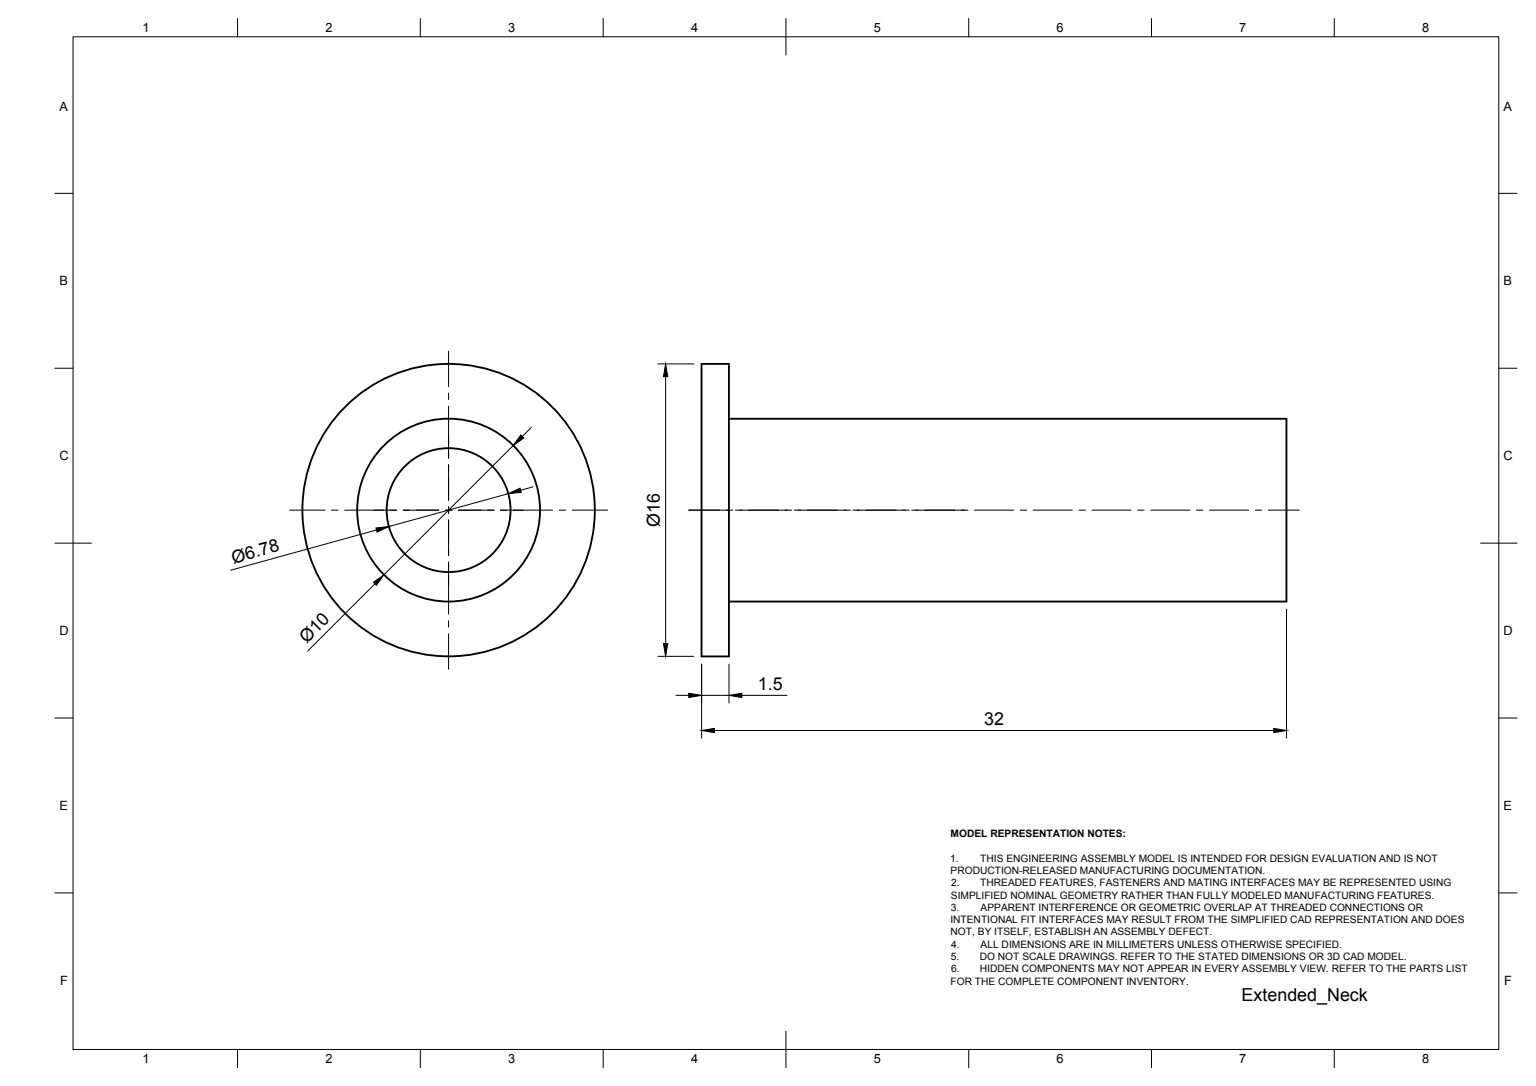
ISO-10303-21;
HEADER;
/* Generated by software containing ST-Developer
 * from STEP Tools, Inc. (www.steptools.com) 
 */

FILE_DESCRIPTION(
/* description */ (''),
/* implementation_level */ '2;1');

FILE_NAME(
/* name */ 'Extended_Neck.step',
/* time_stamp */ '2026-10-06T12:52:28-07:00',
/* author */ (''),
/* organization */ (''),
/* preprocessor_version */ 'ST-DEVELOPER v20.2',
/* originating_system */ 'Autodesk Translation Framework v15.15.0.0',
/* authorisation */ '');

FILE_SCHEMA (('AUTOMOTIVE_DESIGN { 1 0 10303 214 3 1 1 }'));
ENDSEC;

DATA;
#10=MECHANICAL_DESIGN_GEOMETRIC_PRESENTATION_REPRESENTATION('',(#76),#34403);
#45=B_SPLINE_SURFACE_WITH_KNOTS('',3,3,((#12810,#12811,#12812,#12813,#12814,
#12815,#12816,#12817,#12818,#12819,#12820,#12821,#12822,#12823,#12824,#12825,
#12826,#12827,#12828,#12829,#12830,#12831,#12832,#12833,#12834,#12835,#12836,
#12837,#12838,#12839,#12840,#12841,#12842,#12843,#12844,#12845,#12846,#12847,
#12848,#12849,#12850,#12851,#12852,#12853,#12854,#12855,#12856,#12857,#12858,
#12859,#12860,#12861,#12862,#12863,#12864,#12865),(#12866,#12867,#12868,
#12869,#12870,#12871,#12872,#12873,#12874,#12875,#12876,#12877,#12878,#12879,
#12880,#12881,#12882,#12883,#12884,#12885,#12886,#12887,#12888,#12889,#12890,
#12891,#12892,#12893,#12894,#12895,#12896,#12897,#12898,#12899,#12900,#12901,
#12902,#12903,#12904,#12905,#12906,#12907,#12908,#12909,#12910,#12911,#12912,
#12913,#12914,#12915,#12916,#12917,#12918,#12919,#12920,#12921),(#12922,
#12923,#12924,#12925,#12926,#12927,#12928,#12929,#12930,#12931,#12932,#12933,
#12934,#12935,#12936,#12937,#12938,#12939,#12940,#12941,#12942,#12943,#12944,
#12945,#12946,#12947,#12948,#12949,#12950,#12951,#12952,#12953,#12954,#12955,
#12956,#12957,#12958,#12959,#12960,#12961,#12962,#12963,#12964,#12965,#12966,
#12967,#12968,#12969,#12970,#12971,#12972,#12973,#12974,#12975,#12976,#12977),
(#12978,#12979,#12980,#12981,#12982,#12983,#12984,#12985,#12986,#12987,
#12988,#12989,#12990,#12991,#12992,#12993,#12994,#12995,#12996,#12997,#12998,
#12999,#13000,#13001,#13002,#13003,#13004,#13005,#13006,#13007,#13008,#13009,
#13010,#13011,#13012,#13013,#13014,#13015,#13016,#13017,#13018,#13019,#13020,
#13021,#13022,#13023,#13024,#13025,#13026,#13027,#13028,#13029,#13030,#13031,
#13032,#13033)),.UNSPECIFIED.,.F.,.F.,.F.,(4,4),(4,1,1,1,1,1,1,1,1,1,1,
1,1,1,1,1,1,1,1,1,1,1,1,1,1,1,1,1,1,1,1,1,1,1,1,1,1,1,1,1,1,1,1,1,1,1,1,
1,1,1,1,1,1,4),(-0.00052867975577478,0.0806738746488675),(15.627449007124,
16.6139235895809,17.6003981720377,18.5868727544945,19.5733473369513,20.5598219194081,
21.5462965018649,22.5327710843217,23.5192456667785,24.5057202492353,25.4921948316921,
26.4786694141489,27.4651439966058,28.4516185790626,29.4380931615194,30.4245677439762,
31.411042326433,32.3975169088898,33.3839914913466,34.3704660738034,35.3569406562602,
36.343415238717,37.3298898211739,38.3163644036307,39.3028389860875,40.2893135685443,
41.2757881510011,42.2622627334579,43.2487373159147,44.2352118983715,45.2216864808283,
46.2081610632851,47.1946356457419,48.1811102281988,49.1675848106556,50.1540593931124,
51.1405339755692,52.127008558026,53.1134831404828,54.0999577229396,55.0864323053964,
56.0729068878532,57.05938147031,58.0458560527669,59.0323306352237,60.0188052176805,
61.0052798001373,61.9917543825941,62.9782289650509,63.9647035475077,64.9511781299645,
65.9376527124213,66.9241272948781,67.9106018773349),.UNSPECIFIED.);
#46=B_SPLINE_SURFACE_WITH_KNOTS('',3,3,((#13314,#13315,#13316,#13317,#13318,
#13319,#13320,#13321,#13322,#13323,#13324,#13325,#13326,#13327,#13328,#13329,
#13330,#13331,#13332,#13333,#13334,#13335,#13336,#13337,#13338,#13339,#13340,
#13341,#13342,#13343,#13344,#13345,#13346,#13347,#13348,#13349,#13350,#13351,
#13352,#13353,#13354,#13355,#13356,#13357,#13358,#13359,#13360,#13361,#13362,
#13363,#13364,#13365,#13366,#13367,#13368,#13369),(#13370,#13371,#13372,
#13373,#13374,#13375,#13376,#13377,#13378,#13379,#13380,#13381,#13382,#13383,
#13384,#13385,#13386,#13387,#13388,#13389,#13390,#13391,#13392,#13393,#13394,
#13395,#13396,#13397,#13398,#13399,#13400,#13401,#13402,#13403,#13404,#13405,
#13406,#13407,#13408,#13409,#13410,#13411,#13412,#13413,#13414,#13415,#13416,
#13417,#13418,#13419,#13420,#13421,#13422,#13423,#13424,#13425),(#13426,
#13427,#13428,#13429,#13430,#13431,#13432,#13433,#13434,#13435,#13436,#13437,
#13438,#13439,#13440,#13441,#13442,#13443,#13444,#13445,#13446,#13447,#13448,
#13449,#13450,#13451,#13452,#13453,#13454,#13455,#13456,#13457,#13458,#13459,
#13460,#13461,#13462,#13463,#13464,#13465,#13466,#13467,#13468,#13469,#13470,
#13471,#13472,#13473,#13474,#13475,#13476,#13477,#13478,#13479,#13480,#13481),
(#13482,#13483,#13484,#13485,#13486,#13487,#13488,#13489,#13490,#13491,
#13492,#13493,#13494,#13495,#13496,#13497,#13498,#13499,#13500,#13501,#13502,
#13503,#13504,#13505,#13506,#13507,#13508,#13509,#13510,#13511,#13512,#13513,
#13514,#13515,#13516,#13517,#13518,#13519,#13520,#13521,#13522,#13523,#13524,
#13525,#13526,#13527,#13528,#13529,#13530,#13531,#13532,#13533,#13534,#13535,
#13536,#13537)),.UNSPECIFIED.,.F.,.F.,.F.,(4,4),(4,1,1,1,1,1,1,1,1,1,1,
1,1,1,1,1,1,1,1,1,1,1,1,1,1,1,1,1,1,1,1,1,1,1,1,1,1,1,1,1,1,1,1,1,1,1,1,
1,1,1,1,1,1,4),(-0.000393360025247636,0.0809589398657946),(18.1690368310252,
19.155511413482,20.1419859959388,21.1284605783956,22.1149351608524,23.1014097433092,
24.087884325766,25.0743589082228,26.0608334906796,27.0473080731364,28.0337826555933,
29.0202572380501,30.0067318205069,30.9932064029637,31.9796809854205,32.9661555678773,
33.9526301503341,34.9391047327909,35.9255793152477,36.9120538977045,37.8985284801614,
38.8850030626182,39.871477645075,40.8579522275318,41.8444268099886,42.8309013924454,
43.8173759749022,44.803850557359,45.7903251398158,46.7767997222726,47.7632743047295,
48.7497488871863,49.7362234696431,50.7226980520999,51.7091726345567,52.6956472170135,
53.6821217994703,54.6685963819271,55.6550709643839,56.6415455468407,57.6280201292976,
58.6144947117544,59.6009692942112,60.587443876668,61.5739184591248,62.5603930415816,
63.5468676240384,64.5333422064952,65.519816788952,66.5062913714088,67.4927659538656,
68.4792405363225,69.4657151187793,70.452868086171),.UNSPECIFIED.);
#60=SHAPE_REPRESENTATION_RELATIONSHIP('SRR','None',#34438,#68);
#68=ADVANCED_BREP_SHAPE_REPRESENTATION('',(#84),#34398);
#76=STYLED_ITEM('',(#34484),#84);
#84=MANIFOLD_SOLID_BREP('Body1',#4385);
#97=FACE_BOUND('',#795,.T.);
#98=FACE_BOUND('',#797,.T.);
#99=FACE_BOUND('',#800,.T.);
#131=PLANE('',#4547);
#132=PLANE('',#4551);
#133=PLANE('',#4553);
#134=PLANE('',#4556);
#182=CIRCLE('',#4524,4.085);
#183=CIRCLE('',#4532,4.085);
#184=CIRCLE('',#4534,3.38975);
#185=CIRCLE('',#4542,3.38975);
#186=CIRCLE('',#4543,3.38975);
#187=CIRCLE('',#4544,3.38975);
#188=CIRCLE('',#4549,8.);
#189=CIRCLE('',#4550,8.);
#190=CIRCLE('',#4552,5.);
#191=CIRCLE('',#4554,5.);
#533=FACE_OUTER_BOUND('',#772,.T.);
#534=FACE_OUTER_BOUND('',#773,.T.);
#535=FACE_OUTER_BOUND('',#774,.T.);
#536=FACE_OUTER_BOUND('',#775,.T.);
#537=FACE_OUTER_BOUND('',#776,.T.);
#538=FACE_OUTER_BOUND('',#777,.T.);
#539=FACE_OUTER_BOUND('',#778,.T.);
#540=FACE_OUTER_BOUND('',#779,.T.);
#541=FACE_OUTER_BOUND('',#780,.T.);
#542=FACE_OUTER_BOUND('',#781,.T.);
#543=FACE_OUTER_BOUND('',#782,.T.);
#544=FACE_OUTER_BOUND('',#783,.T.);
#545=FACE_OUTER_BOUND('',#784,.T.);
#546=FACE_OUTER_BOUND('',#785,.T.);
#547=FACE_OUTER_BOUND('',#786,.T.);
#548=FACE_OUTER_BOUND('',#787,.T.);
#549=FACE_OUTER_BOUND('',#788,.T.);
#550=FACE_OUTER_BOUND('',#789,.T.);
#551=FACE_OUTER_BOUND('',#790,.T.);
#552=FACE_OUTER_BOUND('',#791,.T.);
#553=FACE_OUTER_BOUND('',#792,.T.);
#554=FACE_OUTER_BOUND('',#793,.T.);
#555=FACE_OUTER_BOUND('',#794,.T.);
#556=FACE_OUTER_BOUND('',#796,.T.);
#557=FACE_OUTER_BOUND('',#798,.T.);
#558=FACE_OUTER_BOUND('',#799,.T.);
#772=EDGE_LOOP('',(#2757,#2758,#2759,#2760));
#773=EDGE_LOOP('',(#2761,#2762,#2763,#2764,#2765,#2766));
#774=EDGE_LOOP('',(#2767,#2768,#2769,#2770,#2771,#2772));
#775=EDGE_LOOP('',(#2773,#2774,#2775,#2776,#2777,#2778));
#776=EDGE_LOOP('',(#2779,#2780,#2781,#2782,#2783,#2784));
#777=EDGE_LOOP('',(#2785,#2786,#2787,#2788,#2789,#2790));
#778=EDGE_LOOP('',(#2791,#2792,#2793,#2794,#2795,#2796));
#779=EDGE_LOOP('',(#2797,#2798,#2799,#2800,#2801,#2802));
#780=EDGE_LOOP('',(#2803,#2804,#2805,#2806,#2807,#2808));
#781=EDGE_LOOP('',(#2809,#2810,#2811,#2812,#2813,#2814));
#782=EDGE_LOOP('',(#2815,#2816,#2817,#2818,#2819,#2820));
#783=EDGE_LOOP('',(#2821,#2822,#2823,#2824,#2825));
#784=EDGE_LOOP('',(#2826,#2827,#2828,#2829,#2830,#2831));
#785=EDGE_LOOP('',(#2832,#2833,#2834,#2835,#2836));
#786=EDGE_LOOP('',(#2837,#2838,#2839,#2840,#2841,#2842));
#787=EDGE_LOOP('',(#2843,#2844,#2845,#2846,#2847,#2848,#2849,#2850));
#788=EDGE_LOOP('',(#2851,#2852,#2853,#2854,#2855));
#789=EDGE_LOOP('',(#2856,#2857,#2858,#2859,#2860,#2861));
#790=EDGE_LOOP('',(#2862,#2863,#2864,#2865,#2866,#2867,#2868,#2869,#2870,
#2871,#2872,#2873,#2874,#2875,#2876,#2877,#2878,#2879,#2880,#2881,#2882,
#2883,#2884,#2885,#2886,#2887,#2888,#2889,#2890,#2891,#2892,#2893,#2894,
#2895,#2896,#2897));
#791=EDGE_LOOP('',(#2898,#2899,#2900,#2901,#2902));
#792=EDGE_LOOP('',(#2903,#2904,#2905,#2906,#2907,#2908,#2909,#2910,#2911,
#2912,#2913,#2914,#2915,#2916,#2917,#2918,#2919,#2920,#2921,#2922,#2923,
#2924,#2925,#2926,#2927,#2928,#2929,#2930,#2931,#2932,#2933,#2934,#2935));
#793=EDGE_LOOP('',(#2936,#2937,#2938,#2939));
#794=EDGE_LOOP('',(#2940));
#795=EDGE_LOOP('',(#2941));
#796=EDGE_LOOP('',(#2942));
#797=EDGE_LOOP('',(#2943));
#798=EDGE_LOOP('',(#2944,#2945,#2946,#2947));
#799=EDGE_LOOP('',(#2948));
#800=EDGE_LOOP('',(#2949,#2950,#2951,#2952));
#1021=LINE('',#6412,#1158);
#1022=LINE('',#6478,#1159);
#1023=LINE('',#6912,#1160);
#1024=LINE('',#7381,#1161);
#1025=LINE('',#7847,#1162);
#1026=LINE('',#8319,#1163);
#1027=LINE('',#8782,#1164);
#1028=LINE('',#9248,#1165);
#1029=LINE('',#9489,#1166);
#1030=LINE('',#9865,#1167);
#1031=LINE('',#10100,#1168);
#1032=LINE('',#10536,#1169);
#1033=LINE('',#10928,#1170);
#1034=LINE('',#11325,#1171);
#1035=LINE('',#11705,#1172);
#1036=LINE('',#11896,#1173);
#1037=LINE('',#11943,#1174);
#1038=LINE('',#13633,#1175);
#1039=LINE('',#13642,#1176);
#1158=VECTOR('',#5100,4.085);
#1159=VECTOR('',#5105,4.085);
#1160=VECTOR('',#5108,4.085);
#1161=VECTOR('',#5111,4.085);
#1162=VECTOR('',#5114,4.085);
#1163=VECTOR('',#5117,4.085);
#1164=VECTOR('',#5120,4.085);
#1165=VECTOR('',#5123,4.085);
#1166=VECTOR('',#5128,3.38975);
#1167=VECTOR('',#5133,3.38975);
#1168=VECTOR('',#5136,3.38975);
#1169=VECTOR('',#5139,3.38975);
#1170=VECTOR('',#5142,3.38975);
#1171=VECTOR('',#5145,3.38975);
#1172=VECTOR('',#5148,3.38975);
#1173=VECTOR('',#5153,3.38975);
#1174=VECTOR('',#5156,3.38975);
#1175=VECTOR('',#5169,8.);
#1176=VECTOR('',#5182,5.);
#1296=B_SPLINE_CURVE_WITH_KNOTS('',3,(#6414,#6415,#6416,#6417),
 .UNSPECIFIED.,.F.,.F.,(4,4),(66.9422038205255,67.9106018773349),
 .UNSPECIFIED.);
#1297=B_SPLINE_CURVE_WITH_KNOTS('',3,(#6420,#6421,#6422,#6423,#6424,#6425,
#6426,#6427,#6428,#6429,#6430,#6431,#6432,#6433,#6434,#6435,#6436,#6437,
#6438,#6439,#6440,#6441,#6442,#6443,#6444,#6445,#6446,#6447,#6448,#6449,
#6450,#6451,#6452,#6453,#6454,#6455,#6456,#6457,#6458,#6459,#6460,#6461,
#6462,#6463,#6464,#6465,#6466,#6467,#6468,#6469,#6470,#6471,#6472,#6473,
#6474),.UNSPECIFIED.,.F.,.F.,(4,3,3,3,3,3,3,3,3,3,3,3,3,3,3,3,3,3,4),(66.9424261296312,
67.0301287110664,67.11783680989,67.2055708646774,67.2933977991414,67.3812798406369,
67.4692836569234,67.4927659538656,67.5800588691701,67.6672436830704,67.7543439714456,
67.8413856927823,67.9283969745756,68.0153990026826,68.1024129513622,68.1895118069197,
68.276654508908,68.3639316760445,68.4345182397239),.UNSPECIFIED.);
#1298=B_SPLINE_CURVE_WITH_KNOTS('',3,(#6480,#6481,#6482,#6483,#6484,#6485,
#6486,#6487,#6488,#6489,#6490,#6491,#6492,#6493,#6494,#6495,#6496,#6497,
#6498,#6499,#6500,#6501,#6502,#6503,#6504,#6505,#6506,#6507,#6508,#6509,
#6510,#6511,#6512,#6513,#6514,#6515,#6516,#6517,#6518,#6519,#6520,#6521,
#6522,#6523,#6524,#6525,#6526,#6527,#6528,#6529,#6530,#6531,#6532,#6533,
#6534,#6535,#6536,#6537,#6538,#6539,#6540,#6541,#6542,#6543,#6544,#6545,
#6546,#6547,#6548,#6549,#6550,#6551,#6552,#6553,#6554,#6555,#6556,#6557,
#6558,#6559,#6560,#6561,#6562,#6563,#6564,#6565,#6566,#6567,#6568,#6569,
#6570,#6571,#6572,#6573,#6574,#6575,#6576,#6577,#6578,#6579,#6580,#6581,
#6582,#6583,#6584,#6585,#6586,#6587,#6588,#6589,#6590,#6591,#6592,#6593,
#6594,#6595,#6596,#6597,#6598,#6599,#6600,#6601,#6602,#6603,#6604,#6605,
#6606,#6607,#6608,#6609,#6610,#6611,#6612,#6613,#6614,#6615,#6616,#6617,
#6618,#6619,#6620,#6621,#6622,#6623,#6624,#6625,#6626,#6627,#6628,#6629,
#6630,#6631,#6632,#6633,#6634,#6635,#6636,#6637,#6638,#6639,#6640,#6641,
#6642,#6643,#6644,#6645,#6646,#6647,#6648,#6649,#6650,#6651,#6652,#6653,
#6654,#6655,#6656,#6657,#6658,#6659,#6660,#6661,#6662,#6663,#6664,#6665,
#6666,#6667,#6668,#6669,#6670,#6671,#6672,#6673,#6674,#6675),
 .UNSPECIFIED.,.F.,.F.,(4,3,3,3,3,3,3,3,3,3,3,3,3,3,3,3,3,3,3,3,3,3,3,3,
3,3,3,3,3,3,3,3,3,3,3,3,3,3,3,3,3,3,3,3,3,3,3,3,3,3,3,3,3,3,3,3,3,3,3,3,
3,3,3,3,3,4),(60.65863305798,60.7462805898925,60.8339724069765,60.9218056826776,
61.0052798001373,61.0931588658759,61.1809279562765,61.268609989713,61.3590030388232,
61.4465878063973,61.5341599134385,61.6217399433751,61.7093484801914,61.7970529682031,
61.8848150467633,61.9727002613834,61.9917543825941,62.0796342468088,62.1674043958499,
62.2550877431606,62.3454803958969,62.4330670954196,62.5206413585054,62.6082237650501,
62.6958348956645,62.783542281868,62.8713074397826,62.9591959709118,62.9782289650509,
63.0659959514938,63.1536528050209,63.2412225781541,63.3316576993233,63.4191308553117,
63.5065917826189,63.5940611841444,63.6815597638258,63.7691558290588,63.8568102574783,
63.944589744661,63.9647035475077,64.052716452029,64.1406191116994,64.2284342850664,
64.3187772656787,64.406493254731,64.4941956385468,64.581904856344,64.6742231747492,
64.7620556467768,64.8499453709517,64.9379542944654,64.9511781299645,65.039109056126,
65.1269316198708,65.2146686503736,65.3050416581296,65.3926847974272,65.4803164125707,
65.5679570124934,65.6556271074234,65.743394281365,65.8312197741986,65.9191689688196,
65.9376527124213,65.9734457253856),.UNSPECIFIED.);
#1299=B_SPLINE_CURVE_WITH_KNOTS('',3,(#6676,#6677,#6678,#6679,#6680),
 .UNSPECIFIED.,.F.,.F.,(4,1,4),(65.9734517999329,66.9241272948781,66.9422038205255),
 .UNSPECIFIED.);
#1300=B_SPLINE_CURVE_WITH_KNOTS('',3,(#6682,#6683,#6684,#6685,#6686,#6687,
#6688,#6689,#6690,#6691,#6692,#6693,#6694,#6695,#6696,#6697,#6698,#6699,
#6700,#6701,#6702,#6703,#6704,#6705,#6706,#6707,#6708,#6709,#6710,#6711,
#6712,#6713,#6714,#6715),.UNSPECIFIED.,.F.,.F.,(4,3,3,3,3,3,3,3,3,3,3,4),
(65.9734457253856,66.0635791722207,66.1537859784836,66.2441584095279,66.3346160682269,
66.4252650574005,66.5062913714088,66.5943110699188,66.6821978307666,66.7700074190229,
66.8577576382145,66.9424261296312),.UNSPECIFIED.);
#1301=B_SPLINE_CURVE_WITH_KNOTS('',3,(#6716,#6717,#6718,#6719,#6720,#6721,
#6722,#6723,#6724,#6725,#6726,#6727,#6728,#6729,#6730,#6731,#6732,#6733,
#6734,#6735,#6736,#6737,#6738,#6739,#6740,#6741,#6742,#6743,#6744,#6745,
#6746,#6747,#6748,#6749,#6750,#6751,#6752,#6753,#6754,#6755,#6756,#6757,
#6758,#6759,#6760,#6761,#6762,#6763,#6764,#6765,#6766,#6767,#6768,#6769,
#6770,#6771,#6772,#6773,#6774,#6775,#6776,#6777,#6778,#6779,#6780,#6781,
#6782,#6783,#6784,#6785,#6786,#6787,#6788,#6789,#6790,#6791,#6792,#6793,
#6794,#6795,#6796,#6797,#6798,#6799,#6800,#6801,#6802,#6803,#6804,#6805,
#6806,#6807,#6808,#6809,#6810,#6811,#6812,#6813,#6814,#6815,#6816,#6817,
#6818,#6819,#6820,#6821,#6822,#6823,#6824,#6825,#6826,#6827,#6828,#6829,
#6830,#6831,#6832,#6833,#6834,#6835,#6836,#6837,#6838,#6839,#6840,#6841,
#6842,#6843,#6844,#6845,#6846,#6847,#6848,#6849,#6850,#6851,#6852,#6853,
#6854,#6855,#6856,#6857,#6858,#6859,#6860,#6861,#6862,#6863,#6864,#6865,
#6866,#6867,#6868,#6869,#6870,#6871,#6872,#6873,#6874,#6875,#6876,#6877,
#6878,#6879,#6880,#6881,#6882,#6883,#6884,#6885,#6886,#6887,#6888,#6889,
#6890,#6891,#6892,#6893,#6894,#6895,#6896,#6897,#6898,#6899,#6900,#6901,
#6902,#6903,#6904,#6905,#6906,#6907,#6908),.UNSPECIFIED.,.F.,.F.,(4,3,3,
3,3,3,3,3,3,3,3,3,3,3,3,3,3,3,3,3,3,3,3,3,3,3,3,3,3,3,3,3,3,3,3,3,3,3,3,
3,3,3,3,3,3,3,3,3,3,3,3,3,3,3,3,3,3,3,3,3,3,3,3,3,4),(60.6593693718721,
60.7471428095145,60.8348250979655,60.922439102879,61.0100156253259,61.0975752044484,
61.1851384398607,61.2727259287143,61.3604075726339,61.4481429995207,61.5360068051033,
61.5739184591248,61.6617852019871,61.7495420513973,61.8372119392129,61.927609577009,
62.015182510545,62.1027429191062,62.1903113984739,62.2779085450996,62.3656019348734,
62.4533530734372,62.541227657696,62.5603930415816,62.6482441716657,62.7359853638815,
62.8236395693427,62.9140430761797,63.001600365264,63.0891451707661,63.1766981055555,
63.2642797832255,63.3519578926021,63.439693843782,63.5275534886173,63.5468676240384,
63.634746673192,63.722515747168,63.810197764357,63.9005908196243,63.9881755714853,
64.0757476630367,64.1633276777229,64.2509361995434,64.3386406730057,64.4264027372613,
64.5142879380342,64.5333422064952,64.621221995123,64.7089920681593,64.7966753391438,
64.8870680203698,64.9746546432615,65.0622288297388,65.1498111597819,65.2374222140876,
65.3251295246472,65.4128946072222,65.5007830640145,65.519816788952,65.6138059465638,
65.707511444738,65.8010451097038,65.8943210633096,65.9734457251906),
 .UNSPECIFIED.);
#1302=B_SPLINE_CURVE_WITH_KNOTS('',3,(#6914,#6915,#6916,#6917,#6918,#6919,
#6920,#6921,#6922,#6923,#6924,#6925,#6926,#6927,#6928,#6929,#6930,#6931,
#6932,#6933,#6934,#6935,#6936,#6937,#6938,#6939,#6940,#6941,#6942,#6943,
#6944,#6945,#6946,#6947,#6948,#6949,#6950,#6951,#6952,#6953,#6954,#6955,
#6956,#6957,#6958,#6959,#6960,#6961,#6962,#6963,#6964,#6965,#6966,#6967,
#6968,#6969,#6970,#6971,#6972,#6973,#6974,#6975,#6976,#6977,#6978,#6979,
#6980,#6981,#6982,#6983,#6984,#6985,#6986,#6987,#6988,#6989,#6990,#6991,
#6992,#6993,#6994,#6995,#6996,#6997,#6998,#6999,#7000,#7001,#7002,#7003,
#7004,#7005,#7006,#7007,#7008,#7009,#7010,#7011,#7012,#7013,#7014,#7015,
#7016,#7017,#7018,#7019,#7020,#7021,#7022,#7023,#7024,#7025,#7026,#7027,
#7028,#7029,#7030,#7031,#7032,#7033,#7034,#7035,#7036,#7037,#7038,#7039,
#7040,#7041,#7042,#7043,#7044,#7045,#7046,#7047,#7048,#7049,#7050,#7051,
#7052,#7053,#7054,#7055,#7056,#7057,#7058,#7059,#7060,#7061,#7062,#7063,
#7064,#7065,#7066,#7067,#7068,#7069,#7070,#7071,#7072,#7073,#7074,#7075,
#7076,#7077,#7078,#7079,#7080,#7081,#7082,#7083,#7084,#7085,#7086,#7087,
#7088,#7089,#7090,#7091,#7092,#7093,#7094,#7095,#7096,#7097,#7098,#7099,
#7100,#7101,#7102,#7103,#7104,#7105,#7106),.UNSPECIFIED.,.F.,.F.,(4,3,3,
3,3,3,3,3,3,3,3,3,3,3,3,3,3,3,3,3,3,3,3,3,3,3,3,3,3,3,3,3,3,3,3,3,3,3,3,
3,3,3,3,3,3,3,3,3,3,3,3,3,3,3,3,3,3,3,3,3,3,3,3,3,4),(54.3763646710769,
54.4651231253668,54.5526899009801,54.6402468478357,54.7278145647135,54.8174689998842,
54.9051667757655,54.9957995405809,55.0864323053964,55.1742960896468,55.2620499541187,
55.3497168345997,55.4401155912564,55.5276854816214,55.615242839173,55.7028082631215,
55.7904023533463,55.8780927007007,55.9658408016046,56.0537123778884,56.0729068878532,
56.1607710647536,56.2485253261876,56.3361926074087,56.4265912152714,56.5141615131015,
56.6017192798774,56.689285114346,56.7768796159245,56.864570373776,56.952318885137,
57.0401908687341,57.05938147031,57.1472435605767,57.2349957310401,57.3226609195071,
57.4130603111646,57.5006285251765,57.5881842150842,57.6757479819056,57.7633404273363,
57.851029156223,57.9387756522291,58.02664565519,58.0458560527669,58.1337211732737,
58.2214763663591,58.3091445663341,58.3995428249453,58.4871140040178,58.5746726366804,
58.6622393207953,58.7498346548823,58.8375262159865,58.9252755144032,59.0131482558552,
59.0323306352237,59.1201349616358,59.2078320873874,59.2954427965408,59.3829878029622,
59.4704935028068,59.5579758209044,59.6454743488502,59.6902604182061),
 .UNSPECIFIED.);
#1303=B_SPLINE_CURVE_WITH_KNOTS('',3,(#7107,#7108,#7109,#7110,#7111,#7112,
#7113,#7114,#7115,#7116,#7117,#7118,#7119,#7120,#7121,#7122,#7123,#7124,
#7125,#7126,#7127,#7128,#7129,#7130,#7131,#7132,#7133,#7134,#7135,#7136,
#7137,#7138,#7139,#7140,#7141,#7142,#7143),.UNSPECIFIED.,.F.,.F.,(4,3,3,
3,3,3,3,3,3,3,3,3,4),(59.6902604184005,59.7919143931213,59.8941560797584,
59.9970488126565,60.0188052176805,60.1066415554168,60.194374903753,60.2820260480705,
60.3696157068656,60.4571706432182,60.544705998586,60.632257830546,60.65863305798),
 .UNSPECIFIED.);
#1304=B_SPLINE_CURVE_WITH_KNOTS('',3,(#7145,#7146,#7147,#7148,#7149,#7150,
#7151,#7152,#7153,#7154,#7155,#7156,#7157,#7158,#7159,#7160,#7161,#7162,
#7163,#7164,#7165,#7166,#7167,#7168,#7169,#7170,#7171,#7172,#7173,#7174,
#7175,#7176,#7177,#7178,#7179,#7180,#7181),.UNSPECIFIED.,.F.,.F.,(4,3,3,
3,3,3,3,3,3,3,3,3,4),(59.69026041841,59.7770684744581,59.8637759910736,
59.9542344767729,60.0408167469363,60.1273775252551,60.2139383758267,60.3005208587838,
60.3871935732878,60.4739195335137,60.5607688817594,60.587443876668,60.6593693718721),
 .UNSPECIFIED.);
#1305=B_SPLINE_CURVE_WITH_KNOTS('',3,(#7182,#7183,#7184,#7185,#7186,#7187,
#7188,#7189,#7190,#7191,#7192,#7193,#7194,#7195,#7196,#7197,#7198,#7199,
#7200,#7201,#7202,#7203,#7204,#7205,#7206,#7207,#7208,#7209,#7210,#7211,
#7212,#7213,#7214,#7215,#7216,#7217,#7218,#7219,#7220,#7221,#7222,#7223,
#7224,#7225,#7226,#7227,#7228,#7229,#7230,#7231,#7232,#7233,#7234,#7235,
#7236,#7237,#7238,#7239,#7240,#7241,#7242,#7243,#7244,#7245,#7246,#7247,
#7248,#7249,#7250,#7251,#7252,#7253,#7254,#7255,#7256,#7257,#7258,#7259,
#7260,#7261,#7262,#7263,#7264,#7265,#7266,#7267,#7268,#7269,#7270,#7271,
#7272,#7273,#7274,#7275,#7276,#7277,#7278,#7279,#7280,#7281,#7282,#7283,
#7284,#7285,#7286,#7287,#7288,#7289,#7290,#7291,#7292,#7293,#7294,#7295,
#7296,#7297,#7298,#7299,#7300,#7301,#7302,#7303,#7304,#7305,#7306,#7307,
#7308,#7309,#7310,#7311,#7312,#7313,#7314,#7315,#7316,#7317,#7318,#7319,
#7320,#7321,#7322,#7323,#7324,#7325,#7326,#7327,#7328,#7329,#7330,#7331,
#7332,#7333,#7334,#7335,#7336,#7337,#7338,#7339,#7340,#7341,#7342,#7343,
#7344,#7345,#7346,#7347,#7348,#7349,#7350,#7351,#7352,#7353,#7354,#7355,
#7356,#7357,#7358,#7359,#7360,#7361,#7362,#7363,#7364,#7365,#7366,#7367,
#7368,#7369,#7370,#7371,#7372,#7373,#7374,#7375,#7376,#7377),
 .UNSPECIFIED.,.F.,.F.,(4,3,3,3,3,3,3,3,3,3,3,3,3,3,3,3,3,3,3,3,3,3,3,3,
3,3,3,3,3,3,3,3,3,3,3,3,3,3,3,3,3,3,3,3,3,3,3,3,3,3,3,3,3,3,3,3,3,3,3,3,
3,3,3,3,3,4),(54.3753548645582,54.4630392923091,54.5507792046392,54.6386454074467,
54.6685963819271,54.7564600562574,54.8442138119439,54.9318805848875,55.0222793823246,
55.1098491689013,55.1974064242269,55.2849717476172,55.3725657390588,55.4602559907231,
55.5480039976374,55.6358754830825,55.6550709643839,55.7429347095602,55.8306885366184,
55.9183553813669,56.0087541520512,56.0963240110393,56.1838813388722,56.2714467347849,
56.3590407986829,56.4467311223415,56.5344792010609,56.6223507574992,56.6415455468407,
56.7294090248321,56.8171625843396,56.9048291614957,56.995228032471,57.0827976254673,
57.170354688365,57.257919820688,57.3455136226315,57.433203688048,57.5209515104051,
57.6088228151113,57.6280201292976,57.7158839134109,57.8036377777518,57.8913046581076,
57.9817034148135,58.069273305069,58.1568306625171,58.2443960863681,58.3319901765016,
58.4196805237739,58.5074286246011,58.5953002008165,58.6144947117544,58.7023588861019,
58.7901131449712,58.8777804236191,58.9681790324431,59.0557493276956,59.1433070918966,
59.2308729237961,59.3184674228137,59.4061581781297,59.4939066869673,59.5817786680768,
59.6009692942112,59.6902604182061),.UNSPECIFIED.);
#1306=B_SPLINE_CURVE_WITH_KNOTS('',3,(#7383,#7384,#7385,#7386,#7387,#7388,
#7389,#7390,#7391,#7392,#7393,#7394,#7395,#7396,#7397,#7398,#7399,#7400,
#7401,#7402,#7403,#7404,#7405,#7406,#7407,#7408,#7409,#7410,#7411,#7412,
#7413,#7414,#7415,#7416,#7417,#7418,#7419,#7420,#7421,#7422,#7423,#7424,
#7425,#7426,#7427,#7428,#7429,#7430,#7431,#7432,#7433,#7434,#7435,#7436,
#7437,#7438,#7439,#7440,#7441,#7442,#7443,#7444,#7445,#7446,#7447,#7448,
#7449,#7450,#7451,#7452,#7453,#7454,#7455,#7456,#7457,#7458,#7459,#7460,
#7461,#7462,#7463,#7464,#7465,#7466,#7467,#7468,#7469,#7470,#7471,#7472,
#7473,#7474,#7475,#7476,#7477,#7478,#7479,#7480,#7481,#7482,#7483,#7484,
#7485,#7486,#7487,#7488,#7489,#7490,#7491,#7492,#7493,#7494,#7495,#7496,
#7497,#7498,#7499,#7500,#7501,#7502,#7503,#7504,#7505,#7506,#7507,#7508,
#7509,#7510,#7511,#7512,#7513,#7514,#7515,#7516,#7517,#7518,#7519,#7520,
#7521,#7522,#7523,#7524,#7525,#7526,#7527,#7528,#7529,#7530,#7531,#7532,
#7533,#7534,#7535,#7536,#7537,#7538,#7539,#7540,#7541,#7542,#7543,#7544,
#7545,#7546,#7547,#7548,#7549,#7550,#7551,#7552,#7553,#7554,#7555,#7556,
#7557,#7558,#7559,#7560,#7561,#7562,#7563,#7564,#7565,#7566,#7567,#7568,
#7569,#7570,#7571,#7572,#7573,#7574,#7575),.UNSPECIFIED.,.F.,.F.,(4,3,3,
3,3,3,3,3,3,3,3,3,3,3,3,3,3,3,3,3,3,3,3,3,3,3,3,3,3,3,3,3,3,3,3,3,3,3,3,
3,3,3,3,3,3,3,3,3,3,3,3,3,3,3,3,3,3,3,3,3,3,3,3,3,4),(48.0922715957158,
48.1811102281988,48.2689738944005,48.356727642146,48.4443944073429,48.534793207757,
48.6223629871136,48.7099202354255,48.7974855520155,48.8850795368768,48.9727697823158,
49.0605177832053,49.1483892629593,49.1675848106556,49.255448478926,49.3432022287112,
49.430868995917,49.5212677955664,49.6088375768429,49.6963948270385,49.7839601454743,
49.8715541321415,49.9592443793189,50.0469923819093,50.1348638632974,50.1540593931124,
50.2419230728153,50.3296768340956,50.4173436128442,50.5077424081848,50.5953122010484,
50.682869462827,50.7704347928287,50.8580287910321,50.9457190496439,51.0334670636219,
51.1213385562451,51.1405339755692,51.2283976218724,51.3161513497307,51.4038180950754,
51.4942169029442,51.5817866626605,51.6693438914446,51.7569091886402,51.8445031542623,
51.9321933807854,52.0199413629268,52.1078128243148,52.127008558026,52.2148722323394,
52.3026259880082,52.3902927609331,52.4806915583768,52.5682613449324,52.6558186002362,
52.743383923604,52.8309779150221,52.9186681666621,53.0064161735513,53.0942876589708,
53.1134831404828,53.2201894401228,53.325638450398,53.4070751108784),
 .UNSPECIFIED.);
#1307=B_SPLINE_CURVE_WITH_KNOTS('',3,(#7576,#7577,#7578,#7579,#7580,#7581,
#7582,#7583,#7584,#7585,#7586,#7587,#7588,#7589,#7590,#7591,#7592,#7593,
#7594,#7595,#7596,#7597,#7598,#7599,#7600,#7601,#7602,#7603,#7604,#7605,
#7606,#7607,#7608,#7609,#7610,#7611,#7612),.UNSPECIFIED.,.F.,.F.,(4,3,3,
3,3,3,3,3,3,3,3,3,4),(53.4070751110265,53.4941360616469,53.5811674224662,
53.668190330731,53.7552259127633,53.8423504842459,53.9295193536601,54.0168313543366,
54.0999577229396,54.18781472203,54.2755749632124,54.3632416699008,54.3763646710769),
 .UNSPECIFIED.);
#1308=B_SPLINE_CURVE_WITH_KNOTS('',3,(#7614,#7615,#7616,#7617,#7618,#7619,
#7620,#7621,#7622,#7623,#7624,#7625,#7626,#7627,#7628,#7629,#7630,#7631,
#7632,#7633,#7634,#7635,#7636,#7637,#7638,#7639,#7640,#7641,#7642,#7643,
#7644,#7645,#7646,#7647),.UNSPECIFIED.,.F.,.F.,(4,3,3,3,3,3,3,3,3,3,3,4),
(53.4070751112481,53.514566858387,53.6236544087936,53.6821217994703,53.7699662995981,
53.8577089201619,53.9453704283004,54.0329715255116,54.1205451319431,54.2080995546255,
54.2956889402079,54.3753548645582),.UNSPECIFIED.);
#1309=B_SPLINE_CURVE_WITH_KNOTS('',3,(#7648,#7649,#7650,#7651,#7652,#7653,
#7654,#7655,#7656,#7657,#7658,#7659,#7660,#7661,#7662,#7663,#7664,#7665,
#7666,#7667,#7668,#7669,#7670,#7671,#7672,#7673,#7674,#7675,#7676,#7677,
#7678,#7679,#7680,#7681,#7682,#7683,#7684,#7685,#7686,#7687,#7688,#7689,
#7690,#7691,#7692,#7693,#7694,#7695,#7696,#7697,#7698,#7699,#7700,#7701,
#7702,#7703,#7704,#7705,#7706,#7707,#7708,#7709,#7710,#7711,#7712,#7713,
#7714,#7715,#7716,#7717,#7718,#7719,#7720,#7721,#7722,#7723,#7724,#7725,
#7726,#7727,#7728,#7729,#7730,#7731,#7732,#7733,#7734,#7735,#7736,#7737,
#7738,#7739,#7740,#7741,#7742,#7743,#7744,#7745,#7746,#7747,#7748,#7749,
#7750,#7751,#7752,#7753,#7754,#7755,#7756,#7757,#7758,#7759,#7760,#7761,
#7762,#7763,#7764,#7765,#7766,#7767,#7768,#7769,#7770,#7771,#7772,#7773,
#7774,#7775,#7776,#7777,#7778,#7779,#7780,#7781,#7782,#7783,#7784,#7785,
#7786,#7787,#7788,#7789,#7790,#7791,#7792,#7793,#7794,#7795,#7796,#7797,
#7798,#7799,#7800,#7801,#7802,#7803,#7804,#7805,#7806,#7807,#7808,#7809,
#7810,#7811,#7812,#7813,#7814,#7815,#7816,#7817,#7818,#7819,#7820,#7821,
#7822,#7823,#7824,#7825,#7826,#7827,#7828,#7829,#7830,#7831,#7832,#7833,
#7834,#7835,#7836,#7837,#7838,#7839,#7840,#7841,#7842,#7843),
 .UNSPECIFIED.,.F.,.F.,(4,3,3,3,3,3,3,3,3,3,3,3,3,3,3,3,3,3,3,3,3,3,3,3,
3,3,3,3,3,3,3,3,3,3,3,3,3,3,3,3,3,3,3,3,3,3,3,3,3,3,3,3,3,3,3,3,3,3,3,3,
3,3,3,3,3,4),(48.0930924415186,48.1806692098407,48.2682278326461,48.3557889116037,
48.4433730450696,48.5310507770843,48.6187812155429,48.7066414710093,48.7497488871863,
48.8376125557049,48.92536630576,49.0130330732565,49.1034318728048,49.1910016544217,
49.2785589049755,49.3661242237864,49.4537182108454,49.5414084584371,49.6291564614553,
49.7170279432874,49.7362234696431,49.8240871398504,49.9118408916014,49.9995076607984,
50.0899064597111,50.1774762430298,50.2650334952829,50.3525988157889,50.4401928045367,
50.5278830537994,50.6156310584803,50.7035025419507,50.7226980520999,50.8105617183162,
50.8983154660761,50.9859822312877,51.0763810316963,51.1639508110672,51.2515080593933,
51.3390733759977,51.4266673608728,51.5143576063255,51.6021056072286,51.6899770869957,
51.7091726345567,51.7970363028357,51.88479005263,51.9724568198442,52.0628556194904,
52.1504254007761,52.2379826509813,52.3255479694264,52.4131419561032,52.5008322032902,
52.5885802058899,52.6764516872875,52.6956472170135,52.7845757037651,52.8715739991427,
52.9584927489579,53.0453533763273,53.1357838100021,53.222609258072,53.3094383650151,
53.3963131402274,53.4070751110265),.UNSPECIFIED.);
#1310=B_SPLINE_CURVE_WITH_KNOTS('',3,(#7849,#7850,#7851,#7852,#7853,#7854,
#7855,#7856,#7857,#7858,#7859,#7860,#7861,#7862,#7863,#7864,#7865,#7866,
#7867,#7868,#7869,#7870,#7871,#7872,#7873,#7874,#7875,#7876,#7877,#7878,
#7879,#7880,#7881,#7882,#7883,#7884,#7885,#7886,#7887,#7888,#7889,#7890,
#7891,#7892,#7893,#7894,#7895,#7896,#7897,#7898,#7899,#7900,#7901,#7902,
#7903,#7904,#7905,#7906,#7907,#7908,#7909,#7910,#7911,#7912,#7913,#7914,
#7915,#7916,#7917,#7918,#7919,#7920,#7921,#7922,#7923,#7924,#7925,#7926,
#7927,#7928,#7929,#7930,#7931,#7932,#7933,#7934,#7935,#7936,#7937,#7938,
#7939,#7940,#7941,#7942,#7943,#7944,#7945,#7946,#7947,#7948,#7949,#7950,
#7951,#7952,#7953,#7954,#7955,#7956,#7957,#7958,#7959,#7960,#7961,#7962,
#7963,#7964,#7965,#7966,#7967,#7968,#7969,#7970,#7971,#7972,#7973,#7974,
#7975,#7976,#7977,#7978,#7979,#7980,#7981,#7982,#7983,#7984,#7985,#7986,
#7987,#7988,#7989,#7990,#7991,#7992,#7993,#7994,#7995,#7996,#7997,#7998,
#7999,#8000,#8001,#8002,#8003,#8004,#8005,#8006,#8007,#8008,#8009,#8010,
#8011,#8012,#8013,#8014,#8015,#8016,#8017,#8018,#8019,#8020,#8021,#8022,
#8023,#8024,#8025,#8026,#8027,#8028,#8029,#8030,#8031,#8032,#8033,#8034,
#8035,#8036,#8037,#8038,#8039,#8040,#8041,#8042,#8043,#8044),
 .UNSPECIFIED.,.F.,.F.,(4,3,3,3,3,3,3,3,3,3,3,3,3,3,3,3,3,3,3,3,3,3,3,3,
3,3,3,3,3,3,3,3,3,3,3,3,3,3,3,3,3,3,3,3,3,3,3,3,3,3,3,3,3,3,3,3,3,3,3,3,
3,3,3,3,3,4),(41.8093593517908,41.896925700064,41.9882599584125,42.0759549956636,
42.1637095871173,42.2515854767932,42.2622627334579,42.35012640214,42.4378801523619,
42.5255469200282,42.615945719514,42.7035155013069,42.7910727520387,42.8786380710294,
42.96623205827,43.0539223060446,43.1416703092467,43.229541791263,43.2487373159147,
43.3366009845863,43.4243547347969,43.5120215024516,43.6024203019415,43.6899900837217,
43.7775473344403,43.8651126534175,43.9527066406441,44.0403968884042,44.1281448915917,
44.216016373593,44.2352118983715,44.3230755672879,44.4108293177442,44.4984960856451,
44.588894885043,44.6764646670691,44.7640219180332,44.8515872372552,44.9391812247254,
45.0268714727266,45.1146194761536,45.2024909583908,45.2216864808283,45.3095501492757,
45.3973038992634,45.4849706666966,45.5753694662701,45.6629392478338,45.7504964983383,
45.8380618171039,45.9256558041216,46.0133460516777,46.1010940546639,46.1889655364693,
46.2081610632851,46.2951590562398,46.3820476809983,46.4688508233759,46.5555938060835,
46.6423059132212,46.7290085973227,46.8157232991051,46.9025184488413,46.9893581812461,
47.076320341889,47.1238898036606),.UNSPECIFIED.);
#1311=B_SPLINE_CURVE_WITH_KNOTS('',3,(#8045,#8046,#8047,#8048,#8049,#8050,
#8051,#8052,#8053,#8054,#8055,#8056,#8057,#8058,#8059,#8060,#8061,#8062,
#8063,#8064,#8065,#8066,#8067,#8068,#8069,#8070,#8071,#8072,#8073,#8074,
#8075,#8076,#8077,#8078,#8079,#8080,#8081),.UNSPECIFIED.,.F.,.F.,(4,3,3,
3,3,3,3,3,3,3,3,3,4),(47.1238898038469,47.1946356457419,47.2825045734518,
47.3702623111564,47.4605134717263,47.5481137855468,47.6356791061043,47.7232300467962,
47.8107872053906,47.8984076190842,47.9860664921885,48.0738212559678,48.0922715957158),
 .UNSPECIFIED.);
#1312=B_SPLINE_CURVE_WITH_KNOTS('',3,(#8083,#8084,#8085,#8086,#8087,#8088,
#8089,#8090,#8091,#8092,#8093,#8094,#8095,#8096,#8097,#8098,#8099,#8100,
#8101,#8102,#8103,#8104,#8105,#8106,#8107,#8108,#8109,#8110,#8111,#8112,
#8113,#8114,#8115,#8116,#8117,#8118,#8119),.UNSPECIFIED.,.F.,.F.,(4,3,3,
3,3,3,3,3,3,3,3,3,4),(47.1238898038469,47.2116835861261,47.2994728509267,
47.3872777931941,47.4751186140045,47.5630664520304,47.6510775151526,47.7392218004681,
47.7632743047295,47.8511215254599,47.9388724351879,48.026531246103,48.0930924415186),
 .UNSPECIFIED.);
#1313=B_SPLINE_CURVE_WITH_KNOTS('',3,(#8120,#8121,#8122,#8123,#8124,#8125,
#8126,#8127,#8128,#8129,#8130,#8131,#8132,#8133,#8134,#8135,#8136,#8137,
#8138,#8139,#8140,#8141,#8142,#8143,#8144,#8145,#8146,#8147,#8148,#8149,
#8150,#8151,#8152,#8153,#8154,#8155,#8156,#8157,#8158,#8159,#8160,#8161,
#8162,#8163,#8164,#8165,#8166,#8167,#8168,#8169,#8170,#8171,#8172,#8173,
#8174,#8175,#8176,#8177,#8178,#8179,#8180,#8181,#8182,#8183,#8184,#8185,
#8186,#8187,#8188,#8189,#8190,#8191,#8192,#8193,#8194,#8195,#8196,#8197,
#8198,#8199,#8200,#8201,#8202,#8203,#8204,#8205,#8206,#8207,#8208,#8209,
#8210,#8211,#8212,#8213,#8214,#8215,#8216,#8217,#8218,#8219,#8220,#8221,
#8222,#8223,#8224,#8225,#8226,#8227,#8228,#8229,#8230,#8231,#8232,#8233,
#8234,#8235,#8236,#8237,#8238,#8239,#8240,#8241,#8242,#8243,#8244,#8245,
#8246,#8247,#8248,#8249,#8250,#8251,#8252,#8253,#8254,#8255,#8256,#8257,
#8258,#8259,#8260,#8261,#8262,#8263,#8264,#8265,#8266,#8267,#8268,#8269,
#8270,#8271,#8272,#8273,#8274,#8275,#8276,#8277,#8278,#8279,#8280,#8281,
#8282,#8283,#8284,#8285,#8286,#8287,#8288,#8289,#8290,#8291,#8292,#8293,
#8294,#8295,#8296,#8297,#8298,#8299,#8300,#8301,#8302,#8303,#8304,#8305,
#8306,#8307,#8308,#8309,#8310,#8311,#8312,#8313,#8314,#8315),
 .UNSPECIFIED.,.F.,.F.,(4,3,3,3,3,3,3,3,3,3,3,3,3,3,3,3,3,3,3,3,3,3,3,3,
3,3,3,3,3,3,3,3,3,3,3,3,3,3,3,3,3,3,3,3,3,3,3,3,3,3,3,3,3,3,3,3,3,3,3,3,
3,3,3,3,3,4),(41.8092918158648,41.8444268099886,41.9322904786594,42.0200442288696,
42.107710996524,42.1981097960142,42.2856795777946,42.3732368285137,42.4608021474917,
42.5483961347192,42.6360863824806,42.7238343856694,42.8117058676723,42.8309013924454,
42.918765061131,43.0065188113555,43.094185579024,43.1845843785088,43.2721541603024,
43.3597114110342,43.4472767300246,43.5348707172641,43.6225609650369,43.7103089682367,
43.7981804502501,43.8173759749022,43.9052396436662,43.9929933939702,44.0806601617188,
44.1710589611738,44.258628743049,44.3461859938629,44.4337513129356,44.5213453002577,
44.6090355481129,44.6967835513953,44.7846550334906,44.803850557359,44.8917142260414,
44.9794679762634,45.0671347439299,45.1575335434156,45.2451033252088,45.3326605759407,
45.4202258949318,45.5078198821724,45.5955101299472,45.6832581331496,45.7711296151661,
45.7903251398158,45.8781888084878,45.9659425586989,46.0536093263539,46.1440081258437,
46.2315779076243,46.3191351583433,46.406700477321,46.494294464548,46.5819847123087,
46.6697327154966,46.7576041974983,46.7767997222726,46.8778180388024,46.9784525393735,
47.0783877221767,47.1238898036409),.UNSPECIFIED.);
#1314=B_SPLINE_CURVE_WITH_KNOTS('',3,(#8321,#8322,#8323,#8324,#8325,#8326,
#8327,#8328,#8329,#8330,#8331,#8332,#8333,#8334,#8335,#8336,#8337,#8338,
#8339,#8340,#8341,#8342,#8343,#8344,#8345,#8346,#8347,#8348,#8349,#8350,
#8351,#8352,#8353,#8354,#8355,#8356,#8357,#8358,#8359,#8360,#8361,#8362,
#8363,#8364,#8365,#8366,#8367,#8368,#8369,#8370,#8371,#8372,#8373,#8374,
#8375,#8376,#8377,#8378,#8379,#8380,#8381,#8382,#8383,#8384,#8385,#8386,
#8387,#8388,#8389,#8390,#8391,#8392,#8393,#8394,#8395,#8396,#8397,#8398,
#8399,#8400,#8401,#8402,#8403,#8404,#8405,#8406,#8407,#8408,#8409,#8410,
#8411,#8412,#8413,#8414,#8415,#8416,#8417,#8418,#8419,#8420,#8421,#8422,
#8423,#8424,#8425,#8426,#8427,#8428,#8429,#8430,#8431,#8432,#8433,#8434,
#8435,#8436,#8437,#8438,#8439,#8440,#8441,#8442,#8443,#8444,#8445,#8446,
#8447,#8448,#8449,#8450,#8451,#8452,#8453,#8454,#8455,#8456,#8457,#8458,
#8459,#8460,#8461,#8462,#8463,#8464,#8465,#8466,#8467,#8468,#8469,#8470,
#8471,#8472,#8473,#8474,#8475,#8476,#8477,#8478,#8479,#8480,#8481,#8482,
#8483,#8484,#8485,#8486,#8487,#8488,#8489,#8490,#8491,#8492,#8493,#8494,
#8495,#8496,#8497,#8498,#8499,#8500,#8501,#8502,#8503,#8504,#8505,#8506,
#8507,#8508,#8509,#8510,#8511,#8512,#8513),.UNSPECIFIED.,.F.,.F.,(4,3,3,
3,3,3,3,3,3,3,3,3,3,3,3,3,3,3,3,3,3,3,3,3,3,3,3,3,3,3,3,3,3,3,3,3,3,3,3,
3,3,3,3,3,3,3,3,3,3,3,3,3,3,3,3,3,3,3,3,3,3,3,3,3,4),(35.5268366911762,
35.6145084367687,35.7056217870122,35.7931929079879,35.8807503212151,35.9683146264148,
36.0559064231432,36.1435939353638,36.2313381445587,36.3192071347035,36.343415238717,
36.431278907217,36.5190326572565,36.6066994247405,36.6970982242947,36.784668005907,
36.872225256459,36.9597905752715,37.0473845623344,37.1350748099347,37.2228228129641,
37.3106942948111,37.3298898211739,37.4177534896489,37.505507239659,37.5931740071094,
37.6835728066745,37.7711425882421,37.8586998387456,37.946265157505,38.0338591445114,
38.1215493920497,38.2092973950135,38.2971688767908,38.3163644036307,38.4042280725361,
38.4919818229839,38.5796485908782,38.6700473902794,38.7576171723039,38.8451744232686,
38.9327397424928,39.0203337299674,39.1080239779757,39.1957719814113,39.2836434636597,
39.3028389860875,39.3907026547579,39.4784564049676,39.5661231726209,39.6565219721114,
39.7440917538913,39.8316490046101,39.9192143235875,40.0068083108156,40.0944985585765,
40.1822465617651,40.2701180437678,40.2893135685443,40.3795378388649,40.4696301596092,
40.5623987438737,40.6522493144927,40.74647690558,40.8407044966673),
 .UNSPECIFIED.);
#1315=B_SPLINE_CURVE_WITH_KNOTS('',3,(#8514,#8515,#8516,#8517,#8518,#8519,
#8520,#8521,#8522,#8523,#8524,#8525,#8526,#8527,#8528,#8529,#8530,#8531,
#8532,#8533,#8534,#8535,#8536,#8537,#8538,#8539,#8540,#8541,#8542,#8543,
#8544,#8545,#8546,#8547),.UNSPECIFIED.,.F.,.F.,(4,3,3,3,3,3,3,3,3,3,3,4),
(40.840704496799,40.9348549665562,41.0293618567931,41.1240517300647,41.2190251707754,
41.2757881510011,41.3636473621912,41.451401427047,41.540890908233,41.6284903539905,
41.7189248528907,41.8093593517908),.UNSPECIFIED.);
#1316=B_SPLINE_CURVE_WITH_KNOTS('',3,(#8549,#8550,#8551,#8552,#8553,#8554,
#8555,#8556,#8557,#8558,#8559,#8560,#8561,#8562,#8563,#8564,#8565,#8566,
#8567,#8568,#8569,#8570,#8571,#8572,#8573,#8574,#8575,#8576,#8577,#8578,
#8579,#8580,#8581,#8582,#8583,#8584,#8585),.UNSPECIFIED.,.F.,.F.,(4,3,3,
3,3,3,3,3,3,3,3,3,4),(40.8407044966673,40.8579522275318,40.9458179320816,
41.0335732153263,41.121241015274,41.2088441090132,41.2964126890953,41.3839673694283,
41.4715287488756,41.5591660707284,41.6468417480247,41.7346436206963,41.8092918158648),
 .UNSPECIFIED.);
#1317=B_SPLINE_CURVE_WITH_KNOTS('',3,(#8586,#8587,#8588,#8589,#8590,#8591,
#8592,#8593,#8594,#8595,#8596,#8597,#8598,#8599,#8600,#8601,#8602,#8603,
#8604,#8605,#8606,#8607,#8608,#8609,#8610,#8611,#8612,#8613,#8614,#8615,
#8616,#8617,#8618,#8619,#8620,#8621,#8622,#8623,#8624,#8625,#8626,#8627,
#8628,#8629,#8630,#8631,#8632,#8633,#8634,#8635,#8636,#8637,#8638,#8639,
#8640,#8641,#8642,#8643,#8644,#8645,#8646,#8647,#8648,#8649,#8650,#8651,
#8652,#8653,#8654,#8655,#8656,#8657,#8658,#8659,#8660,#8661,#8662,#8663,
#8664,#8665,#8666,#8667,#8668,#8669,#8670,#8671,#8672,#8673,#8674,#8675,
#8676,#8677,#8678,#8679,#8680,#8681,#8682,#8683,#8684,#8685,#8686,#8687,
#8688,#8689,#8690,#8691,#8692,#8693,#8694,#8695,#8696,#8697,#8698,#8699,
#8700,#8701,#8702,#8703,#8704,#8705,#8706,#8707,#8708,#8709,#8710,#8711,
#8712,#8713,#8714,#8715,#8716,#8717,#8718,#8719,#8720,#8721,#8722,#8723,
#8724,#8725,#8726,#8727,#8728,#8729,#8730,#8731,#8732,#8733,#8734,#8735,
#8736,#8737,#8738,#8739,#8740,#8741,#8742,#8743,#8744,#8745,#8746,#8747,
#8748,#8749,#8750,#8751,#8752,#8753,#8754,#8755,#8756,#8757,#8758,#8759,
#8760,#8761,#8762,#8763,#8764,#8765,#8766,#8767,#8768,#8769,#8770,#8771,
#8772,#8773,#8774,#8775,#8776,#8777,#8778),.UNSPECIFIED.,.F.,.F.,(4,3,3,
3,3,3,3,3,3,3,3,3,3,3,3,3,3,3,3,3,3,3,3,3,3,3,3,3,3,3,3,3,3,3,3,3,3,3,3,
3,3,3,3,3,3,3,3,3,3,3,3,3,3,3,3,3,3,3,3,3,3,3,3,3,4),(35.5260257192705,
35.6136077753379,35.7012827832995,35.7890093143363,35.8768671942592,35.9255793152477,
36.0134429833182,36.1011967329437,36.1888635000296,36.279262299739,36.3668320809955,
36.4543893312083,36.5419546496982,36.6295486364565,36.7172388837792,36.8049868865467,
36.8928583681567,36.9120538977045,36.9999175641475,37.0876713120909,37.1753380774423,
37.2657368777822,37.3533066571848,37.4408639055025,37.5284292220579,37.6160232068443,
37.7037134521494,37.7914614528703,37.8793329324066,37.8985284801614,37.9863921502957,
38.0741459019874,38.1618126711394,38.2522114700742,38.3397812533827,38.4273385056385,
38.51490382616,38.6024978149364,38.6901880642466,38.777936068986,38.8658075525305,
38.8850030626182,38.9728667311203,39.060620481162,39.1482872486483,39.2386860482016,
39.3262558298162,39.4138130803705,39.5013783991851,39.5889723862506,39.6766626338531,
39.7644106368846,39.8522821187338,39.871477645075,39.9590839627409,40.046580472658,
40.1339904231532,40.2223296823268,40.3096449944239,40.3969485865632,40.4842613371711,
40.5733721270138,40.6608118986615,40.7507581976017,40.8407044965419),
 .UNSPECIFIED.);
#1318=B_SPLINE_CURVE_WITH_KNOTS('',3,(#8784,#8785,#8786,#8787,#8788,#8789,
#8790,#8791,#8792,#8793,#8794,#8795,#8796,#8797,#8798,#8799,#8800,#8801,
#8802,#8803,#8804,#8805,#8806,#8807,#8808,#8809,#8810,#8811,#8812,#8813,
#8814,#8815,#8816,#8817,#8818,#8819,#8820,#8821,#8822,#8823,#8824,#8825,
#8826,#8827,#8828,#8829,#8830,#8831,#8832,#8833,#8834,#8835,#8836,#8837,
#8838,#8839,#8840,#8841,#8842,#8843,#8844,#8845,#8846,#8847,#8848,#8849,
#8850,#8851,#8852,#8853,#8854,#8855,#8856,#8857,#8858,#8859,#8860,#8861,
#8862,#8863,#8864,#8865,#8866,#8867,#8868,#8869,#8870,#8871,#8872,#8873,
#8874,#8875,#8876,#8877,#8878,#8879,#8880,#8881,#8882,#8883,#8884,#8885,
#8886,#8887,#8888,#8889,#8890,#8891,#8892,#8893,#8894,#8895,#8896,#8897,
#8898,#8899,#8900,#8901,#8902,#8903,#8904,#8905,#8906,#8907,#8908,#8909,
#8910,#8911,#8912,#8913,#8914,#8915,#8916,#8917,#8918,#8919,#8920,#8921,
#8922,#8923,#8924,#8925,#8926,#8927,#8928,#8929,#8930,#8931,#8932,#8933,
#8934,#8935,#8936,#8937,#8938,#8939,#8940,#8941,#8942,#8943,#8944,#8945,
#8946,#8947,#8948,#8949,#8950,#8951,#8952,#8953,#8954,#8955,#8956,#8957,
#8958,#8959,#8960,#8961,#8962,#8963,#8964,#8965,#8966,#8967,#8968,#8969,
#8970,#8971,#8972,#8973,#8974,#8975,#8976,#8977,#8978,#8979),
 .UNSPECIFIED.,.F.,.F.,(4,3,3,3,3,3,3,3,3,3,3,3,3,3,3,3,3,3,3,3,3,3,3,3,
3,3,3,3,3,3,3,3,3,3,3,3,3,3,3,3,3,3,3,3,3,3,3,3,3,3,3,3,3,3,3,3,3,3,3,3,
3,3,3,3,3,4),(29.2425482859762,29.3302955402787,29.4181664625321,29.4380931615194,
29.525956904785,29.613710730384,29.7013775741223,29.791776345354,29.8793462044527,
29.9669035328111,30.0544689296637,30.1420629949156,30.2297533205319,30.3175014015646,
30.4053729608139,30.4245677439762,30.5124314160683,30.6001851699415,30.687851941495,
30.7782507396122,30.8658205258578,30.9533777812449,31.0409431050895,31.1285370973784,
31.2162273504652,31.3039753591402,31.3918468468228,31.411042326433,31.4989059745539,
31.5866597038815,31.6743264503483,31.764725257666,31.8522950176361,31.9398522463518,
32.0274175431573,32.1150115080668,32.202701733406,32.2904497140863,32.3783211736226,
32.3975169088898,32.4853805881456,32.5731343490644,32.660801127537,32.7511999230132,
32.8387697158143,32.9263269776097,33.0138923077074,33.101486306086,33.1891765649889,
33.2769245793264,33.3647960724051,33.3839914913466,33.4718551594076,33.5596089090236,
33.6472756761,33.737674475813,33.8252442570602,33.9128015072637,34.0003668257444,
34.0879608124935,34.1756510598073,34.2633990625659,34.3512705441674,34.3704660738034,
34.4979605070231,34.5575191894877),.UNSPECIFIED.);
#1319=B_SPLINE_CURVE_WITH_KNOTS('',3,(#8980,#8981,#8982,#8983,#8984,#8985,
#8986,#8987,#8988,#8989,#8990,#8991,#8992,#8993,#8994,#8995,#8996,#8997,
#8998,#8999,#9000,#9001,#9002,#9003,#9004,#9005,#9006,#9007,#9008,#9009,
#9010,#9011,#9012,#9013,#9014,#9015,#9016),.UNSPECIFIED.,.F.,.F.,(4,3,3,
3,3,3,3,3,3,3,3,3,4),(34.5575191896929,34.6439788935642,34.7330991139012,
34.8194341984083,34.9057479013124,34.9920619722673,35.0783981577317,35.1648239857159,
35.2513038501986,35.3379043039037,35.3569406562602,35.4447862511981,35.5268366911762),
 .UNSPECIFIED.);
#1320=B_SPLINE_CURVE_WITH_KNOTS('',3,(#9018,#9019,#9020,#9021,#9022,#9023,
#9024,#9025,#9026,#9027,#9028,#9029,#9030,#9031,#9032,#9033,#9034,#9035,
#9036,#9037,#9038,#9039,#9040,#9041,#9042,#9043,#9044,#9045,#9046,#9047,
#9048,#9049,#9050,#9051),.UNSPECIFIED.,.F.,.F.,(4,3,3,3,3,3,3,3,3,3,3,4),
(34.5575191896899,34.6549831946974,34.7527736528568,34.8510352792918,34.9391047327909,
35.0269585210482,35.1147082551822,35.2023747117386,35.289976688806,35.3775401437585,
35.465101297594,35.5260257192705),.UNSPECIFIED.);
#1321=B_SPLINE_CURVE_WITH_KNOTS('',3,(#9052,#9053,#9054,#9055,#9056,#9057,
#9058,#9059,#9060,#9061,#9062,#9063,#9064,#9065,#9066,#9067,#9068,#9069,
#9070,#9071,#9072,#9073,#9074,#9075,#9076,#9077,#9078,#9079,#9080,#9081,
#9082,#9083,#9084,#9085,#9086,#9087,#9088,#9089,#9090,#9091,#9092,#9093,
#9094,#9095,#9096,#9097,#9098,#9099,#9100,#9101,#9102,#9103,#9104,#9105,
#9106,#9107,#9108,#9109,#9110,#9111,#9112,#9113,#9114,#9115,#9116,#9117,
#9118,#9119,#9120,#9121,#9122,#9123,#9124,#9125,#9126,#9127,#9128,#9129,
#9130,#9131,#9132,#9133,#9134,#9135,#9136,#9137,#9138,#9139,#9140,#9141,
#9142,#9143,#9144,#9145,#9146,#9147,#9148,#9149,#9150,#9151,#9152,#9153,
#9154,#9155,#9156,#9157,#9158,#9159,#9160,#9161,#9162,#9163,#9164,#9165,
#9166,#9167,#9168,#9169,#9170,#9171,#9172,#9173,#9174,#9175,#9176,#9177,
#9178,#9179,#9180,#9181,#9182,#9183,#9184,#9185,#9186,#9187,#9188,#9189,
#9190,#9191,#9192,#9193,#9194,#9195,#9196,#9197,#9198,#9199,#9200,#9201,
#9202,#9203,#9204,#9205,#9206,#9207,#9208,#9209,#9210,#9211,#9212,#9213,
#9214,#9215,#9216,#9217,#9218,#9219,#9220,#9221,#9222,#9223,#9224,#9225,
#9226,#9227,#9228,#9229,#9230,#9231,#9232,#9233,#9234,#9235,#9236,#9237,
#9238,#9239,#9240,#9241,#9242,#9243,#9244),.UNSPECIFIED.,.F.,.F.,(4,3,3,
3,3,3,3,3,3,3,3,3,3,3,3,3,3,3,3,3,3,3,3,3,3,3,3,3,3,3,3,3,3,3,3,3,3,3,3,
3,3,3,3,3,3,3,3,3,3,3,3,3,3,3,3,3,3,3,3,3,3,3,3,3,4),(29.243664967692,29.3312944627721,
29.4188783169648,29.5064396083037,29.5939989404945,29.6815769108029,29.7692462733555,
29.8569643702558,29.9448174904114,30.0067318205069,30.0945955831954,30.1823494302193,
30.2700162973492,30.360415060551,30.447984947815,30.5355423060676,30.6231077345184,
30.7107018330489,30.7983921942754,30.8861403123251,30.9740119103669,30.9932064029637,
31.0810698948999,31.1688234656784,31.2564900514433,31.3468889181904,31.4344585131339,
31.522015575508,31.6095807048371,31.697174501315,31.7848645576492,31.872612368797,
31.9604836592968,31.9796809854205,32.0675447282664,32.1552985534412,32.2429653967515,
32.3333641681422,32.420934026805,32.5084913547255,32.5960567511386,32.6836508159498,
32.771341141126,32.8590892217185,32.9469607805306,32.9661555678773,33.0540192399948,
33.1417729938924,33.2294397654696,33.3198385635777,33.4074083498455,33.4949656052541,
33.5825309291192,33.6701249214278,33.7578151745333,33.8455631832266,33.9334346709259,
33.9526301503341,34.0414524496082,34.1301581696792,34.2187666849647,34.3072860964107,
34.395752460746,34.484192796774,34.5575191894877),.UNSPECIFIED.);
#1322=B_SPLINE_CURVE_WITH_KNOTS('',3,(#9250,#9251,#9252,#9253,#9254,#9255,
#9256,#9257,#9258,#9259,#9260,#9261,#9262,#9263,#9264,#9265,#9266,#9267,
#9268,#9269,#9270,#9271,#9272,#9273,#9274,#9275,#9276,#9277,#9278,#9279,
#9280,#9281,#9282,#9283),.UNSPECIFIED.,.F.,.F.,(4,3,3,3,3,3,3,3,3,3,3,4),
(21.9911485751285,22.1149351608524,22.2027160146711,22.2903837338802,22.3779478024412,
22.4654536992169,22.5529221753128,22.6403739494206,22.7278622838359,22.8153692328211,
22.9029614226615,22.959407626261),.UNSPECIFIED.);
#1323=B_SPLINE_CURVE_WITH_KNOTS('',3,(#9285,#9286,#9287,#9288,#9289,#9290,
#9291),.UNSPECIFIED.,.F.,.F.,(4,1,1,1,4),(18.1690368310252,19.155511413482,
20.1419859959388,21.1284605783956,21.9911407069303),.UNSPECIFIED.);
#1324=B_SPLINE_CURVE_WITH_KNOTS('',3,(#9295,#9296,#9297,#9298,#9299,#9300,
#9301,#9302,#9303,#9304,#9305,#9306,#9307,#9308,#9309,#9310,#9311,#9312,
#9313,#9314,#9315,#9316,#9317,#9318,#9319,#9320,#9321,#9322,#9323,#9324,
#9325,#9326,#9327,#9328,#9329,#9330,#9331,#9332,#9333,#9334,#9335,#9336,
#9337,#9338,#9339,#9340,#9341,#9342,#9343,#9344,#9345,#9346,#9347,#9348,
#9349,#9350,#9351,#9352,#9353,#9354,#9355,#9356,#9357,#9358,#9359,#9360,
#9361,#9362,#9363,#9364,#9365,#9366,#9367,#9368,#9369,#9370,#9371,#9372,
#9373,#9374,#9375,#9376,#9377,#9378,#9379,#9380,#9381,#9382,#9383,#9384,
#9385,#9386,#9387,#9388,#9389,#9390,#9391,#9392,#9393,#9394,#9395,#9396,
#9397,#9398,#9399,#9400,#9401,#9402,#9403,#9404,#9405,#9406,#9407,#9408,
#9409,#9410,#9411,#9412,#9413,#9414,#9415,#9416,#9417,#9418,#9419,#9420,
#9421,#9422,#9423,#9424,#9425,#9426,#9427,#9428,#9429,#9430,#9431,#9432,
#9433,#9434,#9435,#9436,#9437,#9438,#9439,#9440,#9441,#9442,#9443,#9444,
#9445,#9446,#9447,#9448,#9449,#9450,#9451),.UNSPECIFIED.,.F.,.F.,(4,3,3,
3,3,3,3,3,3,3,3,3,3,3,3,3,3,3,3,3,3,3,3,3,3,3,3,3,3,3,3,3,3,3,3,3,3,3,3,
3,3,3,3,3,3,3,3,3,3,3,3,3,4),(17.6451204658269,17.7324138960806,17.8195992142952,
17.9066999959299,17.9937421922357,18.080753937747,18.167756417921,18.2547708066079,
18.3418700810798,18.4290131909813,18.5162907440526,18.5868727544945,18.6748711844211,
18.7627621489718,18.8505683956313,18.9409157632963,19.0286297421553,19.1163326847563,
19.2040450297739,19.2963706065682,19.3842126461842,19.4721141501259,19.5601379184068,
19.5733473369513,19.661119323604,19.7487802196365,19.8363530814819,19.9267866862227,
20.0142605428918,20.1017212859224,20.1891896184029,20.2766862438119,20.3642790579177,
20.4519294732645,20.5397038712882,20.5598219194081,20.6477025677944,20.7354733506331,
20.8231571819731,20.9135495969596,21.0011364059084,21.0887106394504,21.1762928775113,
21.2639037006302,21.3516105759406,21.4393751033165,21.5272628354399,21.5462965018649,
21.6407892334465,21.7349872067073,21.8290035864883,21.9227454576979,21.9911485749053),
 .UNSPECIFIED.);
#1325=B_SPLINE_CURVE_WITH_KNOTS('',3,(#9452,#9453,#9454,#9455,#9456,#9457,
#9458,#9459,#9460,#9461,#9462,#9463,#9464,#9465,#9466,#9467,#9468,#9469,
#9470,#9471,#9472,#9473,#9474,#9475,#9476,#9477,#9478,#9479,#9480,#9481,
#9482,#9483,#9484,#9485),.UNSPECIFIED.,.F.,.F.,(4,3,3,3,3,3,3,3,3,3,3,4),
(21.9911485751285,22.081189059175,22.1712954056986,22.2616643253544,22.3520075127491,
22.442539438158,22.5327710843217,22.6206308683745,22.7083577673478,22.7960076583844,
22.8835975443804,22.9601178369312),.UNSPECIFIED.);
#1326=B_SPLINE_CURVE_WITH_KNOTS('',3,(#9491,#9492,#9493,#9494),
 .UNSPECIFIED.,.F.,.F.,(4,4),(47.7645509873098,47.8044058628387),
 .UNSPECIFIED.);
#1327=B_SPLINE_CURVE_WITH_KNOTS('',3,(#9496,#9497,#9498,#9499,#9500,#9501,
#9502,#9503,#9504,#9505,#9506,#9507,#9508,#9509,#9510,#9511,#9512,#9513,
#9514,#9515,#9516,#9517,#9518,#9519,#9520,#9521,#9522,#9523,#9524,#9525,
#9526,#9527,#9528,#9529,#9530,#9531,#9532,#9533,#9534,#9535,#9536,#9537,
#9538,#9539,#9540,#9541,#9542,#9543,#9544,#9545,#9546,#9547,#9548,#9549,
#9550,#9551,#9552,#9553,#9554,#9555,#9556,#9557,#9558,#9559,#9560,#9561,
#9562,#9563,#9564,#9565,#9566,#9567,#9568,#9569,#9570,#9571,#9572,#9573,
#9574,#9575,#9576,#9577,#9578,#9579,#9580,#9581,#9582,#9583,#9584,#9585,
#9586,#9587,#9588,#9589,#9590,#9591,#9592,#9593,#9594,#9595,#9596,#9597,
#9598,#9599,#9600,#9601,#9602,#9603,#9604,#9605,#9606,#9607,#9608,#9609,
#9610,#9611,#9612,#9613,#9614,#9615,#9616,#9617,#9618,#9619,#9620,#9621,
#9622,#9623,#9624,#9625,#9626,#9627,#9628,#9629,#9630,#9631,#9632,#9633,
#9634,#9635,#9636,#9637,#9638,#9639,#9640,#9641,#9642,#9643,#9644,#9645,
#9646),.UNSPECIFIED.,.F.,.F.,(4,3,3,3,3,3,3,3,3,3,3,3,3,3,3,3,3,3,3,3,3,
3,3,3,3,3,3,3,3,3,3,3,3,3,3,3,3,3,3,3,3,3,3,3,3,3,3,3,3,3,4),(47.8044088943605,
47.8988458715296,47.9933637699636,48.0880590284704,48.1828496682947,48.2778377921346,
48.3372545403837,48.4294696563408,48.5215643431454,48.6135647748162,48.7054993456098,
48.7973996202586,48.889289121424,48.9811913568557,49.0731852010223,49.1652272928627,
49.257412825594,49.3237291228405,49.41585789497,49.5078683040179,49.5997866059479,
49.6916425715041,49.7834664330782,49.8752817926359,49.9671122390392,50.0590383362072,
50.1510148357375,50.243138907479,50.3102037052973,50.4014179770184,50.4925118584179,
50.5835127350798,50.6744535421951,50.7653638250799,50.8562681794588,50.9471911906559,
51.0382208929196,51.1293056432464,51.2205548827498,51.2966782877541,51.3911470133568,
51.4854792917811,51.5796967693301,51.6738054165067,51.7678505381326,51.8618515310768,
51.9558277481792,52.0498237215135,52.1438284502303,52.2378954387847,52.2831528702109),
 .UNSPECIFIED.);
#1328=B_SPLINE_CURVE_WITH_KNOTS('',3,(#9650,#9651,#9652,#9653,#9654,#9655,
#9656,#9657,#9658,#9659,#9660,#9661,#9662,#9663,#9664,#9665,#9666,#9667,
#9668,#9669,#9670,#9671,#9672,#9673,#9674,#9675,#9676,#9677,#9678,#9679,
#9680,#9681,#9682,#9683,#9684,#9685,#9686,#9687,#9688,#9689,#9690,#9691,
#9692,#9693,#9694,#9695,#9696,#9697,#9698,#9699,#9700,#9701,#9702,#9703,
#9704,#9705,#9706,#9707,#9708,#9709,#9710,#9711,#9712,#9713,#9714,#9715,
#9716,#9717,#9718,#9719,#9720,#9721,#9722,#9723,#9724,#9725,#9726,#9727,
#9728,#9729,#9730,#9731,#9732,#9733,#9734,#9735,#9736,#9737,#9738,#9739,
#9740,#9741,#9742,#9743,#9744,#9745,#9746,#9747,#9748,#9749,#9750,#9751,
#9752,#9753,#9754,#9755,#9756,#9757,#9758,#9759,#9760,#9761,#9762,#9763,
#9764,#9765,#9766,#9767,#9768,#9769,#9770,#9771,#9772,#9773,#9774,#9775,
#9776,#9777,#9778,#9779,#9780,#9781,#9782,#9783,#9784,#9785,#9786,#9787,
#9788,#9789,#9790,#9791,#9792,#9793,#9794,#9795,#9796,#9797,#9798,#9799,
#9800,#9801,#9802,#9803,#9804,#9805,#9806,#9807,#9808,#9809,#9810,#9811,
#9812,#9813,#9814,#9815,#9816,#9817,#9818,#9819,#9820,#9821,#9822,#9823,
#9824,#9825,#9826,#9827,#9828,#9829,#9830,#9831,#9832,#9833,#9834,#9835,
#9836,#9837,#9838,#9839,#9840,#9841,#9842,#9843,#9844,#9845,#9846,#9847,
#9848,#9849,#9850,#9851,#9852,#9853,#9854,#9855,#9856,#9857),
 .UNSPECIFIED.,.F.,.F.,(4,3,3,3,3,3,3,3,3,3,3,3,3,3,3,3,3,3,3,3,3,3,3,3,
3,3,3,3,3,3,3,3,3,3,3,3,3,3,3,3,3,3,3,3,3,3,3,3,3,3,3,3,3,3,3,3,3,3,3,3,
3,3,3,3,3,3,3,3,3,4),(-50.2654642069239,-50.174002871108,-50.0826595972117,
-49.9877932879153,-49.8966027347253,-49.8054407495249,-49.7142829692658,
-49.6231050404631,-49.5318321853382,-49.440502858591,-49.3490411078306,
-49.3237291228405,-49.2315291015422,-49.1394464590948,-49.0474550341997,
-48.9555248846661,-48.8636262123592,-48.7717354971473,-48.6798292315804,
-48.5878270327216,-48.4957741651475,-48.4035740334089,-48.3372545403837,
-48.245291774167,-48.1534503585896,-48.0617037771693,-47.9700228870573,
-47.8783760922691,-47.7867395670033,-47.6950894999377,-47.6033450470191,
-47.5115511593569,-47.4196094077833,-47.3507799579269,-47.2587033417908,
-47.1667467351112,-47.0748837851034,-46.9830852378435,-46.8913200370523,
-46.7995644990034,-46.7077949539867,-46.6159310309032,-46.5240175020027,
-46.4319570406068,-46.36430537547,-46.2722322020199,-46.1802787999358,-46.088418812967,
-45.9966228505351,-45.9048600007786,-45.8131065761715,-45.7213389030145,
-45.6294764629031,-45.5375642026684,-45.4455046445268,-45.3778307930132,
-45.285784361828,-45.1938581747992,-45.1020258358177,-45.0102580580154,
-44.9185237121079,-44.8267990763685,-44.7350604431189,-44.6432272555675,
-44.5513444087202,-44.4593142303005,-44.3913562105564,-44.2836645683137,
-44.1732379897799,-44.0628114112462),.UNSPECIFIED.);
#1329=B_SPLINE_CURVE_WITH_KNOTS('',3,(#9858,#9859,#9860,#9861),
 .UNSPECIFIED.,.F.,.F.,(4,4),(-44.062811411082,-44.0219726945388),
 .UNSPECIFIED.);
#1330=B_SPLINE_CURVE_WITH_KNOTS('',3,(#9867,#9868,#9869,#9870),
 .UNSPECIFIED.,.F.,.F.,(4,4),(41.481273340989,41.5212235871809),
 .UNSPECIFIED.);
#1331=B_SPLINE_CURVE_WITH_KNOTS('',3,(#9871,#9872,#9873,#9874,#9875,#9876,
#9877,#9878,#9879,#9880),.UNSPECIFIED.,.F.,.F.,(4,1,1,1,1,1,1,4),(41.5212316192577,
42.4184070456428,43.4048816280996,44.3913562105564,45.3778307930133,46.3643053754701,
47.3507799579269,47.7645509873098),.UNSPECIFIED.);
#1332=B_SPLINE_CURVE_WITH_KNOTS('',3,(#9882,#9883,#9884,#9885,#9886,#9887,
#9888,#9889,#9890,#9891,#9892,#9893,#9894,#9895,#9896,#9897,#9898,#9899,
#9900,#9901,#9902,#9903,#9904,#9905,#9906,#9907,#9908,#9909,#9910,#9911,
#9912,#9913,#9914,#9915,#9916,#9917,#9918,#9919,#9920,#9921,#9922,#9923,
#9924,#9925,#9926,#9927,#9928,#9929,#9930,#9931,#9932,#9933,#9934,#9935,
#9936,#9937,#9938,#9939,#9940,#9941,#9942,#9943,#9944,#9945,#9946,#9947,
#9948,#9949,#9950,#9951,#9952,#9953,#9954,#9955,#9956,#9957,#9958,#9959,
#9960,#9961,#9962,#9963,#9964,#9965,#9966,#9967,#9968,#9969,#9970,#9971,
#9972,#9973,#9974,#9975,#9976,#9977,#9978,#9979,#9980,#9981,#9982,#9983,
#9984,#9985,#9986,#9987,#9988,#9989,#9990,#9991,#9992,#9993,#9994,#9995,
#9996,#9997,#9998,#9999,#10000,#10001,#10002,#10003,#10004,#10005,#10006,
#10007,#10008,#10009,#10010,#10011,#10012,#10013,#10014,#10015,#10016,#10017,
#10018,#10019,#10020,#10021,#10022,#10023,#10024,#10025,#10026,#10027,#10028,
#10029,#10030,#10031,#10032,#10033,#10034,#10035,#10036,#10037,#10038,#10039,
#10040,#10041,#10042,#10043,#10044,#10045,#10046,#10047,#10048,#10049,#10050,
#10051,#10052,#10053,#10054,#10055,#10056,#10057,#10058,#10059,#10060,#10061,
#10062,#10063,#10064,#10065,#10066,#10067,#10068,#10069,#10070,#10071,#10072,
#10073,#10074,#10075,#10076,#10077,#10078,#10079,#10080,#10081,#10082,#10083,
#10084,#10085,#10086,#10087,#10088,#10089,#10090,#10091,#10092),
 .UNSPECIFIED.,.F.,.F.,(4,3,3,3,3,3,3,3,3,3,3,3,3,3,3,3,3,3,3,3,3,3,3,3,
3,3,3,3,3,3,3,3,3,3,3,3,3,3,3,3,3,3,3,3,3,3,3,3,3,3,3,3,3,3,3,3,3,3,3,3,
3,3,3,3,3,3,3,3,3,3,4),(-44.0219726945388,-43.9302993798164,-43.8386303041183,
-43.746941779298,-43.6551507631959,-43.5633054158736,-43.4713063922967,
-43.4048816280996,-43.3128214862464,-43.2208813800638,-43.1290349336417,
-43.0372528238165,-42.9455040132506,-42.8537647976379,-42.7620114866317,
-42.6701635590492,-42.5782659160732,-42.4862209992494,-42.4184070456428,
-42.3263497646008,-42.234412573871,-42.1425690932578,-42.0507900127371,
-41.9590442693662,-41.8673081551732,-41.7755579761731,-41.6837132090212,
-41.5918187468843,-41.4997770122276,-41.431932463186,-41.3398731138376,
-41.2479338264137,-41.1560882237537,-41.0643069919101,-40.9725590800402,
-40.880820782799,-40.7890684088164,-40.6972214416019,-40.6053247733791,
-40.5132808450966,-40.4454578807292,-40.3533989564471,-40.2614600960634,
-40.1696149218158,-40.0778341186257,-39.9860866353904,-39.8943487662328,
-39.8025968192505,-39.7107502747056,-39.6188540273564,-39.5268105127238,
-39.4589832982724,-39.3669246585381,-39.2749860887432,-39.183141210696,
-39.0913607109285,-38.9996135354415,-38.9078759779926,-38.816124346316,
-38.724278120748,-38.6323821948822,-38.5403390025968,-38.4725087158156,
-38.3810288132208,-38.2896616015582,-38.1983825809915,-38.1071673347784,
-38.0159770156749,-37.9248025582061,-37.8335885854587,-37.7796261039024),
 .UNSPECIFIED.);
#1333=B_SPLINE_CURVE_WITH_KNOTS('',3,(#10093,#10094,#10095,#10096),
 .UNSPECIFIED.,.F.,.F.,(4,4),(-37.7796261036537,-37.7402431363199),
 .UNSPECIFIED.);
#1334=B_SPLINE_CURVE_WITH_KNOTS('',3,(#10102,#10103,#10104,#10105),
 .UNSPECIFIED.,.F.,.F.,(4,4),(-0.01489375026152,-0.000951714991103148),
 .UNSPECIFIED.);
#1335=B_SPLINE_CURVE_WITH_KNOTS('',3,(#10106,#10107,#10108,#10109,#10110,
#10111,#10112,#10113,#10114,#10115,#10116,#10117,#10118,#10119,#10120,#10121,
#10122,#10123,#10124,#10125,#10126,#10127,#10128,#10129,#10130,#10131,#10132,
#10133,#10134,#10135,#10136,#10137,#10138,#10139,#10140,#10141,#10142,#10143,
#10144,#10145,#10146,#10147,#10148,#10149,#10150,#10151,#10152,#10153,#10154,
#10155,#10156,#10157,#10158,#10159,#10160,#10161,#10162,#10163,#10164,#10165,
#10166,#10167,#10168,#10169,#10170,#10171,#10172,#10173,#10174,#10175,#10176,
#10177,#10178,#10179,#10180,#10181,#10182,#10183,#10184,#10185,#10186,#10187,
#10188,#10189,#10190,#10191,#10192,#10193,#10194,#10195,#10196,#10197,#10198,
#10199,#10200,#10201,#10202,#10203,#10204,#10205,#10206,#10207,#10208,#10209,
#10210,#10211,#10212,#10213,#10214,#10215,#10216,#10217,#10218,#10219,#10220,
#10221,#10222,#10223,#10224,#10225,#10226,#10227,#10228,#10229,#10230,#10231,
#10232,#10233,#10234,#10235,#10236,#10237,#10238,#10239,#10240,#10241,#10242,
#10243,#10244,#10245,#10246,#10247,#10248,#10249,#10250,#10251,#10252,#10253,
#10254,#10255,#10256,#10257,#10258,#10259,#10260,#10261,#10262,#10263,#10264,
#10265,#10266,#10267,#10268,#10269,#10270,#10271,#10272,#10273,#10274,#10275,
#10276,#10277,#10278,#10279,#10280,#10281,#10282,#10283,#10284,#10285,#10286,
#10287,#10288,#10289,#10290,#10291,#10292,#10293,#10294,#10295,#10296,#10297,
#10298,#10299,#10300,#10301,#10302,#10303,#10304,#10305,#10306,#10307,#10308,
#10309,#10310,#10311,#10312,#10313,#10314,#10315,#10316),.UNSPECIFIED.,
 .F.,.F.,(4,3,3,3,3,3,3,3,3,3,3,3,3,3,3,3,3,3,3,3,3,3,3,3,3,3,3,3,3,3,3,
3,3,3,3,3,3,3,3,3,3,3,3,3,3,3,3,3,3,3,3,3,3,3,3,3,3,3,3,3,3,3,3,3,3,3,3,
3,3,3,4),(35.2380382801875,35.3506623506834,35.4649882294613,35.5130849684452,
35.6051437708323,35.6970825062651,35.7889275526903,35.8807082242548,35.9724555735748,
36.0641933066831,36.1559451156365,36.2477915199073,36.3396876255291,36.4317309974756,
36.499559550902,36.5916183825352,36.683557146995,36.7754022221935,36.8671829220369,
36.9589302993224,37.0506680600512,37.1424198962478,37.2342663270164,37.32616245876,
37.4182058559552,37.4860341333588,37.5780930392207,37.6700318784838,37.7618770289539,
37.8536578044556,37.9454052576079,38.0371430943186,38.1288950065193,38.2207415128571,
38.3126377200377,38.4046811916876,38.4725087158156,38.5645673417354,38.6565059006634,
38.7483507707782,38.8401312670426,38.9318784417468,39.0236160011304,39.1153676374572,
39.2072138718485,39.2991098088712,39.3911530160044,39.4589832982724,39.5510422449303,
39.6429811231728,39.7348263107813,39.8266071205372,39.9183546061647,40.0100924735443,
40.1018444145791,40.1936909467628,40.2855871781657,40.37763067117,40.4454578807292,
40.5375172362535,40.6294565280628,40.7213021333286,40.8130833651009,40.9048312752559,
40.9965695691435,41.0883219381371,41.1801688978633,41.2720655571968,41.3641094743968,
41.431932463186,41.481273340989),.UNSPECIFIED.);
#1336=B_SPLINE_CURVE_WITH_KNOTS('',3,(#10318,#10319,#10320,#10321,#10322,
#10323,#10324,#10325,#10326,#10327,#10328,#10329,#10330,#10331,#10332,#10333,
#10334,#10335,#10336,#10337,#10338,#10339,#10340,#10341,#10342,#10343,#10344,
#10345,#10346,#10347,#10348,#10349,#10350,#10351,#10352,#10353,#10354,#10355,
#10356,#10357,#10358,#10359,#10360,#10361,#10362,#10363,#10364,#10365,#10366,
#10367,#10368,#10369,#10370,#10371,#10372,#10373,#10374,#10375,#10376,#10377,
#10378,#10379,#10380,#10381,#10382,#10383,#10384,#10385,#10386,#10387,#10388,
#10389,#10390,#10391,#10392,#10393,#10394,#10395,#10396,#10397,#10398,#10399,
#10400,#10401,#10402,#10403,#10404,#10405,#10406,#10407,#10408,#10409,#10410,
#10411,#10412,#10413,#10414,#10415,#10416,#10417,#10418,#10419,#10420,#10421,
#10422,#10423,#10424,#10425,#10426,#10427,#10428,#10429,#10430,#10431,#10432,
#10433,#10434,#10435,#10436,#10437,#10438,#10439,#10440,#10441,#10442,#10443,
#10444,#10445,#10446,#10447,#10448,#10449,#10450,#10451,#10452,#10453,#10454,
#10455,#10456,#10457,#10458,#10459,#10460,#10461,#10462,#10463,#10464,#10465,
#10466,#10467,#10468,#10469,#10470,#10471,#10472,#10473,#10474,#10475,#10476,
#10477,#10478,#10479,#10480,#10481,#10482,#10483,#10484,#10485,#10486,#10487,
#10488,#10489,#10490,#10491,#10492,#10493,#10494,#10495,#10496,#10497,#10498,
#10499,#10500,#10501,#10502,#10503,#10504,#10505,#10506,#10507,#10508,#10509,
#10510,#10511,#10512,#10513,#10514,#10515,#10516,#10517,#10518,#10519,#10520,
#10521,#10522,#10523,#10524,#10525,#10526,#10527,#10528),.UNSPECIFIED.,
 .F.,.F.,(4,3,3,3,3,3,3,3,3,3,3,3,3,3,3,3,3,3,3,3,3,3,3,3,3,3,3,3,3,3,3,
3,3,3,3,3,3,3,3,3,3,3,3,3,3,3,3,3,3,3,3,3,3,3,3,3,3,3,3,3,3,3,3,3,3,3,3,
3,3,3,4),(-37.7402431363199,-37.6296257451957,-37.5178108639187,-37.4860341333588,
-37.3939753040707,-37.3020365414895,-37.210191467705,-37.1184107685739,
-37.0266633915695,-36.9349256306911,-36.8431737939141,-36.7513273619022,
-36.6594312285449,-36.5673878291486,-36.4995595509019,-36.4075007467294,
-36.3155620098938,-36.2237169624464,-36.1319362904343,-36.0401889410196,
-35.9484512081691,-35.8566993998259,-35.7648529967065,-35.6729568925387,
-35.580913522525,-35.5130849684451,-35.4210261316512,-35.3290873616942,
-35.2372422806735,-35.1454615745483,-35.0537141907017,-34.9619764231418,
-34.8702245798533,-34.7783781416357,-34.6864820022339,-34.5944385971196,
-34.5266103859883,-34.4345515609237,-34.3426128028142,-34.2507677337424,
-34.1589870396681,-34.0672396679303,-33.9755019125228,-33.883750081415,
-33.7919036553475,-33.7000075280963,-33.6079641350102,-33.5401358035315,
-33.448076980176,-33.3561382238359,-33.2642931565909,-33.1725124644226,
-33.0807650946389,-32.989027341231,-32.8972755121666,-32.8054290881977,
-32.7135329630789,-32.6214895721594,-32.5536612210747,-32.4616023938271,
-32.369663633532,-32.2778185622746,-32.1860378660245,-32.0942904921179,
-32.0025527345512,-31.9108009012964,-31.8189544731144,-31.7270583437636,
-31.635014948624,-31.5671866386179,-31.4964407967228),.UNSPECIFIED.);
#1337=B_SPLINE_CURVE_WITH_KNOTS('',3,(#10529,#10530,#10531,#10532),
 .UNSPECIFIED.,.F.,.F.,(4,4),(-31.4964407964964,-31.4556278135382),
 .UNSPECIFIED.);
#1338=B_SPLINE_CURVE_WITH_KNOTS('',3,(#10537,#10538,#10539,#10540,#10541,
#10542,#10543,#10544,#10545,#10546,#10547,#10548,#10549,#10550,#10551,#10552,
#10553,#10554,#10555,#10556,#10557,#10558,#10559,#10560,#10561,#10562,#10563,
#10564,#10565,#10566,#10567,#10568,#10569,#10570,#10571,#10572,#10573,#10574,
#10575,#10576,#10577,#10578,#10579,#10580,#10581,#10582,#10583,#10584,#10585,
#10586,#10587,#10588,#10589,#10590,#10591,#10592,#10593,#10594,#10595,#10596,
#10597,#10598,#10599,#10600,#10601,#10602,#10603,#10604,#10605,#10606,#10607,
#10608,#10609,#10610,#10611,#10612,#10613,#10614,#10615,#10616,#10617,#10618,
#10619,#10620,#10621,#10622,#10623,#10624,#10625,#10626,#10627,#10628,#10629,
#10630,#10631,#10632,#10633,#10634,#10635,#10636,#10637,#10638,#10639,#10640,
#10641,#10642,#10643,#10644,#10645,#10646,#10647,#10648,#10649,#10650,#10651,
#10652,#10653,#10654,#10655,#10656,#10657,#10658,#10659,#10660,#10661,#10662,
#10663,#10664,#10665,#10666,#10667,#10668,#10669,#10670,#10671,#10672,#10673,
#10674,#10675,#10676,#10677,#10678,#10679,#10680,#10681,#10682,#10683,#10684,
#10685,#10686,#10687,#10688,#10689,#10690,#10691,#10692,#10693,#10694,#10695,
#10696,#10697,#10698,#10699,#10700,#10701,#10702,#10703,#10704,#10705,#10706,
#10707,#10708),.UNSPECIFIED.,.F.,.F.,(4,2,2,2,2,2,2,2,2,2,2,2,2,2,2,2,2,
2,2,2,2,2,2,2,2,2,2,2,2,2,2,2,2,2,2,2,2,2,2,2,2,2,2,2,2,2,2,2,2,2,2,2,2,
2,2,2,2,2,2,2,2,2,2,2,2,2,2,2,2,2,2,2,2,2,2,2,2,2,2,2,2,2,2,2,2,4),(-2.14953858586417,
-2.13610813898098,-2.10687093381457,-2.0935221044845,-2.0831254479754,-2.07149231131417,
-2.05102003132299,-2.00904126853951,-1.93718251534886,-1.92579729579304,
-1.91931651355889,-1.91321297044488,-1.90366780511875,-1.86670492808403,
-1.78240676041869,-1.76404857092553,-1.75282287879321,-1.74230005870951,
-1.72778442760372,-1.68692585622836,-1.64388492520681,-1.60272463552078,
-1.59094892501349,-1.58438844302371,-1.57833165355395,-1.56903538001366,
-1.53604613636689,-1.48940831177372,-1.44101759357861,-1.4257294457842,
-1.4151857264115,-1.40421607879289,-1.38718524602246,-1.33908552311463,
-1.26676466619605,-1.25545930392889,-1.24899494598056,-1.24288080222962,
-1.23328057998228,-1.19528505603487,-1.10808253925909,-1.09174994054149,
-1.08091235409407,-1.07013932885364,-1.05415624803017,-1.03536586910847,
-0.995752605398778,-0.930612136396024,-0.919842288811208,-0.913489215146185,
-0.907293604969757,-0.897281569532202,-0.846083643004777,-0.774843892541429,
-0.757586723106827,-0.746574089308113,-0.735937662077742,-0.720723346769414,
-0.67056321977808,-0.599313589175422,-0.586315801481275,-0.579511648957109,
-0.573555967702531,-0.564864394134943,-0.538903563574624,-0.484576057882175,
-0.435577041749676,-0.420270860093574,-0.409724031026593,-0.398758819190083,
-0.381751445361605,-0.361316527916232,-0.314989293643927,-0.261991215016622,
-0.25031083845285,-0.243769640704525,-0.237702029212099,-0.228347600828176,
-0.194514321580064,-0.106632668467665,-0.0883038156412996,-0.0770840502604572,
-0.0665590960501105,-0.0561515529498116,-0.0359226655579419,-0.01489375026152),
 .UNSPECIFIED.);
#1339=B_SPLINE_CURVE_WITH_KNOTS('',3,(#10710,#10711,#10712,#10713,#10714,
#10715,#10716,#10717,#10718,#10719,#10720,#10721,#10722,#10723,#10724,#10725,
#10726,#10727,#10728,#10729,#10730,#10731,#10732,#10733,#10734,#10735,#10736,
#10737,#10738,#10739,#10740,#10741,#10742,#10743,#10744,#10745,#10746,#10747,
#10748,#10749,#10750,#10751,#10752,#10753,#10754,#10755,#10756,#10757,#10758,
#10759,#10760,#10761,#10762,#10763,#10764,#10765,#10766,#10767,#10768,#10769,
#10770,#10771,#10772,#10773,#10774,#10775,#10776,#10777,#10778,#10779,#10780,
#10781,#10782,#10783,#10784,#10785,#10786,#10787,#10788,#10789,#10790,#10791,
#10792,#10793,#10794,#10795,#10796,#10797,#10798,#10799,#10800,#10801,#10802,
#10803,#10804,#10805,#10806,#10807,#10808,#10809,#10810,#10811,#10812,#10813,
#10814,#10815,#10816,#10817,#10818,#10819,#10820,#10821,#10822,#10823,#10824,
#10825,#10826,#10827,#10828,#10829,#10830,#10831,#10832,#10833,#10834,#10835,
#10836,#10837,#10838,#10839,#10840,#10841,#10842,#10843,#10844,#10845,#10846,
#10847,#10848,#10849,#10850,#10851,#10852,#10853,#10854,#10855,#10856,#10857,
#10858,#10859,#10860,#10861,#10862,#10863,#10864,#10865,#10866,#10867,#10868,
#10869,#10870,#10871,#10872,#10873,#10874,#10875,#10876,#10877,#10878,#10879,
#10880,#10881,#10882,#10883,#10884,#10885,#10886,#10887,#10888,#10889,#10890,
#10891,#10892,#10893,#10894,#10895,#10896,#10897,#10898,#10899,#10900,#10901,
#10902,#10903,#10904,#10905,#10906,#10907,#10908,#10909,#10910,#10911,#10912,
#10913,#10914,#10915,#10916,#10917,#10918,#10919,#10920),.UNSPECIFIED.,
 .F.,.F.,(4,3,3,3,3,3,3,3,3,3,3,3,3,3,3,3,3,3,3,3,3,3,3,3,3,3,3,3,3,3,3,
3,3,3,3,3,3,3,3,3,3,3,3,3,3,3,3,3,3,3,3,3,3,3,3,3,3,3,3,3,3,3,3,3,3,3,3,
3,3,3,4),(-31.4556278135382,-31.3645591435807,-31.2735913846309,-31.1826963684724,
-31.0918391897302,-31.000995169334,-30.9101396451473,-30.8191934310805,
-30.7281979935595,-30.6370606348414,-30.5807120561611,-30.4886532306627,
-30.3967144721414,-30.3048694026802,-30.2130887082518,-30.121341336182,
-30.0296035804647,-29.9378517490699,-29.8460053227535,-29.7541091952737,
-29.6620658019955,-29.5942374737043,-29.5021786477549,-29.410239888775,
-29.3183948188481,-29.2266141239454,-29.134866751396,-29.0431289951948,
-28.9513771633125,-28.8595307365047,-28.7676346085315,-28.6755912147604,
-28.6077628912475,-28.5157040655444,-28.4237653068137,-28.3319202371385,
-28.2401395424906,-28.1483921701978,-28.0566544142547,-27.9649025826313,
-27.8730561560826,-27.7811600283684,-27.6891166348549,-27.6212883087907,
-27.529229483072,-27.4372907243261,-27.3454456546361,-27.2536649599738,
-27.1619175876671,-27.0701798317099,-26.9784280000733,-26.8865815735122,
-26.7946854457863,-26.7026420522615,-26.6348137263339,-26.5427549005322,
-26.4508161417019,-26.3589710719269,-26.2671903771789,-26.1754430047856,
-26.0837052487418,-25.9919534170181,-25.9001069903698,-25.8082108625567,
-25.7161674689453,-25.6483391438771,-25.5487804941692,-25.4495593335883,
-25.3505537169068,-25.2518618478458,-25.2132554897648),.UNSPECIFIED.);
#1340=B_SPLINE_CURVE_WITH_KNOTS('',3,(#10921,#10922,#10923,#10924),
 .UNSPECIFIED.,.F.,.F.,(4,4),(-25.2132554895433,-25.1729131975202),
 .UNSPECIFIED.);
#1341=B_SPLINE_CURVE_WITH_KNOTS('',3,(#10930,#10931,#10932,#10933,#10934,
#10935,#10936,#10937),.UNSPECIFIED.,.F.,.F.,(4,2,2,4),(-0.0146656910965199,
-0.0136853303791787,-0.00578768816179248,-0.000952400549440762),
 .UNSPECIFIED.);
#1342=B_SPLINE_CURVE_WITH_KNOTS('',3,(#10938,#10939,#10940,#10941,#10942,
#10943,#10944,#10945,#10946,#10947,#10948,#10949,#10950,#10951,#10952,#10953,
#10954,#10955,#10956,#10957,#10958,#10959,#10960,#10961,#10962,#10963,#10964,
#10965,#10966,#10967,#10968,#10969,#10970,#10971,#10972,#10973,#10974,#10975,
#10976,#10977,#10978,#10979,#10980,#10981,#10982,#10983,#10984,#10985,#10986,
#10987,#10988,#10989,#10990,#10991,#10992,#10993,#10994,#10995,#10996,#10997,
#10998,#10999,#11000,#11001,#11002,#11003,#11004,#11005,#11006,#11007,#11008,
#11009,#11010,#11011,#11012,#11013,#11014,#11015,#11016,#11017,#11018,#11019,
#11020,#11021,#11022,#11023,#11024,#11025,#11026,#11027,#11028,#11029,#11030,
#11031,#11032,#11033,#11034,#11035,#11036,#11037,#11038,#11039,#11040,#11041,
#11042,#11043,#11044,#11045,#11046,#11047,#11048,#11049,#11050,#11051,#11052,
#11053,#11054,#11055,#11056,#11057,#11058,#11059,#11060,#11061,#11062,#11063,
#11064,#11065,#11066,#11067,#11068,#11069,#11070,#11071,#11072,#11073,#11074,
#11075,#11076,#11077,#11078,#11079,#11080,#11081,#11082,#11083,#11084,#11085,
#11086,#11087,#11088,#11089,#11090,#11091,#11092,#11093,#11094,#11095,#11096,
#11097,#11098,#11099,#11100,#11101,#11102,#11103,#11104,#11105),
 .UNSPECIFIED.,.F.,.F.,(4,2,2,2,2,2,2,2,2,2,2,2,2,2,2,2,2,2,2,2,2,2,2,2,
2,2,2,2,2,2,2,2,2,2,2,2,2,2,2,2,2,2,2,2,2,2,2,2,2,2,2,2,2,2,2,2,2,2,2,2,
2,2,2,2,2,2,2,2,2,2,2,2,2,2,2,2,2,2,2,2,2,2,2,4),(-4.27070740756644,-4.26845734415281,
-4.26513559133958,-4.25906606303054,-4.24952699657373,-4.21011345994702,
-4.16915985939891,-4.12180760711633,-4.10676704011442,-4.09615910290225,
-4.08509740221113,-4.06758940933802,-3.99910328784442,-3.9458945201856,
-3.93578396964048,-3.9295677886981,-3.9240191638012,-3.91420944433972,-3.87342317107289,
-3.79628390799866,-3.77640623229577,-3.76488647469895,-3.75446318749615,
-3.74089878878225,-3.71027019002783,-3.69362884610084,-3.61789986526809,
-3.60359714260818,-3.59654526967702,-3.59064853248447,-3.58241197101851,
-3.5666807665863,-3.50044895582588,-3.45166143435875,-3.43652726145964,
-3.42590371268601,-3.4161810895516,-3.40005101277712,-3.31189369827086,
-3.27441517997453,-3.26484243659632,-3.25873327803455,-3.25226026131045,
-3.24091380528961,-3.18231134609231,-3.11799245657953,-3.10215500393181,
-3.09140788170318,-3.08053988233276,-3.06404741549002,-2.97767954176669,
-2.9392793607554,-2.92965905691019,-2.92354073671627,-2.91708181879243,
-2.90580370886008,-2.83327143510972,-2.78524170933674,-2.76822013775899,
-2.75725201681171,-2.74670681015199,-2.73141094379886,-2.68269075238979,
-2.63636231039439,-2.60346383850845,-2.5941744648963,-2.58811880042586,
-2.58155582225467,-2.56976801339054,-2.52829661670641,-2.47414699093332,
-2.44211003703892,-2.42859143623981,-2.41820155744132,-2.40653635310401,
-2.38644804475334,-2.30015407711382,-2.26816090375457,-2.25893700769353,
-2.2528930562116,-2.24630694500189,-2.23440577610699,-2.18385852421173,
-2.14953858586417),.UNSPECIFIED.);
#1343=B_SPLINE_CURVE_WITH_KNOTS('',3,(#11107,#11108,#11109,#11110,#11111,
#11112,#11113,#11114,#11115,#11116,#11117,#11118,#11119,#11120,#11121,#11122,
#11123,#11124,#11125,#11126,#11127,#11128,#11129,#11130,#11131,#11132,#11133,
#11134,#11135,#11136,#11137,#11138,#11139,#11140,#11141,#11142,#11143,#11144,
#11145,#11146,#11147,#11148,#11149,#11150,#11151,#11152,#11153,#11154,#11155,
#11156,#11157,#11158,#11159,#11160,#11161,#11162,#11163,#11164,#11165,#11166,
#11167,#11168,#11169,#11170,#11171,#11172,#11173,#11174,#11175,#11176,#11177,
#11178,#11179,#11180,#11181,#11182,#11183,#11184,#11185,#11186,#11187,#11188,
#11189,#11190,#11191,#11192,#11193,#11194,#11195,#11196,#11197,#11198,#11199,
#11200,#11201,#11202,#11203,#11204,#11205,#11206,#11207,#11208,#11209,#11210,
#11211,#11212,#11213,#11214,#11215,#11216,#11217,#11218,#11219,#11220,#11221,
#11222,#11223,#11224,#11225,#11226,#11227,#11228,#11229,#11230,#11231,#11232,
#11233,#11234,#11235,#11236,#11237,#11238,#11239,#11240,#11241,#11242,#11243,
#11244,#11245,#11246,#11247,#11248,#11249,#11250,#11251,#11252,#11253,#11254,
#11255,#11256,#11257,#11258,#11259,#11260,#11261,#11262,#11263,#11264,#11265,
#11266,#11267,#11268,#11269,#11270,#11271,#11272,#11273,#11274,#11275,#11276,
#11277,#11278,#11279,#11280,#11281,#11282,#11283,#11284,#11285,#11286,#11287,
#11288,#11289,#11290,#11291,#11292,#11293,#11294,#11295,#11296,#11297,#11298,
#11299,#11300,#11301,#11302,#11303,#11304,#11305,#11306,#11307,#11308,#11309,
#11310,#11311,#11312,#11313,#11314,#11315,#11316,#11317),.UNSPECIFIED.,
 .F.,.F.,(4,3,3,3,3,3,3,3,3,3,3,3,3,3,3,3,3,3,3,3,3,3,3,3,3,3,3,3,3,3,3,
3,3,3,3,3,3,3,3,3,3,3,3,3,3,3,3,3,3,3,3,3,3,3,3,3,3,3,3,3,3,3,3,3,3,3,3,
3,3,3,4),(-25.1729131975202,-25.0788738378323,-24.9847644203176,-24.8904963173327,
-24.7961392500284,-24.7016048176209,-24.6618645614202,-24.5698057357159,
-24.4778669769843,-24.3860219073086,-24.2942412126603,-24.2024938403674,
-24.1107560844241,-24.0190042528011,-23.9271578262531,-23.8352616985401,
-23.7432183050277,-23.6753899789634,-23.5833311530027,-23.4913923940134,
-23.3995473240798,-23.3077666291737,-23.2160192566231,-23.1242815004226,
-23.032529668543,-22.9406832417416,-22.8487871137763,-22.7567437200162,
-22.6889153965066,-22.5968565710371,-22.5049178125391,-22.413072743095,
-22.3212920486752,-22.2295446766086,-22.1378069208892,-22.046055089487,
-21.9542086631547,-21.8623125356545,-21.7702691423485,-21.7024408140498,
-21.6103819885079,-21.5184432299415,-21.426598160434,-21.3348174659573,
-21.243070093838,-21.1513323380701,-21.0595805066238,-20.9677340802541,
-20.8758379527205,-20.7837945593873,-20.715966231593,-20.6239074042684,
-20.5319686439116,-20.4401235726081,-20.3483428763351,-20.2565955024199,
-20.1648577448588,-20.0731059116239,-19.9812594834839,-19.8893633541873,
-19.7973199591215,-19.7294916491362,-19.6387533739174,-19.5481571350446,
-19.4576413869019,-19.3671810154049,-19.276750966138,-19.1862889103547,
-19.0958131870846,-19.0052388477835,-18.930070182607),.UNSPECIFIED.);
#1344=B_SPLINE_CURVE_WITH_KNOTS('',3,(#11318,#11319,#11320,#11321),
 .UNSPECIFIED.,.F.,.F.,(4,4),(-18.9300701823637,-18.8905536429109),
 .UNSPECIFIED.);
#1345=B_SPLINE_CURVE_WITH_KNOTS('',3,(#11326,#11327,#11328,#11329,#11330,
#11331,#11332,#11333,#11334,#11335,#11336,#11337,#11338,#11339,#11340,#11341,
#11342,#11343,#11344,#11345,#11346,#11347,#11348,#11349,#11350,#11351,#11352,
#11353,#11354,#11355,#11356,#11357,#11358,#11359,#11360,#11361,#11362,#11363,
#11364,#11365,#11366,#11367,#11368,#11369,#11370,#11371,#11372,#11373,#11374,
#11375,#11376,#11377,#11378,#11379,#11380,#11381,#11382,#11383,#11384,#11385,
#11386,#11387,#11388,#11389,#11390,#11391,#11392,#11393,#11394,#11395,#11396,
#11397,#11398,#11399,#11400,#11401,#11402,#11403,#11404,#11405,#11406,#11407,
#11408,#11409,#11410,#11411,#11412,#11413,#11414,#11415,#11416,#11417,#11418,
#11419,#11420,#11421,#11422,#11423,#11424,#11425,#11426,#11427,#11428,#11429,
#11430,#11431,#11432,#11433,#11434,#11435,#11436,#11437,#11438,#11439,#11440,
#11441,#11442,#11443,#11444,#11445,#11446,#11447,#11448,#11449,#11450,#11451,
#11452,#11453,#11454,#11455,#11456,#11457,#11458,#11459,#11460,#11461,#11462,
#11463,#11464,#11465,#11466,#11467,#11468,#11469,#11470,#11471,#11472,#11473,
#11474,#11475,#11476,#11477,#11478,#11479,#11480,#11481,#11482,#11483,#11484,
#11485),.UNSPECIFIED.,.F.,.F.,(4,2,2,2,2,2,2,2,2,2,2,2,2,2,2,2,2,2,2,2,
2,2,2,2,2,2,2,2,2,2,2,2,2,2,2,2,2,2,2,2,2,2,2,2,2,2,2,2,2,2,2,2,2,2,2,2,
2,2,2,2,2,2,2,2,2,2,2,2,2,2,2,2,2,2,2,2,2,2,2,4),(-2.14929610429856,-2.13546420060753,
-2.05952257959691,-2.02135630128187,-2.01163747150297,-2.00610532855159,
-1.99986862416345,-1.98965703996022,-1.93689921034541,-1.86805261034334,
-1.85056925677954,-1.83951280409052,-1.82890296846166,-1.81384752281798,
-1.76624363582999,-1.70408844889312,-1.68313484161148,-1.67484391041751,
-1.66894143595695,-1.6619238153601,-1.64780429759842,-1.57828901672924,
-1.5283911789661,-1.51306292788187,-1.50251304115817,-1.49155461978892,
-1.47457925945926,-1.41954608868631,-1.35272459954898,-1.34215288669531,
-1.33584132096922,-1.32961008093004,-1.31942331018782,-1.30672559706725,
-1.27796607365477,-1.19950440879412,-1.18112791310739,-1.16989924299949,
-1.15937887655559,-1.14487520442654,-1.10413562971075,-1.06124090532109,
-1.01981336371654,-1.00802996324934,-1.00146822761214,-0.995412816490563,
-0.986122322518482,-0.953207721022963,-0.906835969948993,-0.858125564142618,
-0.84282877879844,-0.832284183874897,-0.821317806699372,-0.804301090105841,
-0.756295628946055,-0.683810467133665,-0.672535405490896,-0.666077605267117,
-0.659959925147,-0.650339754463948,-0.611939939149989,-0.525525154332974,
-0.509036470323033,-0.498170260114691,-0.487424478073313,-0.471588035855322,
-0.40707434501598,-0.348776340856676,-0.337419925706362,-0.330945468836147,
-0.324838891291911,-0.315275743896004,-0.277969583990255,-0.191934540819767,
-0.174670707009472,-0.163657356711335,-0.153022693458767,-0.137815258590444,
-0.0877584016624937,-0.0146656910965199),.UNSPECIFIED.);
#1346=B_SPLINE_CURVE_WITH_KNOTS('',3,(#11487,#11488,#11489,#11490,#11491,
#11492,#11493,#11494,#11495,#11496,#11497,#11498,#11499,#11500,#11501,#11502,
#11503,#11504,#11505,#11506,#11507,#11508,#11509,#11510,#11511,#11512,#11513,
#11514,#11515,#11516,#11517,#11518,#11519,#11520,#11521,#11522,#11523,#11524,
#11525,#11526,#11527,#11528,#11529,#11530,#11531,#11532,#11533,#11534,#11535,
#11536,#11537,#11538,#11539,#11540,#11541,#11542,#11543,#11544,#11545,#11546,
#11547,#11548,#11549,#11550,#11551,#11552,#11553,#11554,#11555,#11556,#11557,
#11558,#11559,#11560,#11561,#11562,#11563,#11564,#11565,#11566,#11567,#11568,
#11569,#11570,#11571,#11572,#11573,#11574,#11575,#11576,#11577,#11578,#11579,
#11580,#11581,#11582,#11583,#11584,#11585,#11586,#11587,#11588,#11589,#11590,
#11591,#11592,#11593,#11594,#11595,#11596,#11597,#11598,#11599,#11600,#11601,
#11602,#11603,#11604,#11605,#11606,#11607,#11608,#11609,#11610,#11611,#11612,
#11613,#11614,#11615,#11616,#11617,#11618,#11619,#11620,#11621,#11622,#11623,
#11624,#11625,#11626,#11627,#11628,#11629,#11630,#11631,#11632,#11633,#11634,
#11635,#11636,#11637,#11638,#11639,#11640,#11641,#11642,#11643,#11644,#11645,
#11646,#11647,#11648,#11649,#11650,#11651,#11652,#11653,#11654,#11655,#11656,
#11657,#11658,#11659,#11660,#11661,#11662,#11663,#11664,#11665,#11666,#11667,
#11668,#11669,#11670,#11671,#11672,#11673,#11674,#11675,#11676,#11677,#11678,
#11679,#11680,#11681,#11682,#11683,#11684,#11685,#11686,#11687,#11688,#11689,
#11690,#11691,#11692,#11693,#11694,#11695,#11696,#11697),.UNSPECIFIED.,
 .F.,.F.,(4,3,3,3,3,3,3,3,3,3,3,3,3,3,3,3,3,3,3,3,3,3,3,3,3,3,3,3,3,3,3,
3,3,3,3,3,3,3,3,3,3,3,3,3,3,3,3,3,3,3,3,3,3,3,3,3,3,3,3,3,3,3,3,3,3,3,3,
3,3,3,4),(-18.8905536429109,-18.7557293146775,-18.7430170666794,-18.6509582413954,
-18.5590194831107,-18.4671744139074,-18.375393719768,-18.2836463480059,
-18.1919085926147,-18.1001567615639,-18.008310335616,-17.9164142085194,
-17.8243708156434,-17.7565424842226,-17.6644836469602,-17.5725448766289,
-17.4806997953276,-17.3889190890633,-17.2971717051645,-17.2054339376393,
-17.1136820944725,-17.0218356565102,-16.9299395174383,-16.8378961127723,
-16.7700679017658,-16.6780090994978,-16.5860703641842,-16.4942253178778,
-16.4024446464311,-16.3106972972283,-16.2189595642365,-16.1272077553988,
-16.0353613512415,-15.9434652457323,-15.8514218738956,-15.783593319309,
-15.6915344876934,-15.5995957232524,-15.5077506480737,-15.4159699482515,
-15.3242225709882,-15.2324848102825,-15.1407329741097,-15.0488865433661,
-14.9569904116482,-14.8649470144796,-14.7971187368521,-14.705059830534,
-14.6131209908129,-14.5212758398835,-14.4294950639227,-14.3377476103115,
-14.2460097731428,-14.1542578604853,-14.0624113536955,-13.970515146065,
-13.8784716739733,-13.8106441543953,-13.7185855293363,-13.6266469712689,
-13.5348021020134,-13.443021606603,-13.3512744327491,-13.2595368742113,
-13.1677852387247,-13.0759390051598,-12.984043068957,-12.8919998626249,
-12.8241695719385,-12.6868365123048,-12.6468848751841),.UNSPECIFIED.);
#1347=B_SPLINE_CURVE_WITH_KNOTS('',3,(#11698,#11699,#11700,#11701),
 .UNSPECIFIED.,.F.,.F.,(4,4),(-12.646880067867,-12.605793069694),
 .UNSPECIFIED.);
#1348=B_SPLINE_CURVE_WITH_KNOTS('',3,(#11707,#11708,#11709,#11710),
 .UNSPECIFIED.,.F.,.F.,(4,4),(-0.0143336373215858,-0.000956395227510613),
 .UNSPECIFIED.);
#1349=B_SPLINE_CURVE_WITH_KNOTS('',3,(#11711,#11712,#11713,#11714,#11715,
#11716,#11717,#11718,#11719,#11720,#11721,#11722,#11723,#11724,#11725,#11726,
#11727,#11728,#11729,#11730,#11731,#11732,#11733,#11734,#11735,#11736,#11737,
#11738,#11739,#11740,#11741,#11742,#11743,#11744,#11745,#11746,#11747,#11748,
#11749,#11750,#11751,#11752,#11753,#11754,#11755,#11756,#11757,#11758,#11759,
#11760,#11761,#11762,#11763,#11764,#11765,#11766,#11767,#11768,#11769,#11770,
#11771,#11772,#11773,#11774,#11775,#11776,#11777,#11778,#11779,#11780,#11781,
#11782,#11783,#11784,#11785,#11786,#11787,#11788,#11789,#11790,#11791,#11792,
#11793,#11794,#11795,#11796,#11797,#11798,#11799,#11800,#11801,#11802,#11803,
#11804,#11805,#11806,#11807,#11808,#11809,#11810,#11811,#11812,#11813,#11814,
#11815,#11816,#11817,#11818,#11819,#11820,#11821,#11822,#11823,#11824,#11825,
#11826,#11827,#11828,#11829,#11830,#11831,#11832,#11833,#11834,#11835,#11836,
#11837,#11838,#11839,#11840,#11841,#11842,#11843,#11844,#11845,#11846,#11847,
#11848,#11849,#11850,#11851,#11852,#11853,#11854,#11855,#11856,#11857,#11858,
#11859,#11860,#11861,#11862,#11863,#11864,#11865,#11866,#11867,#11868,#11869,
#11870,#11871,#11872,#11873,#11874,#11875,#11876),.UNSPECIFIED.,.F.,.F.,
(4,2,2,2,2,2,2,2,2,2,2,2,2,2,2,2,2,2,2,2,2,2,2,2,2,2,2,2,2,2,2,2,2,2,2,
2,2,2,2,2,2,2,2,2,2,2,2,2,2,2,2,2,2,2,2,2,2,2,2,2,2,2,2,2,2,2,2,2,2,2,2,
2,2,2,2,2,2,2,2,2,2,2,4),(-4.27075566588217,-4.22829678691838,-4.20716660973916,
-4.19293595591049,-4.18245536031667,-4.17112333488929,-4.15221716328105,
-4.06868544790909,-4.03199788215742,-4.02246865308842,-4.0163680373765,
-4.00988188810468,-3.99847231363553,-3.92669569261786,-3.87825848541359,
-3.8611788431039,-3.8501991667344,-3.83966060812061,-3.82440676220799,-3.77698114903899,
-3.72959533825348,-3.69640951053994,-3.68709961168663,-3.68103990998908,
-3.67448343916799,-3.66272817673599,-3.59300078740973,-3.53954516752815,
-3.52415797255716,-3.51349170215524,-3.50252321294966,-3.48549619727635,
-3.40186688966681,-3.37473034606797,-3.357250251695,-3.34965453134102,-3.3437982546825,
-3.33624589446818,-3.31970212565846,-3.25279360715997,-3.20381711487164,
-3.18867215516095,-3.17804747178415,-3.16701625163083,-3.14966237173264,
-3.06775066371959,-3.03995088258877,-3.02219342779498,-3.01455398168473,
-3.00869716189578,-3.00118673040566,-2.98423878097789,-2.91755043422619,
-2.86863582116899,-2.85349447367274,-2.84287021075578,-2.83183763790963,
-2.81447766485955,-2.73259719480224,-2.6917318137603,-2.68199898243569,
-2.67585903222826,-2.66943293761237,-2.65831194878752,-2.59624265451598,
-2.53553574898416,-2.51945125413548,-2.50865972422484,-2.49784196283243,
-2.48161523124333,-2.39394462718287,-2.35622582513403,-2.34664103482908,
-2.34052992366097,-2.33406129785287,-2.32273445645158,-2.26364092558707,
-2.22082481112579,-2.19268930029812,-2.17973084959801,-2.16938969329131,
-2.15736609801839,-2.14929610429856),.UNSPECIFIED.);
#1350=B_SPLINE_CURVE_WITH_KNOTS('',3,(#11878,#11879,#11880,#11881,#11882,
#11883,#11884,#11885,#11886,#11887),.UNSPECIFIED.,.F.,.F.,(4,1,1,1,1,1,
1,4),(-12.605793069694,-11.8376949894817,-10.8512204070249,-9.86474582456809,
-8.87827124211129,-7.89179665965447,-6.90532207719767,-6.36369956800449),
 .UNSPECIFIED.);
#1351=B_SPLINE_CURVE_WITH_KNOTS('',3,(#11888,#11889,#11890,#11891),
 .UNSPECIFIED.,.F.,.F.,(4,4),(-6.36369956800449,-6.32388523350727),
 .UNSPECIFIED.);
#1352=B_SPLINE_CURVE_WITH_KNOTS('',3,(#11900,#11901,#11902,#11903,#11904,
#11905,#11906,#11907,#11908,#11909,#11910,#11911,#11912,#11913,#11914,#11915,
#11916,#11917,#11918,#11919,#11920,#11921,#11922,#11923,#11924,#11925,#11926,
#11927,#11928,#11929,#11930,#11931,#11932,#11933,#11934,#11935,#11936,#11937,
#11938,#11939,#11940,#11941),.UNSPECIFIED.,.F.,.F.,(4,2,2,2,2,2,2,2,2,2,
2,2,2,2,2,2,2,2,2,2,4),(-2.74875994684861,-2.73680062346907,-2.66994582987793,
-2.61858205907705,-2.6031629846185,-2.59238489636777,-2.58254038544452,
-2.56622343375549,-2.49014672046941,-2.4448468966665,-2.43487891586894,
-2.42860085479822,-2.42208310613659,-2.41069541006536,-2.35241981652588,
-2.28811087525863,-2.27228734435194,-2.26150416905709,-2.25055972640412,
-2.23386405000636,-2.14915318645226),.UNSPECIFIED.);
#1353=B_SPLINE_CURVE_WITH_KNOTS('',3,(#11945,#11946,#11947,#11948,#11949,
#11950,#11951,#11952),.UNSPECIFIED.,.F.,.F.,(4,2,2,4),(-0.0136766484190329,
-0.0136650905131395,-0.00597929307771191,0.),.UNSPECIFIED.);
#1354=B_SPLINE_CURVE_WITH_KNOTS('',3,(#11955,#11956,#11957,#11958,#11959,
#11960,#11961,#11962,#11963,#11964,#11965,#11966,#11967,#11968,#11969,#11970,
#11971,#11972,#11973,#11974,#11975,#11976,#11977,#11978,#11979,#11980,#11981,
#11982,#11983,#11984,#11985,#11986,#11987,#11988,#11989,#11990,#11991,#11992,
#11993,#11994,#11995,#11996,#11997,#11998,#11999,#12000,#12001,#12002,#12003,
#12004,#12005,#12006,#12007,#12008,#12009,#12010,#12011,#12012,#12013,#12014,
#12015,#12016,#12017,#12018,#12019,#12020,#12021,#12022,#12023,#12024,#12025,
#12026,#12027,#12028,#12029,#12030,#12031,#12032,#12033,#12034,#12035,#12036,
#12037,#12038,#12039,#12040,#12041,#12042,#12043,#12044,#12045,#12046,#12047,
#12048,#12049,#12050,#12051,#12052,#12053,#12054,#12055,#12056,#12057,#12058,
#12059,#12060,#12061,#12062,#12063,#12064,#12065,#12066,#12067,#12068,#12069,
#12070,#12071,#12072,#12073,#12074,#12075,#12076,#12077,#12078,#12079,#12080,
#12081,#12082,#12083,#12084,#12085,#12086,#12087,#12088,#12089,#12090,#12091,
#12092,#12093,#12094,#12095,#12096,#12097,#12098,#12099,#12100,#12101,#12102,
#12103,#12104,#12105,#12106,#12107,#12108,#12109,#12110,#12111,#12112,#12113,
#12114,#12115,#12116,#12117,#12118,#12119,#12120,#12121,#12122,#12123,#12124,
#12125,#12126,#12127,#12128,#12129,#12130),.UNSPECIFIED.,.F.,.F.,(4,2,2,
2,2,2,2,2,2,2,2,2,2,2,2,2,2,2,2,2,2,2,2,2,2,2,2,2,2,2,2,2,2,2,2,2,2,2,2,
2,2,2,2,2,2,2,2,2,2,2,2,2,2,2,2,2,2,2,2,2,2,2,2,2,2,2,2,2,2,2,2,2,2,2,2,
2,2,2,2,2,2,2,2,2,2,2,2,4),(-2.14915318645226,-2.13977645196419,-2.1080230085618,
-2.09880088562358,-2.09275325065881,-2.08619301461964,-2.07432944046408,
-2.0300292253873,-1.98844183527612,-1.94900613152566,-1.93467381877651,
-1.92422632513365,-1.91303383787223,-1.89463127284146,-1.81011878904744,
-1.77302312501884,-1.7635031006812,-1.75742728330176,-1.75096223581443,
-1.73966073299329,-1.67978569541584,-1.61701600790134,-1.60094705824663,
-1.59014195292663,-1.57929034828942,-1.56296779956946,-1.48469862007157,
-1.44235556857053,-1.43053416799353,-1.42395101506027,-1.41795441653693,
-1.40870095239954,-1.37865652758475,-1.3747320458654,-1.28308794063715,
-1.2666199265708,-1.25575343244952,-1.24499674298735,-1.22912387208739,
-1.21051175727462,-1.17159093799611,-1.10488623403885,-1.09429026306603,
-1.0879733151939,-1.08175019409971,-1.0715936047182,-1.01834666410771,-0.949943627903787,
-0.932427970779454,-0.921370136937541,-0.910772556920358,-0.895759187861899,
-0.848708020265131,-0.806917382321201,-0.768059114382065,-0.75831517249119,
-0.752781020769279,-0.746551879382092,-0.736378438319912,-0.723703588450711,
-0.69503427209062,-0.616952807509691,-0.598284433783136,-0.586996233807493,
-0.576494503724389,-0.562136071312497,-0.522918651835135,-0.48100459936932,
-0.436903944879415,-0.425031998285458,-0.418450138009205,-0.412401545987218,
-0.403155310551825,-0.370872617388443,-0.284506134251647,-0.26461898844124,
-0.252994408223817,-0.242596629471047,-0.229004035373909,-0.196403462788172,
-0.140328709106667,-0.0979915958228728,-0.0881577625901853,-0.0826054945296962,
-0.0763967162790068,-0.066317535538703,-0.0537979154367359,-0.0143336373215858),
 .UNSPECIFIED.);
#1355=B_SPLINE_CURVE_WITH_KNOTS('',3,(#12132,#12133,#12134,#12135,#12136,
#12137,#12138,#12139,#12140,#12141,#12142,#12143,#12144,#12145,#12146,#12147,
#12148,#12149,#12150,#12151,#12152,#12153,#12154,#12155,#12156,#12157,#12158,
#12159,#12160,#12161,#12162,#12163,#12164,#12165,#12166,#12167,#12168,#12169,
#12170,#12171,#12172,#12173,#12174,#12175,#12176,#12177,#12178,#12179,#12180,
#12181,#12182,#12183,#12184,#12185,#12186,#12187,#12188,#12189,#12190,#12191,
#12192,#12193,#12194,#12195,#12196,#12197,#12198,#12199,#12200,#12201,#12202,
#12203,#12204,#12205,#12206,#12207,#12208,#12209,#12210,#12211,#12212,#12213,
#12214,#12215,#12216,#12217,#12218,#12219,#12220,#12221,#12222,#12223,#12224,
#12225,#12226,#12227,#12228,#12229,#12230,#12231,#12232,#12233,#12234,#12235,
#12236,#12237,#12238,#12239,#12240,#12241,#12242,#12243,#12244,#12245,#12246,
#12247,#12248,#12249,#12250,#12251,#12252,#12253,#12254,#12255,#12256,#12257,
#12258,#12259,#12260,#12261,#12262,#12263,#12264,#12265,#12266,#12267,#12268,
#12269,#12270,#12271,#12272,#12273,#12274,#12275,#12276,#12277,#12278,#12279,
#12280,#12281,#12282,#12283,#12284,#12285,#12286,#12287,#12288,#12289,#12290,
#12291,#12292,#12293,#12294,#12295,#12296,#12297,#12298,#12299,#12300,#12301,
#12302,#12303,#12304,#12305,#12306,#12307,#12308,#12309,#12310,#12311,#12312,
#12313,#12314,#12315,#12316,#12317,#12318,#12319,#12320,#12321,#12322,#12323,
#12324,#12325,#12326,#12327,#12328,#12329,#12330,#12331,#12332,#12333,#12334,
#12335,#12336,#12337,#12338,#12339),.UNSPECIFIED.,.F.,.F.,(4,3,3,3,3,3,
3,3,3,3,3,3,3,3,3,3,3,3,3,3,3,3,3,3,3,3,3,3,3,3,3,3,3,3,3,3,3,3,3,3,3,3,
3,3,3,3,3,3,3,3,3,3,3,3,3,3,3,3,3,3,3,3,3,3,3,3,3,3,3,4),(-6.32388523350727,
-6.22262579881566,-6.12405219125192,-6.02144984299638,-5.91884749474085,
-5.82677170021766,-5.73481575008188,-5.64295329224136,-5.55115498883091,
-5.45938987934615,-5.36763428019483,-5.27586452167952,-5.18400015070594,
-5.09208604288732,-5.00002479493562,-4.93237291228405,-4.84041538501824,
-4.74857815709913,-4.65683471651366,-4.56515538493322,-4.47350917728831,
-4.38187226863628,-4.29022084773689,-4.19847354646315,-4.10667597603899,
-4.01472921555433,-3.94589832982724,-3.85368314282726,-3.76158838577229,
-3.66958788472042,-3.57765324610522,-3.48575290461766,-3.39386333766725,
-3.30196103757621,-3.20996713085427,-3.11792497754333,-3.02573938568974,
-2.95942374737043,-2.86729445288601,-2.77528351990613,-2.68336469320923,
-2.59150820388178,-2.49968381936634,-2.40786793835657,-2.3160369726511,
-2.22411036274905,-2.13213335341171,-2.04000878182278,-1.97294916491362,
-1.88173600258,-1.79064323262133,-1.69964346841178,-1.60870377166317,-1.51779459789241,
-1.42689135047595,-1.33596944318732,-1.24494083397421,-1.15385717271455,
-1.06260900446962,-0.986474582456811,-0.892933128223043,-0.799526737551554,
-0.706253524008857,-0.613057275991345,-0.519916434825251,-0.426809493840829,
-0.333687967356518,-0.240561825277099,-0.14736608189716,-0.0805142608249079),
 .UNSPECIFIED.);
#1356=B_SPLINE_CURVE_WITH_KNOTS('',3,(#12340,#12341,#12342,#12343),
 .UNSPECIFIED.,.F.,.F.,(4,4),(-0.0273304800634966,-0.0136766484190329),
 .UNSPECIFIED.);
#1357=B_SPLINE_CURVE_WITH_KNOTS('',3,(#12346,#12347,#12348,#12349,#12350,
#12351,#12352,#12353,#12354,#12355,#12356,#12357,#12358,#12359,#12360,#12361,
#12362,#12363,#12364,#12365,#12366,#12367,#12368,#12369,#12370,#12371,#12372,
#12373,#12374,#12375,#12376,#12377,#12378,#12379,#12380,#12381,#12382,#12383,
#12384,#12385,#12386,#12387,#12388,#12389,#12390,#12391,#12392,#12393,#12394,
#12395,#12396,#12397,#12398,#12399,#12400,#12401,#12402,#12403,#12404,#12405,
#12406,#12407,#12408,#12409,#12410,#12411,#12412,#12413,#12414,#12415,#12416,
#12417,#12418,#12419,#12420,#12421,#12422,#12423,#12424,#12425,#12426,#12427,
#12428,#12429,#12430,#12431,#12432,#12433,#12434,#12435,#12436,#12437,#12438,
#12439,#12440,#12441,#12442,#12443,#12444,#12445,#12446,#12447,#12448,#12449,
#12450,#12451,#12452,#12453,#12454,#12455,#12456,#12457,#12458,#12459,#12460,
#12461,#12462,#12463,#12464,#12465,#12466,#12467,#12468,#12469,#12470,#12471,
#12472,#12473,#12474,#12475,#12476,#12477,#12478,#12479,#12480,#12481,#12482,
#12483,#12484,#12485,#12486,#12487,#12488,#12489,#12490,#12491,#12492,#12493,
#12494,#12495,#12496,#12497,#12498,#12499,#12500,#12501,#12502,#12503,#12504,
#12505,#12506,#12507,#12508,#12509,#12510,#12511,#12512,#12513,#12514,#12515,
#12516,#12517,#12518,#12519,#12520,#12521,#12522,#12523,#12524,#12525,#12526,
#12527,#12528,#12529,#12530,#12531,#12532,#12533,#12534,#12535,#12536,#12537,
#12538,#12539,#12540,#12541),.UNSPECIFIED.,.F.,.F.,(4,3,3,3,3,3,3,3,3,3,
3,3,3,3,3,3,3,3,3,3,3,3,3,3,3,3,3,3,3,3,3,3,3,3,3,3,3,3,3,3,3,3,3,3,3,3,
3,3,3,3,3,3,3,3,3,3,3,3,3,3,3,3,3,3,3,4),(22.9601178369312,23.0476632051047,
23.135213307798,23.2227887574945,23.3104589160482,23.3981838672193,23.4860359984705,
23.5192456667785,23.6071124398246,23.6948693164178,23.7825392284102,23.8729368560134,
23.960509806113,24.0480702283888,24.1356387186068,24.2232358732018,24.3109292666562,
24.3986804063943,24.4865549881911,24.5057202492353,24.5935851740784,24.6813402090151,
24.769008288204,24.85940660614,24.9469777578932,25.0345363979054,25.1221031240315,
25.209698534809,25.2973902233545,25.3851396790604,25.4730126198469,25.4921948316921,
25.5800570260922,25.6678092807244,25.7554745334751,25.8458738935593,25.9334421221125,
26.0209978081109,26.1085615525769,26.1961539571956,26.2838426182611,26.3715890305608,
26.4594589274378,26.4786694141489,26.5665335826018,26.6542878372078,26.7419551132146,
26.8323537236385,26.9199240202891,27.0074817873822,27.0950476236647,27.1826421285534,
27.2703328919068,27.3580814100585,27.4459534022615,27.4651439966058,27.5517327508406,
27.6420578922587,27.7284382334182,27.8147667965675,27.9010653768991,27.9873557389373,
28.073693063983,28.160058275786,28.2465113806051,28.2743338821854),
 .UNSPECIFIED.);
#1358=B_SPLINE_CURVE_WITH_KNOTS('',3,(#12542,#12543,#12544,#12545,#12546,
#12547,#12548,#12549,#12550,#12551,#12552,#12553,#12554,#12555,#12556,#12557,
#12558,#12559,#12560,#12561,#12562,#12563,#12564,#12565,#12566,#12567,#12568,
#12569,#12570,#12571,#12572,#12573,#12574,#12575),.UNSPECIFIED.,.F.,.F.,
(4,3,3,3,3,3,3,3,3,3,3,4),(28.2743338823081,28.4054086201873,28.4516185790626,
28.5394941256643,28.6273758957033,28.7150344267578,28.8026345706311,28.8901969753923,
28.9782848030383,29.0658567392794,29.1542025126278,29.2425482859762),
 .UNSPECIFIED.);
#1359=B_SPLINE_CURVE_WITH_KNOTS('',3,(#12577,#12578,#12579,#12580,#12581,
#12582,#12583,#12584,#12585,#12586,#12587,#12588,#12589,#12590,#12591,#12592,
#12593,#12594,#12595,#12596,#12597,#12598,#12599,#12600,#12601,#12602,#12603,
#12604,#12605,#12606,#12607,#12608,#12609,#12610,#12611,#12612,#12613),
 .UNSPECIFIED.,.F.,.F.,(4,3,3,3,3,3,3,3,3,3,3,3,4),(28.2743338823081,28.3609594265871,
28.4475299266133,28.5340726431711,28.6206091569836,28.7071610397518,28.7938001360196,
28.8804868583994,28.9673043233213,29.0202572380501,29.1081269068421,29.1958739894493,
29.243664967692),.UNSPECIFIED.);
#1360=B_SPLINE_CURVE_WITH_KNOTS('',3,(#12614,#12615,#12616,#12617,#12618,
#12619,#12620,#12621,#12622,#12623,#12624,#12625,#12626,#12627,#12628,#12629,
#12630,#12631,#12632,#12633,#12634,#12635,#12636,#12637,#12638,#12639,#12640,
#12641,#12642,#12643,#12644,#12645,#12646,#12647,#12648,#12649,#12650,#12651,
#12652,#12653,#12654,#12655,#12656,#12657,#12658,#12659,#12660,#12661,#12662,
#12663,#12664,#12665,#12666,#12667,#12668,#12669,#12670,#12671,#12672,#12673,
#12674,#12675,#12676,#12677,#12678,#12679,#12680,#12681,#12682,#12683,#12684,
#12685,#12686,#12687,#12688,#12689,#12690,#12691,#12692,#12693,#12694,#12695,
#12696,#12697,#12698,#12699,#12700,#12701,#12702,#12703,#12704,#12705,#12706,
#12707,#12708,#12709,#12710,#12711,#12712,#12713,#12714,#12715,#12716,#12717,
#12718,#12719,#12720,#12721,#12722,#12723,#12724,#12725,#12726,#12727,#12728,
#12729,#12730,#12731,#12732,#12733,#12734,#12735,#12736,#12737,#12738,#12739,
#12740,#12741,#12742,#12743,#12744,#12745,#12746,#12747,#12748,#12749,#12750,
#12751,#12752,#12753,#12754,#12755,#12756,#12757,#12758,#12759,#12760,#12761,
#12762,#12763,#12764,#12765,#12766,#12767,#12768,#12769,#12770,#12771,#12772,
#12773,#12774,#12775,#12776,#12777,#12778,#12779,#12780,#12781,#12782,#12783,
#12784,#12785,#12786,#12787,#12788,#12789,#12790,#12791,#12792,#12793,#12794,
#12795,#12796,#12797,#12798,#12799,#12800,#12801,#12802,#12803,#12804,#12805,
#12806,#12807,#12808,#12809),.UNSPECIFIED.,.F.,.F.,(4,3,3,3,3,3,3,3,3,3,
3,3,3,3,3,3,3,3,3,3,3,3,3,3,3,3,3,3,3,3,3,3,3,3,3,3,3,3,3,3,3,3,3,3,3,3,
3,3,3,3,3,3,3,3,3,3,3,3,3,3,3,3,3,3,3,4),(22.959407626261,23.0471667563207,
23.1014097433092,23.1892903176247,23.2770610256841,23.364744781634,23.4551372246505,
23.5427239571801,23.6302981140569,23.7178802752913,23.8054910215075,23.8931978201871,
23.9809622710052,24.0688499272475,24.087884325766,24.1757616745349,24.2635293741877,
24.3512103418007,24.4416039126035,24.5291884271683,24.6167605827559,24.7043409627459,
24.7919501512936,24.8796557325264,24.9674191639839,25.0553060972717,25.0743589082228,
25.1622107786669,25.2499525693141,25.3376072318518,25.4280105142053,25.5155679067148,
25.6031126844816,25.6906654604034,25.7782468480054,25.865924475284,25.9536598314417,
26.0415187221286,26.0608334906796,26.148700249896,26.2364571125248,26.3241270104362,
26.4145246432738,26.502097579093,26.5896579870398,26.677226462896,26.7648236031118,
26.8525169822334,26.9402681076499,27.0281426752476,27.0473080731364,27.1351729963301,
27.2229280295589,27.3105961069842,27.4009944255604,27.4885655754207,27.5761242134951,
27.6636909376404,27.7512863463961,27.8389780328687,27.9267274864697,28.0146004251197,
28.0337826555933,28.1540582688503,28.2667246132152,28.2743338821073),
 .UNSPECIFIED.);
#1361=B_SPLINE_CURVE_WITH_KNOTS('',3,(#13034,#13035,#13036,#13037,#13038,
#13039,#13040,#13041,#13042,#13043,#13044,#13045,#13046,#13047,#13048,#13049,
#13050,#13051,#13052,#13053,#13054,#13055,#13056,#13057,#13058,#13059,#13060,
#13061,#13062,#13063,#13064,#13065,#13066,#13067,#13068,#13069,#13070,#13071,
#13072,#13073,#13074,#13075,#13076,#13077,#13078,#13079,#13080,#13081,#13082,
#13083,#13084,#13085,#13086,#13087,#13088,#13089,#13090,#13091,#13092,#13093,
#13094,#13095,#13096,#13097,#13098,#13099,#13100,#13101,#13102,#13103,#13104,
#13105,#13106,#13107,#13108,#13109,#13110,#13111,#13112,#13113,#13114,#13115,
#13116,#13117,#13118,#13119,#13120,#13121,#13122,#13123,#13124,#13125,#13126,
#13127,#13128,#13129,#13130),.UNSPECIFIED.,.F.,.F.,(4,3,3,3,3,3,3,3,3,3,
3,3,3,3,3,3,3,3,3,3,3,3,3,3,3,3,3,3,3,3,3,3,4),(0.,0.0371569355328809,0.0748591992606652,
0.112711498711869,0.148235810103463,0.156456024208327,0.161411147228472,
0.198370337527692,0.235138786797284,0.271056856315181,0.300871782327052,
0.307500754227861,0.312797824867268,0.348043230867719,0.383122091970086,
0.389313331030337,0.425334470814702,0.445315771807008,0.452555104475577,
0.457494349157134,0.49247276846388,0.52759487306579,0.562163035780557,0.595118177172423,
0.600660474525191,0.634670637653703,0.658985440093948,0.671142841314071,
0.679282696844516,0.683300242534193,0.715784112958499,0.74542767605421,
0.760759816994557),.UNSPECIFIED.);
#1362=B_SPLINE_CURVE_WITH_KNOTS('',3,(#13131,#13132,#13133,#13134,#13135,
#13136,#13137,#13138,#13139,#13140,#13141,#13142,#13143,#13144,#13145,#13146,
#13147,#13148,#13149,#13150,#13151,#13152,#13153,#13154,#13155,#13156,#13157,
#13158,#13159,#13160,#13161,#13162,#13163,#13164,#13165,#13166,#13167,#13168,
#13169,#13170,#13171,#13172,#13173,#13174,#13175,#13176,#13177,#13178,#13179,
#13180,#13181,#13182,#13183,#13184,#13185,#13186,#13187,#13188,#13189,#13190,
#13191,#13192,#13193,#13194,#13195,#13196,#13197,#13198,#13199,#13200,#13201,
#13202,#13203,#13204,#13205,#13206,#13207,#13208,#13209,#13210,#13211,#13212,
#13213,#13214,#13215,#13216,#13217,#13218,#13219,#13220,#13221),
 .UNSPECIFIED.,.F.,.F.,(4,3,3,3,3,3,3,3,3,3,3,3,3,3,3,3,3,3,3,3,3,3,3,3,
3,3,3,3,3,3,4),(-0.760759816994501,-0.728670005673473,-0.695695580357834,
-0.67904040478989,-0.673088551585097,-0.639573529909649,-0.605410590976213,
-0.599940992372035,-0.594530569322622,-0.55976930285687,-0.524694383676994,
-0.489867297069393,-0.455524569347743,-0.450701654934437,-0.41471168722101,
-0.406206270916632,-0.371647791277057,-0.336193695752684,-0.316381579222496,
-0.308862022274732,-0.30308148718843,-0.267013208605779,-0.230365762573195,
-0.19336779526563,-0.16051946557862,-0.152997977663309,-0.115126875727451,
-0.0772143395199071,-0.0399904833125805,-0.018319237973236,-7.36539879652355E-5),
 .UNSPECIFIED.);
#1363=B_SPLINE_CURVE_WITH_KNOTS('',3,(#13223,#13224,#13225,#13226,#13227,
#13228,#13229,#13230,#13231,#13232,#13233,#13234,#13235,#13236,#13237,#13238,
#13239,#13240,#13241,#13242,#13243,#13244,#13245,#13246,#13247,#13248,#13249,
#13250,#13251,#13252,#13253,#13254,#13255,#13256,#13257,#13258,#13259,#13260,
#13261,#13262,#13263,#13264,#13265,#13266,#13267,#13268,#13269,#13270,#13271,
#13272,#13273,#13274,#13275,#13276,#13277,#13278,#13279,#13280,#13281,#13282,
#13283,#13284,#13285,#13286,#13287,#13288,#13289,#13290,#13291,#13292,#13293,
#13294,#13295,#13296,#13297,#13298,#13299,#13300,#13301,#13302,#13303,#13304,
#13305,#13306,#13307,#13308,#13309,#13310,#13311,#13312,#13313),
 .UNSPECIFIED.,.F.,.F.,(4,3,3,3,3,3,3,3,3,3,3,3,3,3,3,3,3,3,3,3,3,3,3,3,
3,3,3,3,3,3,4),(-0.757763664684535,-0.720404510040711,-0.682461164219946,
-0.666249834426737,-0.657224676989519,-0.619850542291522,-0.582626533293054,
-0.567658451151491,-0.562369519249481,-0.525849388385921,-0.489664449823462,
-0.454476048800286,-0.419529152402925,-0.414641233789178,-0.379750615840662,
-0.370388554325077,-0.334979505679834,-0.299304808423338,-0.281536130666203,
-0.274019724168078,-0.268423813976394,-0.2336927258581,-0.198996831100818,
-0.165024314498677,-0.137477765641968,-0.130952085419143,-0.0975573927314685,
-0.0646607816327848,-0.0327251878282178,-0.0152860524042387,0.),
 .UNSPECIFIED.);
#1364=B_SPLINE_CURVE_WITH_KNOTS('',3,(#13538,#13539,#13540,#13541,#13542,
#13543,#13544,#13545,#13546,#13547,#13548,#13549,#13550,#13551,#13552,#13553,
#13554,#13555,#13556,#13557,#13558,#13559,#13560,#13561,#13562,#13563,#13564,
#13565,#13566,#13567,#13568,#13569,#13570,#13571,#13572,#13573,#13574,#13575,
#13576,#13577,#13578,#13579,#13580,#13581,#13582,#13583,#13584,#13585,#13586,
#13587,#13588,#13589,#13590,#13591,#13592,#13593,#13594,#13595,#13596,#13597,
#13598,#13599,#13600,#13601,#13602,#13603,#13604,#13605,#13606,#13607,#13608,
#13609,#13610,#13611,#13612,#13613,#13614,#13615,#13616,#13617,#13618,#13619,
#13620,#13621,#13622,#13623,#13624,#13625,#13626,#13627,#13628),
 .UNSPECIFIED.,.F.,.F.,(4,3,3,3,3,3,3,3,3,3,3,3,3,3,3,3,3,3,3,3,3,3,3,3,
3,3,3,3,3,3,4),(0.,0.0316034434157731,0.0643812777074898,0.0977466289617717,
0.11960441098055,0.130201724528789,0.138589441131514,0.172845323700023,
0.207497100291187,0.242107499729991,0.272608885111999,0.27741003130413,
0.313030306842683,0.348526801780242,0.353562303825158,0.388378619449034,
0.410240614928535,0.416663398207457,0.421583450321561,0.457807847609702,
0.49385749865802,0.530474689112555,0.566481039474124,0.571906953632555,
0.609227363829363,0.646598106922613,0.656083906904154,0.662136336864782,
0.700826509992472,0.739516683120162,0.757690266844663),.UNSPECIFIED.);
#1566=VERTEX_POINT('',#6410);
#1567=VERTEX_POINT('',#6411);
#1568=VERTEX_POINT('',#6413);
#1569=VERTEX_POINT('',#6418);
#1570=VERTEX_POINT('',#6476);
#1571=VERTEX_POINT('',#6477);
#1572=VERTEX_POINT('',#6479);
#1573=VERTEX_POINT('',#6681);
#1574=VERTEX_POINT('',#6910);
#1575=VERTEX_POINT('',#6911);
#1576=VERTEX_POINT('',#6913);
#1577=VERTEX_POINT('',#7144);
#1578=VERTEX_POINT('',#7379);
#1579=VERTEX_POINT('',#7380);
#1580=VERTEX_POINT('',#7382);
#1581=VERTEX_POINT('',#7613);
#1582=VERTEX_POINT('',#7845);
#1583=VERTEX_POINT('',#7846);
#1584=VERTEX_POINT('',#7848);
#1585=VERTEX_POINT('',#8082);
#1586=VERTEX_POINT('',#8317);
#1587=VERTEX_POINT('',#8318);
#1588=VERTEX_POINT('',#8320);
#1589=VERTEX_POINT('',#8548);
#1590=VERTEX_POINT('',#8780);
#1591=VERTEX_POINT('',#8781);
#1592=VERTEX_POINT('',#8783);
#1593=VERTEX_POINT('',#9017);
#1594=VERTEX_POINT('',#9246);
#1595=VERTEX_POINT('',#9247);
#1596=VERTEX_POINT('',#9249);
#1597=VERTEX_POINT('',#9284);
#1598=VERTEX_POINT('',#9292);
#1599=VERTEX_POINT('',#9294);
#1600=VERTEX_POINT('',#9487);
#1601=VERTEX_POINT('',#9488);
#1602=VERTEX_POINT('',#9490);
#1603=VERTEX_POINT('',#9495);
#1604=VERTEX_POINT('',#9647);
#1605=VERTEX_POINT('',#9649);
#1606=VERTEX_POINT('',#9863);
#1607=VERTEX_POINT('',#9864);
#1608=VERTEX_POINT('',#9866);
#1609=VERTEX_POINT('',#9881);
#1610=VERTEX_POINT('',#10098);
#1611=VERTEX_POINT('',#10099);
#1612=VERTEX_POINT('',#10101);
#1613=VERTEX_POINT('',#10317);
#1614=VERTEX_POINT('',#10534);
#1615=VERTEX_POINT('',#10535);
#1616=VERTEX_POINT('',#10709);
#1617=VERTEX_POINT('',#10926);
#1618=VERTEX_POINT('',#10927);
#1619=VERTEX_POINT('',#10929);
#1620=VERTEX_POINT('',#11106);
#1621=VERTEX_POINT('',#11323);
#1622=VERTEX_POINT('',#11324);
#1623=VERTEX_POINT('',#11486);
#1624=VERTEX_POINT('',#11703);
#1625=VERTEX_POINT('',#11704);
#1626=VERTEX_POINT('',#11706);
#1627=VERTEX_POINT('',#11877);
#1628=VERTEX_POINT('',#11893);
#1629=VERTEX_POINT('',#11895);
#1630=VERTEX_POINT('',#11897);
#1631=VERTEX_POINT('',#11899);
#1632=VERTEX_POINT('',#11942);
#1633=VERTEX_POINT('',#11944);
#1634=VERTEX_POINT('',#12131);
#1635=VERTEX_POINT('',#12345);
#1636=VERTEX_POINT('',#12576);
#1637=VERTEX_POINT('',#13630);
#1638=VERTEX_POINT('',#13632);
#1639=VERTEX_POINT('',#13636);
#1640=VERTEX_POINT('',#13639);
#2043=EDGE_CURVE('',#1566,#1567,#1021,.T.);
#2044=EDGE_CURVE('',#1567,#1568,#1296,.T.);
#2045=EDGE_CURVE('',#1569,#1568,#182,.T.);
#2046=EDGE_CURVE('',#1566,#1569,#1297,.T.);
#2047=EDGE_CURVE('',#1570,#1571,#1022,.T.);
#2048=EDGE_CURVE('',#1571,#1572,#1298,.T.);
#2049=EDGE_CURVE('',#1572,#1567,#1299,.T.);
#2050=EDGE_CURVE('',#1573,#1566,#1300,.T.);
#2051=EDGE_CURVE('',#1570,#1573,#1301,.T.);
#2052=EDGE_CURVE('',#1574,#1575,#1023,.T.);
#2053=EDGE_CURVE('',#1575,#1576,#1302,.T.);
#2054=EDGE_CURVE('',#1576,#1571,#1303,.T.);
#2055=EDGE_CURVE('',#1577,#1570,#1304,.T.);
#2056=EDGE_CURVE('',#1574,#1577,#1305,.T.);
#2057=EDGE_CURVE('',#1578,#1579,#1024,.T.);
#2058=EDGE_CURVE('',#1579,#1580,#1306,.T.);
#2059=EDGE_CURVE('',#1580,#1575,#1307,.T.);
#2060=EDGE_CURVE('',#1581,#1574,#1308,.T.);
#2061=EDGE_CURVE('',#1578,#1581,#1309,.T.);
#2062=EDGE_CURVE('',#1582,#1583,#1025,.T.);
#2063=EDGE_CURVE('',#1583,#1584,#1310,.T.);
#2064=EDGE_CURVE('',#1584,#1579,#1311,.T.);
#2065=EDGE_CURVE('',#1585,#1578,#1312,.T.);
#2066=EDGE_CURVE('',#1582,#1585,#1313,.T.);
#2067=EDGE_CURVE('',#1586,#1587,#1026,.T.);
#2068=EDGE_CURVE('',#1587,#1588,#1314,.T.);
#2069=EDGE_CURVE('',#1588,#1583,#1315,.T.);
#2070=EDGE_CURVE('',#1589,#1582,#1316,.T.);
#2071=EDGE_CURVE('',#1586,#1589,#1317,.T.);
#2072=EDGE_CURVE('',#1590,#1591,#1027,.T.);
#2073=EDGE_CURVE('',#1591,#1592,#1318,.T.);
#2074=EDGE_CURVE('',#1592,#1587,#1319,.T.);
#2075=EDGE_CURVE('',#1593,#1586,#1320,.T.);
#2076=EDGE_CURVE('',#1590,#1593,#1321,.T.);
#2077=EDGE_CURVE('',#1594,#1595,#1028,.T.);
#2078=EDGE_CURVE('',#1596,#1594,#1322,.T.);
#2079=EDGE_CURVE('',#1597,#1596,#1323,.T.);
#2080=EDGE_CURVE('',#1598,#1597,#183,.T.);
#2081=EDGE_CURVE('',#1598,#1599,#1324,.T.);
#2082=EDGE_CURVE('',#1599,#1595,#1325,.T.);
#2083=EDGE_CURVE('',#1600,#1601,#1029,.T.);
#2084=EDGE_CURVE('',#1601,#1602,#1326,.T.);
#2085=EDGE_CURVE('',#1602,#1603,#1327,.T.);
#2086=EDGE_CURVE('',#1604,#1603,#184,.F.);
#2087=EDGE_CURVE('',#1604,#1605,#1328,.T.);
#2088=EDGE_CURVE('',#1605,#1600,#1329,.T.);
#2089=EDGE_CURVE('',#1606,#1607,#1030,.T.);
#2090=EDGE_CURVE('',#1607,#1608,#1330,.T.);
#2091=EDGE_CURVE('',#1608,#1601,#1331,.T.);
#2092=EDGE_CURVE('',#1600,#1609,#1332,.T.);
#2093=EDGE_CURVE('',#1609,#1606,#1333,.T.);
#2094=EDGE_CURVE('',#1610,#1611,#1031,.T.);
#2095=EDGE_CURVE('',#1611,#1612,#1334,.T.);
#2096=EDGE_CURVE('',#1612,#1607,#1335,.T.);
#2097=EDGE_CURVE('',#1606,#1613,#1336,.T.);
#2098=EDGE_CURVE('',#1613,#1610,#1337,.T.);
#2099=EDGE_CURVE('',#1614,#1615,#1032,.T.);
#2100=EDGE_CURVE('',#1615,#1611,#1338,.T.);
#2101=EDGE_CURVE('',#1610,#1616,#1339,.T.);
#2102=EDGE_CURVE('',#1616,#1614,#1340,.T.);
#2103=EDGE_CURVE('',#1617,#1618,#1033,.T.);
#2104=EDGE_CURVE('',#1618,#1619,#1341,.T.);
#2105=EDGE_CURVE('',#1619,#1615,#1342,.T.);
#2106=EDGE_CURVE('',#1614,#1620,#1343,.T.);
#2107=EDGE_CURVE('',#1620,#1617,#1344,.T.);
#2108=EDGE_CURVE('',#1621,#1622,#1034,.T.);
#2109=EDGE_CURVE('',#1622,#1618,#1345,.T.);
#2110=EDGE_CURVE('',#1617,#1623,#1346,.T.);
#2111=EDGE_CURVE('',#1623,#1621,#1347,.T.);
#2112=EDGE_CURVE('',#1624,#1625,#1035,.T.);
#2113=EDGE_CURVE('',#1625,#1626,#1348,.T.);
#2114=EDGE_CURVE('',#1626,#1622,#1349,.T.);
#2115=EDGE_CURVE('',#1621,#1627,#1350,.T.);
#2116=EDGE_CURVE('',#1627,#1624,#1351,.T.);
#2117=EDGE_CURVE('',#1628,#1628,#185,.F.);
#2118=EDGE_CURVE('',#1628,#1629,#1036,.T.);
#2119=EDGE_CURVE('',#1629,#1630,#186,.T.);
#2120=EDGE_CURVE('',#1630,#1631,#1352,.T.);
#2121=EDGE_CURVE('',#1632,#1631,#1037,.T.);
#2122=EDGE_CURVE('',#1632,#1633,#1353,.T.);
#2123=EDGE_CURVE('',#1633,#1629,#187,.T.);
#2124=EDGE_CURVE('',#1631,#1625,#1354,.T.);
#2125=EDGE_CURVE('',#1624,#1634,#1355,.T.);
#2126=EDGE_CURVE('',#1634,#1632,#1356,.T.);
#2127=EDGE_CURVE('',#1595,#1635,#1357,.T.);
#2128=EDGE_CURVE('',#1635,#1591,#1358,.T.);
#2129=EDGE_CURVE('',#1636,#1590,#1359,.T.);
#2130=EDGE_CURVE('',#1594,#1636,#1360,.T.);
#2131=EDGE_CURVE('',#1568,#1604,#1361,.T.);
#2132=EDGE_CURVE('',#1633,#1598,#1362,.T.);
#2133=EDGE_CURVE('',#1597,#1630,#1363,.T.);
#2134=EDGE_CURVE('',#1603,#1569,#1364,.T.);
#2135=EDGE_CURVE('',#1637,#1637,#188,.T.);
#2136=EDGE_CURVE('',#1637,#1638,#1038,.T.);
#2137=EDGE_CURVE('',#1638,#1638,#189,.T.);
#2138=EDGE_CURVE('',#1639,#1639,#190,.T.);
#2139=EDGE_CURVE('',#1640,#1640,#191,.T.);
#2140=EDGE_CURVE('',#1639,#1640,#1039,.T.);
#2757=ORIENTED_EDGE('',*,*,#2043,.T.);
#2758=ORIENTED_EDGE('',*,*,#2044,.T.);
#2759=ORIENTED_EDGE('',*,*,#2045,.F.);
#2760=ORIENTED_EDGE('',*,*,#2046,.F.);
#2761=ORIENTED_EDGE('',*,*,#2047,.T.);
#2762=ORIENTED_EDGE('',*,*,#2048,.T.);
#2763=ORIENTED_EDGE('',*,*,#2049,.T.);
#2764=ORIENTED_EDGE('',*,*,#2043,.F.);
#2765=ORIENTED_EDGE('',*,*,#2050,.F.);
#2766=ORIENTED_EDGE('',*,*,#2051,.F.);
#2767=ORIENTED_EDGE('',*,*,#2052,.T.);
#2768=ORIENTED_EDGE('',*,*,#2053,.T.);
#2769=ORIENTED_EDGE('',*,*,#2054,.T.);
#2770=ORIENTED_EDGE('',*,*,#2047,.F.);
#2771=ORIENTED_EDGE('',*,*,#2055,.F.);
#2772=ORIENTED_EDGE('',*,*,#2056,.F.);
#2773=ORIENTED_EDGE('',*,*,#2057,.T.);
#2774=ORIENTED_EDGE('',*,*,#2058,.T.);
#2775=ORIENTED_EDGE('',*,*,#2059,.T.);
#2776=ORIENTED_EDGE('',*,*,#2052,.F.);
#2777=ORIENTED_EDGE('',*,*,#2060,.F.);
#2778=ORIENTED_EDGE('',*,*,#2061,.F.);
#2779=ORIENTED_EDGE('',*,*,#2062,.T.);
#2780=ORIENTED_EDGE('',*,*,#2063,.T.);
#2781=ORIENTED_EDGE('',*,*,#2064,.T.);
#2782=ORIENTED_EDGE('',*,*,#2057,.F.);
#2783=ORIENTED_EDGE('',*,*,#2065,.F.);
#2784=ORIENTED_EDGE('',*,*,#2066,.F.);
#2785=ORIENTED_EDGE('',*,*,#2067,.T.);
#2786=ORIENTED_EDGE('',*,*,#2068,.T.);
#2787=ORIENTED_EDGE('',*,*,#2069,.T.);
#2788=ORIENTED_EDGE('',*,*,#2062,.F.);
#2789=ORIENTED_EDGE('',*,*,#2070,.F.);
#2790=ORIENTED_EDGE('',*,*,#2071,.F.);
#2791=ORIENTED_EDGE('',*,*,#2072,.T.);
#2792=ORIENTED_EDGE('',*,*,#2073,.T.);
#2793=ORIENTED_EDGE('',*,*,#2074,.T.);
#2794=ORIENTED_EDGE('',*,*,#2067,.F.);
#2795=ORIENTED_EDGE('',*,*,#2075,.F.);
#2796=ORIENTED_EDGE('',*,*,#2076,.F.);
#2797=ORIENTED_EDGE('',*,*,#2077,.F.);
#2798=ORIENTED_EDGE('',*,*,#2078,.F.);
#2799=ORIENTED_EDGE('',*,*,#2079,.F.);
#2800=ORIENTED_EDGE('',*,*,#2080,.F.);
#2801=ORIENTED_EDGE('',*,*,#2081,.T.);
#2802=ORIENTED_EDGE('',*,*,#2082,.T.);
#2803=ORIENTED_EDGE('',*,*,#2083,.T.);
#2804=ORIENTED_EDGE('',*,*,#2084,.T.);
#2805=ORIENTED_EDGE('',*,*,#2085,.T.);
#2806=ORIENTED_EDGE('',*,*,#2086,.F.);
#2807=ORIENTED_EDGE('',*,*,#2087,.T.);
#2808=ORIENTED_EDGE('',*,*,#2088,.T.);
#2809=ORIENTED_EDGE('',*,*,#2089,.T.);
#2810=ORIENTED_EDGE('',*,*,#2090,.T.);
#2811=ORIENTED_EDGE('',*,*,#2091,.T.);
#2812=ORIENTED_EDGE('',*,*,#2083,.F.);
#2813=ORIENTED_EDGE('',*,*,#2092,.T.);
#2814=ORIENTED_EDGE('',*,*,#2093,.T.);
#2815=ORIENTED_EDGE('',*,*,#2094,.T.);
#2816=ORIENTED_EDGE('',*,*,#2095,.T.);
#2817=ORIENTED_EDGE('',*,*,#2096,.T.);
#2818=ORIENTED_EDGE('',*,*,#2089,.F.);
#2819=ORIENTED_EDGE('',*,*,#2097,.T.);
#2820=ORIENTED_EDGE('',*,*,#2098,.T.);
#2821=ORIENTED_EDGE('',*,*,#2099,.T.);
#2822=ORIENTED_EDGE('',*,*,#2100,.T.);
#2823=ORIENTED_EDGE('',*,*,#2094,.F.);
#2824=ORIENTED_EDGE('',*,*,#2101,.T.);
#2825=ORIENTED_EDGE('',*,*,#2102,.T.);
#2826=ORIENTED_EDGE('',*,*,#2103,.T.);
#2827=ORIENTED_EDGE('',*,*,#2104,.T.);
#2828=ORIENTED_EDGE('',*,*,#2105,.T.);
#2829=ORIENTED_EDGE('',*,*,#2099,.F.);
#2830=ORIENTED_EDGE('',*,*,#2106,.T.);
#2831=ORIENTED_EDGE('',*,*,#2107,.T.);
#2832=ORIENTED_EDGE('',*,*,#2108,.T.);
#2833=ORIENTED_EDGE('',*,*,#2109,.T.);
#2834=ORIENTED_EDGE('',*,*,#2103,.F.);
#2835=ORIENTED_EDGE('',*,*,#2110,.T.);
#2836=ORIENTED_EDGE('',*,*,#2111,.T.);
#2837=ORIENTED_EDGE('',*,*,#2112,.T.);
#2838=ORIENTED_EDGE('',*,*,#2113,.T.);
#2839=ORIENTED_EDGE('',*,*,#2114,.T.);
#2840=ORIENTED_EDGE('',*,*,#2108,.F.);
#2841=ORIENTED_EDGE('',*,*,#2115,.T.);
#2842=ORIENTED_EDGE('',*,*,#2116,.T.);
#2843=ORIENTED_EDGE('',*,*,#2117,.T.);
#2844=ORIENTED_EDGE('',*,*,#2118,.T.);
#2845=ORIENTED_EDGE('',*,*,#2119,.T.);
#2846=ORIENTED_EDGE('',*,*,#2120,.T.);
#2847=ORIENTED_EDGE('',*,*,#2121,.F.);
#2848=ORIENTED_EDGE('',*,*,#2122,.T.);
#2849=ORIENTED_EDGE('',*,*,#2123,.T.);
#2850=ORIENTED_EDGE('',*,*,#2118,.F.);
#2851=ORIENTED_EDGE('',*,*,#2121,.T.);
#2852=ORIENTED_EDGE('',*,*,#2124,.T.);
#2853=ORIENTED_EDGE('',*,*,#2112,.F.);
#2854=ORIENTED_EDGE('',*,*,#2125,.T.);
#2855=ORIENTED_EDGE('',*,*,#2126,.T.);
#2856=ORIENTED_EDGE('',*,*,#2077,.T.);
#2857=ORIENTED_EDGE('',*,*,#2127,.T.);
#2858=ORIENTED_EDGE('',*,*,#2128,.T.);
#2859=ORIENTED_EDGE('',*,*,#2072,.F.);
#2860=ORIENTED_EDGE('',*,*,#2129,.F.);
#2861=ORIENTED_EDGE('',*,*,#2130,.F.);
#2862=ORIENTED_EDGE('',*,*,#2131,.F.);
#2863=ORIENTED_EDGE('',*,*,#2044,.F.);
#2864=ORIENTED_EDGE('',*,*,#2049,.F.);
#2865=ORIENTED_EDGE('',*,*,#2048,.F.);
#2866=ORIENTED_EDGE('',*,*,#2054,.F.);
#2867=ORIENTED_EDGE('',*,*,#2053,.F.);
#2868=ORIENTED_EDGE('',*,*,#2059,.F.);
#2869=ORIENTED_EDGE('',*,*,#2058,.F.);
#2870=ORIENTED_EDGE('',*,*,#2064,.F.);
#2871=ORIENTED_EDGE('',*,*,#2063,.F.);
#2872=ORIENTED_EDGE('',*,*,#2069,.F.);
#2873=ORIENTED_EDGE('',*,*,#2068,.F.);
#2874=ORIENTED_EDGE('',*,*,#2074,.F.);
#2875=ORIENTED_EDGE('',*,*,#2073,.F.);
#2876=ORIENTED_EDGE('',*,*,#2128,.F.);
#2877=ORIENTED_EDGE('',*,*,#2127,.F.);
#2878=ORIENTED_EDGE('',*,*,#2082,.F.);
#2879=ORIENTED_EDGE('',*,*,#2081,.F.);
#2880=ORIENTED_EDGE('',*,*,#2132,.F.);
#2881=ORIENTED_EDGE('',*,*,#2122,.F.);
#2882=ORIENTED_EDGE('',*,*,#2126,.F.);
#2883=ORIENTED_EDGE('',*,*,#2125,.F.);
#2884=ORIENTED_EDGE('',*,*,#2116,.F.);
#2885=ORIENTED_EDGE('',*,*,#2115,.F.);
#2886=ORIENTED_EDGE('',*,*,#2111,.F.);
#2887=ORIENTED_EDGE('',*,*,#2110,.F.);
#2888=ORIENTED_EDGE('',*,*,#2107,.F.);
#2889=ORIENTED_EDGE('',*,*,#2106,.F.);
#2890=ORIENTED_EDGE('',*,*,#2102,.F.);
#2891=ORIENTED_EDGE('',*,*,#2101,.F.);
#2892=ORIENTED_EDGE('',*,*,#2098,.F.);
#2893=ORIENTED_EDGE('',*,*,#2097,.F.);
#2894=ORIENTED_EDGE('',*,*,#2093,.F.);
#2895=ORIENTED_EDGE('',*,*,#2092,.F.);
#2896=ORIENTED_EDGE('',*,*,#2088,.F.);
#2897=ORIENTED_EDGE('',*,*,#2087,.F.);
#2898=ORIENTED_EDGE('',*,*,#2080,.T.);
#2899=ORIENTED_EDGE('',*,*,#2133,.T.);
#2900=ORIENTED_EDGE('',*,*,#2119,.F.);
#2901=ORIENTED_EDGE('',*,*,#2123,.F.);
#2902=ORIENTED_EDGE('',*,*,#2132,.T.);
#2903=ORIENTED_EDGE('',*,*,#2134,.F.);
#2904=ORIENTED_EDGE('',*,*,#2085,.F.);
#2905=ORIENTED_EDGE('',*,*,#2084,.F.);
#2906=ORIENTED_EDGE('',*,*,#2091,.F.);
#2907=ORIENTED_EDGE('',*,*,#2090,.F.);
#2908=ORIENTED_EDGE('',*,*,#2096,.F.);
#2909=ORIENTED_EDGE('',*,*,#2095,.F.);
#2910=ORIENTED_EDGE('',*,*,#2100,.F.);
#2911=ORIENTED_EDGE('',*,*,#2105,.F.);
#2912=ORIENTED_EDGE('',*,*,#2104,.F.);
#2913=ORIENTED_EDGE('',*,*,#2109,.F.);
#2914=ORIENTED_EDGE('',*,*,#2114,.F.);
#2915=ORIENTED_EDGE('',*,*,#2113,.F.);
#2916=ORIENTED_EDGE('',*,*,#2124,.F.);
#2917=ORIENTED_EDGE('',*,*,#2120,.F.);
#2918=ORIENTED_EDGE('',*,*,#2133,.F.);
#2919=ORIENTED_EDGE('',*,*,#2079,.T.);
#2920=ORIENTED_EDGE('',*,*,#2078,.T.);
#2921=ORIENTED_EDGE('',*,*,#2130,.T.);
#2922=ORIENTED_EDGE('',*,*,#2129,.T.);
#2923=ORIENTED_EDGE('',*,*,#2076,.T.);
#2924=ORIENTED_EDGE('',*,*,#2075,.T.);
#2925=ORIENTED_EDGE('',*,*,#2071,.T.);
#2926=ORIENTED_EDGE('',*,*,#2070,.T.);
#2927=ORIENTED_EDGE('',*,*,#2066,.T.);
#2928=ORIENTED_EDGE('',*,*,#2065,.T.);
#2929=ORIENTED_EDGE('',*,*,#2061,.T.);
#2930=ORIENTED_EDGE('',*,*,#2060,.T.);
#2931=ORIENTED_EDGE('',*,*,#2056,.T.);
#2932=ORIENTED_EDGE('',*,*,#2055,.T.);
#2933=ORIENTED_EDGE('',*,*,#2051,.T.);
#2934=ORIENTED_EDGE('',*,*,#2050,.T.);
#2935=ORIENTED_EDGE('',*,*,#2046,.T.);
#2936=ORIENTED_EDGE('',*,*,#2135,.F.);
#2937=ORIENTED_EDGE('',*,*,#2136,.T.);
#2938=ORIENTED_EDGE('',*,*,#2137,.F.);
#2939=ORIENTED_EDGE('',*,*,#2136,.F.);
#2940=ORIENTED_EDGE('',*,*,#2135,.T.);
#2941=ORIENTED_EDGE('',*,*,#2138,.F.);
#2942=ORIENTED_EDGE('',*,*,#2139,.F.);
#2943=ORIENTED_EDGE('',*,*,#2117,.F.);
#2944=ORIENTED_EDGE('',*,*,#2138,.T.);
#2945=ORIENTED_EDGE('',*,*,#2140,.T.);
#2946=ORIENTED_EDGE('',*,*,#2139,.T.);
#2947=ORIENTED_EDGE('',*,*,#2140,.F.);
#2948=ORIENTED_EDGE('',*,*,#2137,.T.);
#2949=ORIENTED_EDGE('',*,*,#2131,.T.);
#2950=ORIENTED_EDGE('',*,*,#2086,.T.);
#2951=ORIENTED_EDGE('',*,*,#2134,.T.);
#2952=ORIENTED_EDGE('',*,*,#2045,.T.);
#4044=CYLINDRICAL_SURFACE('',#4523,4.085);
#4045=CYLINDRICAL_SURFACE('',#4525,4.085);
#4046=CYLINDRICAL_SURFACE('',#4526,4.085);
#4047=CYLINDRICAL_SURFACE('',#4527,4.085);
#4048=CYLINDRICAL_SURFACE('',#4528,4.085);
#4049=CYLINDRICAL_SURFACE('',#4529,4.085);
#4050=CYLINDRICAL_SURFACE('',#4530,4.085);
#4051=CYLINDRICAL_SURFACE('',#4531,4.085);
#4052=CYLINDRICAL_SURFACE('',#4533,3.38975);
#4053=CYLINDRICAL_SURFACE('',#4535,3.38975);
#4054=CYLINDRICAL_SURFACE('',#4536,3.38975);
#4055=CYLINDRICAL_SURFACE('',#4537,3.38975);
#4056=CYLINDRICAL_SURFACE('',#4538,3.38975);
#4057=CYLINDRICAL_SURFACE('',#4539,3.38975);
#4058=CYLINDRICAL_SURFACE('',#4540,3.38975);
#4059=CYLINDRICAL_SURFACE('',#4541,3.38975);
#4060=CYLINDRICAL_SURFACE('',#4545,3.38975);
#4061=CYLINDRICAL_SURFACE('',#4546,4.085);
#4062=CYLINDRICAL_SURFACE('',#4548,8.);
#4063=CYLINDRICAL_SURFACE('',#4555,5.);
#4168=ADVANCED_FACE('',(#533),#4044,.F.);
#4169=ADVANCED_FACE('',(#534),#4045,.F.);
#4170=ADVANCED_FACE('',(#535),#4046,.F.);
#4171=ADVANCED_FACE('',(#536),#4047,.F.);
#4172=ADVANCED_FACE('',(#537),#4048,.F.);
#4173=ADVANCED_FACE('',(#538),#4049,.F.);
#4174=ADVANCED_FACE('',(#539),#4050,.F.);
#4175=ADVANCED_FACE('',(#540),#4051,.F.);
#4176=ADVANCED_FACE('',(#541),#4052,.F.);
#4177=ADVANCED_FACE('',(#542),#4053,.F.);
#4178=ADVANCED_FACE('',(#543),#4054,.F.);
#4179=ADVANCED_FACE('',(#544),#4055,.F.);
#4180=ADVANCED_FACE('',(#545),#4056,.F.);
#4181=ADVANCED_FACE('',(#546),#4057,.F.);
#4182=ADVANCED_FACE('',(#547),#4058,.F.);
#4183=ADVANCED_FACE('',(#548),#4059,.F.);
#4184=ADVANCED_FACE('',(#549),#4060,.F.);
#4185=ADVANCED_FACE('',(#550),#4061,.F.);
#4186=ADVANCED_FACE('',(#551),#45,.F.);
#4187=ADVANCED_FACE('',(#552),#131,.T.);
#4188=ADVANCED_FACE('',(#553),#46,.F.);
#4189=ADVANCED_FACE('',(#554),#4062,.T.);
#4190=ADVANCED_FACE('',(#555,#97),#132,.F.);
#4191=ADVANCED_FACE('',(#556,#98),#133,.F.);
#4192=ADVANCED_FACE('',(#557),#4063,.T.);
#4193=ADVANCED_FACE('',(#558,#99),#134,.T.);
#4385=CLOSED_SHELL('',(#4168,#4169,#4170,#4171,#4172,#4173,#4174,#4175,
#4176,#4177,#4178,#4179,#4180,#4181,#4182,#4183,#4184,#4185,#4186,#4187,
#4188,#4189,#4190,#4191,#4192,#4193));
#4522=AXIS2_PLACEMENT_3D('',#6408,#5096,#5097);
#4523=AXIS2_PLACEMENT_3D('',#6409,#5098,#5099);
#4524=AXIS2_PLACEMENT_3D('',#6419,#5101,#5102);
#4525=AXIS2_PLACEMENT_3D('',#6475,#5103,#5104);
#4526=AXIS2_PLACEMENT_3D('',#6909,#5106,#5107);
#4527=AXIS2_PLACEMENT_3D('',#7378,#5109,#5110);
#4528=AXIS2_PLACEMENT_3D('',#7844,#5112,#5113);
#4529=AXIS2_PLACEMENT_3D('',#8316,#5115,#5116);
#4530=AXIS2_PLACEMENT_3D('',#8779,#5118,#5119);
#4531=AXIS2_PLACEMENT_3D('',#9245,#5121,#5122);
#4532=AXIS2_PLACEMENT_3D('',#9293,#5124,#5125);
#4533=AXIS2_PLACEMENT_3D('',#9486,#5126,#5127);
#4534=AXIS2_PLACEMENT_3D('',#9648,#5129,#5130);
#4535=AXIS2_PLACEMENT_3D('',#9862,#5131,#5132);
#4536=AXIS2_PLACEMENT_3D('',#10097,#5134,#5135);
#4537=AXIS2_PLACEMENT_3D('',#10533,#5137,#5138);
#4538=AXIS2_PLACEMENT_3D('',#10925,#5140,#5141);
#4539=AXIS2_PLACEMENT_3D('',#11322,#5143,#5144);
#4540=AXIS2_PLACEMENT_3D('',#11702,#5146,#5147);
#4541=AXIS2_PLACEMENT_3D('',#11892,#5149,#5150);
#4542=AXIS2_PLACEMENT_3D('',#11894,#5151,#5152);
#4543=AXIS2_PLACEMENT_3D('',#11898,#5154,#5155);
#4544=AXIS2_PLACEMENT_3D('',#11953,#5157,#5158);
#4545=AXIS2_PLACEMENT_3D('',#11954,#5159,#5160);
#4546=AXIS2_PLACEMENT_3D('',#12344,#5161,#5162);
#4547=AXIS2_PLACEMENT_3D('',#13222,#5163,#5164);
#4548=AXIS2_PLACEMENT_3D('',#13629,#5165,#5166);
#4549=AXIS2_PLACEMENT_3D('',#13631,#5167,#5168);
#4550=AXIS2_PLACEMENT_3D('',#13634,#5170,#5171);
#4551=AXIS2_PLACEMENT_3D('',#13635,#5172,#5173);
#4552=AXIS2_PLACEMENT_3D('',#13637,#5174,#5175);
#4553=AXIS2_PLACEMENT_3D('',#13638,#5176,#5177);
#4554=AXIS2_PLACEMENT_3D('',#13640,#5178,#5179);
#4555=AXIS2_PLACEMENT_3D('',#13641,#5180,#5181);
#4556=AXIS2_PLACEMENT_3D('',#13643,#5183,#5184);
#5096=DIRECTION('axis',(0.,0.,1.));
#5097=DIRECTION('refdir',(1.,0.,0.));
#5098=DIRECTION('center_axis',(0.,0.,1.));
#5099=DIRECTION('ref_axis',(0.566311127537338,0.824191547413215,0.));
#5100=DIRECTION('',(0.,0.,1.));
#5101=DIRECTION('center_axis',(0.,0.,-1.));
#5102=DIRECTION('ref_axis',(1.,3.22059269378563E-14,0.));
#5103=DIRECTION('center_axis',(0.,0.,1.));
#5104=DIRECTION('ref_axis',(0.566311127537338,0.824191547413215,0.));
#5105=DIRECTION('',(0.,0.,1.));
#5106=DIRECTION('center_axis',(0.,0.,1.));
#5107=DIRECTION('ref_axis',(0.566311127537338,0.824191547413215,0.));
#5108=DIRECTION('',(0.,0.,1.));
#5109=DIRECTION('center_axis',(0.,0.,1.));
#5110=DIRECTION('ref_axis',(0.566311127537338,0.824191547413215,0.));
#5111=DIRECTION('',(0.,0.,1.));
#5112=DIRECTION('center_axis',(0.,0.,1.));
#5113=DIRECTION('ref_axis',(0.566311127537338,0.824191547413215,0.));
#5114=DIRECTION('',(0.,0.,1.));
#5115=DIRECTION('center_axis',(0.,0.,1.));
#5116=DIRECTION('ref_axis',(0.566311127537338,0.824191547413215,0.));
#5117=DIRECTION('',(0.,0.,1.));
#5118=DIRECTION('center_axis',(0.,0.,1.));
#5119=DIRECTION('ref_axis',(0.566311127537338,0.824191547413215,0.));
#5120=DIRECTION('',(0.,0.,1.));
#5121=DIRECTION('center_axis',(0.,0.,1.));
#5122=DIRECTION('ref_axis',(0.566311127537338,0.824191547413215,0.));
#5123=DIRECTION('',(0.,0.,1.));
#5124=DIRECTION('center_axis',(0.,0.,1.));
#5125=DIRECTION('ref_axis',(1.,3.22059269378563E-14,0.));
#5126=DIRECTION('center_axis',(0.,0.,1.));
#5127=DIRECTION('ref_axis',(0.999190683258091,-0.0402241033489821,0.));
#5128=DIRECTION('',(0.,0.,1.));
#5129=DIRECTION('center_axis',(0.,0.,1.));
#5130=DIRECTION('ref_axis',(1.,0.,0.));
#5131=DIRECTION('center_axis',(0.,0.,1.));
#5132=DIRECTION('ref_axis',(0.999190683258091,-0.0402241033489821,0.));
#5133=DIRECTION('',(0.,0.,1.));
#5134=DIRECTION('center_axis',(0.,0.,1.));
#5135=DIRECTION('ref_axis',(0.999190683258091,-0.0402241033489821,0.));
#5136=DIRECTION('',(0.,0.,1.));
#5137=DIRECTION('center_axis',(0.,0.,1.));
#5138=DIRECTION('ref_axis',(0.999190683258091,-0.0402241033489821,0.));
#5139=DIRECTION('',(0.,0.,1.));
#5140=DIRECTION('center_axis',(0.,0.,1.));
#5141=DIRECTION('ref_axis',(0.999190683258091,-0.0402241033489821,0.));
#5142=DIRECTION('',(0.,0.,1.));
#5143=DIRECTION('center_axis',(0.,0.,1.));
#5144=DIRECTION('ref_axis',(0.999190683258091,-0.0402241033489821,0.));
#5145=DIRECTION('',(0.,0.,1.));
#5146=DIRECTION('center_axis',(0.,0.,1.));
#5147=DIRECTION('ref_axis',(0.999190683258091,-0.0402241033489821,0.));
#5148=DIRECTION('',(0.,0.,1.));
#5149=DIRECTION('center_axis',(0.,0.,1.));
#5150=DIRECTION('ref_axis',(0.999190683258091,-0.0402241033489821,0.));
#5151=DIRECTION('center_axis',(0.,0.,1.));
#5152=DIRECTION('ref_axis',(1.,0.,0.));
#5153=DIRECTION('',(0.,0.,1.));
#5154=DIRECTION('center_axis',(0.,0.,1.));
#5155=DIRECTION('ref_axis',(1.,0.,0.));
#5156=DIRECTION('',(0.,0.,1.));
#5157=DIRECTION('center_axis',(0.,0.,1.));
#5158=DIRECTION('ref_axis',(1.,0.,0.));
#5159=DIRECTION('center_axis',(0.,0.,1.));
#5160=DIRECTION('ref_axis',(0.999190683258091,-0.0402241033489821,0.));
#5161=DIRECTION('center_axis',(0.,0.,1.));
#5162=DIRECTION('ref_axis',(0.566311127537338,0.824191547413215,0.));
#5163=DIRECTION('center_axis',(0.,0.,1.));
#5164=DIRECTION('ref_axis',(1.,0.,0.));
#5165=DIRECTION('center_axis',(0.,0.,-1.));
#5166=DIRECTION('ref_axis',(-1.,0.,0.));
#5167=DIRECTION('center_axis',(0.,0.,-1.));
#5168=DIRECTION('ref_axis',(-1.,0.,0.));
#5169=DIRECTION('',(0.,0.,1.));
#5170=DIRECTION('center_axis',(0.,0.,1.));
#5171=DIRECTION('ref_axis',(-1.,0.,0.));
#5172=DIRECTION('center_axis',(0.,0.,1.));
#5173=DIRECTION('ref_axis',(-1.,0.,0.));
#5174=DIRECTION('center_axis',(0.,0.,-1.));
#5175=DIRECTION('ref_axis',(1.,0.,0.));
#5176=DIRECTION('center_axis',(0.,0.,1.));
#5177=DIRECTION('ref_axis',(1.,0.,0.));
#5178=DIRECTION('center_axis',(0.,0.,1.));
#5179=DIRECTION('ref_axis',(1.,0.,0.));
#5180=DIRECTION('center_axis',(0.,0.,1.));
#5181=DIRECTION('ref_axis',(1.,0.,0.));
#5182=DIRECTION('',(0.,0.,-1.));
#5183=DIRECTION('center_axis',(0.,0.,1.));
#5184=DIRECTION('ref_axis',(1.,0.,0.));
#6408=CARTESIAN_POINT('',(0.,0.,0.));
#6409=CARTESIAN_POINT('Origin',(0.,0.,46.4896150285955));
#6410=CARTESIAN_POINT('',(-2.31338095599003,-3.36682247118298,59.7031574977731));
#6411=CARTESIAN_POINT('',(-2.31666171942419,-3.37161025274083,59.8073433279728));
#6412=CARTESIAN_POINT('',(-2.31338095599002,-3.36682247118298,46.4896150285955));
#6413=CARTESIAN_POINT('',(1.46332546897508,-3.81390922438499,60.));
#6414=CARTESIAN_POINT('Ctrl Pts',(-2.31666171942481,-3.3716102527404,59.8073433279728));
#6415=CARTESIAN_POINT('Ctrl Pts',(-1.23546730076796,-4.11246432174188,59.8715622186486));
#6416=CARTESIAN_POINT('Ctrl Pts',(0.232198041727834,-4.28626973793002,59.9357811093243));
#6417=CARTESIAN_POINT('Ctrl Pts',(1.46332546897508,-3.81390922438499,60.));
#6418=CARTESIAN_POINT('',(3.17563310416156,-2.56954847935454,59.9999997913602));
#6419=CARTESIAN_POINT('Origin',(0.,0.,60.));
#6420=CARTESIAN_POINT('Ctrl Pts',(-2.31338095599003,-3.36682247118298,59.7031574977731));
#6421=CARTESIAN_POINT('Ctrl Pts',(-2.21469513777677,-3.43463058831267,59.7089734558387));
#6422=CARTESIAN_POINT('Ctrl Pts',(-2.11300662318653,-3.49810921792803,59.7147894139042));
#6423=CARTESIAN_POINT('Ctrl Pts',(-2.0087347754621,-3.5569944618806,59.7206053719698));
#6424=CARTESIAN_POINT('Ctrl Pts',(-1.90445636797313,-3.61588341031662,59.7264216959185));
#6425=CARTESIAN_POINT('Ctrl Pts',(-1.79759465807523,-3.67017819886025,59.7322380198673));
#6426=CARTESIAN_POINT('Ctrl Pts',(-1.68859434101989,-3.71966048873759,59.738054343816));
#6427=CARTESIAN_POINT('Ctrl Pts',(-1.57956176687172,-3.76915742219453,59.743872389023));
#6428=CARTESIAN_POINT('Ctrl Pts',(-1.46838969662447,-3.81383885657602,59.7496904342301));
#6429=CARTESIAN_POINT('Ctrl Pts',(-1.35554298540466,-3.85353450934596,59.7555084794371));
#6430=CARTESIAN_POINT('Ctrl Pts',(-1.24257680898892,-3.89327218592754,59.761332683919));
#6431=CARTESIAN_POINT('Ctrl Pts',(-1.1279328361525,-3.92801340962138,59.7671568884009));
#6432=CARTESIAN_POINT('Ctrl Pts',(-1.01209142685303,-3.95763767210827,59.7729810928828));
#6433=CARTESIAN_POINT('Ctrl Pts',(-0.896177332833092,-3.98728052234588,
59.7788089517633));
#6434=CARTESIAN_POINT('Ctrl Pts',(-0.779064702686944,-4.01179993297524,
59.7846368106437));
#6435=CARTESIAN_POINT('Ctrl Pts',(-0.66124285712451,-4.03112675115802,59.7904646695241));
#6436=CARTESIAN_POINT('Ctrl Pts',(-0.543257750327005,-4.05048034977521,
59.7963006038462));
#6437=CARTESIAN_POINT('Ctrl Pts',(-0.424561868666963,-4.06462694542446,
59.8021365381682));
#6438=CARTESIAN_POINT('Ctrl Pts',(-0.305648550467959,-4.0735493078637,59.8079724724903));
#6439=CARTESIAN_POINT('Ctrl Pts',(-0.27391858731232,-4.07593008602838,59.8095296906709));
#6440=CARTESIAN_POINT('Ctrl Pts',(-0.242173134744564,-4.07793918777959,
59.8110869088515));
#6441=CARTESIAN_POINT('Ctrl Pts',(-0.210421531939963,-4.07957691175152,
59.8126441270322));
#6442=CARTESIAN_POINT('Ctrl Pts',(-0.0923883607714591,-4.08566497461545,
59.8184329182687));
#6443=CARTESIAN_POINT('Ctrl Pts',(0.0261069165980141,-4.086636406536,59.8242217095052));
#6444=CARTESIAN_POINT('Ctrl Pts',(0.144580903785145,-4.08244061343955,59.8300105007417));
#6445=CARTESIAN_POINT('Ctrl Pts',(0.262908175693732,-4.07825001631031,59.8357921232812));
#6446=CARTESIAN_POINT('Ctrl Pts',(0.381213800033834,-4.06890493319291,59.8415737458207));
#6447=CARTESIAN_POINT('Ctrl Pts',(0.499010729166501,-4.05440665106212,59.8473553683602));
#6448=CARTESIAN_POINT('Ctrl Pts',(0.61669345438166,-4.03992242499058,59.8531313856267));
#6449=CARTESIAN_POINT('Ctrl Pts',(0.733868056967211,-4.02029498706776,59.8589074028932));
#6450=CARTESIAN_POINT('Ctrl Pts',(0.850049640732392,-3.9955776313683,59.8646834201597));
#6451=CARTESIAN_POINT('Ctrl Pts',(0.966153102927478,-3.97087689584714,59.8704555535788));
#6452=CARTESIAN_POINT('Ctrl Pts',(1.08126447101308,-3.94109313594346,59.876227686998));
#6453=CARTESIAN_POINT('Ctrl Pts',(1.19490673987542,-3.90633112818157,59.8819998204171));
#6454=CARTESIAN_POINT('Ctrl Pts',(1.30850926666104,-3.87158127711449,59.8877699352514));
#6455=CARTESIAN_POINT('Ctrl Pts',(1.42064332039576,-3.83185675992719,59.8935400500856));
#6456=CARTESIAN_POINT('Ctrl Pts',(1.53084539717501,-3.7873126844701,59.8993101649198));
#6457=CARTESIAN_POINT('Ctrl Pts',(1.64103575391707,-3.74277334629415,59.9050796660999));
#6458=CARTESIAN_POINT('Ctrl Pts',(1.74929415882466,-3.69341562428457,59.91084916728));
#6459=CARTESIAN_POINT('Ctrl Pts',(1.8551761647154,-3.63944314392626,59.9166186684601));
#6460=CARTESIAN_POINT('Ctrl Pts',(1.96107267801672,-3.5854632685349,59.9223889601478));
#6461=CARTESIAN_POINT('Ctrl Pts',(2.06459177664333,-3.52686756612609,59.9281592518354));
#6462=CARTESIAN_POINT('Ctrl Pts',(2.16531338027168,-3.46390573850046,59.933929543523));
#6463=CARTESIAN_POINT('Ctrl Pts',(2.2661332664976,-3.40088247368814,59.9397054657729));
#6464=CARTESIAN_POINT('Ctrl Pts',(2.36414985453216,-3.33348479456704,59.9454813880227));
#6465=CARTESIAN_POINT('Ctrl Pts',(2.45897173564387,-3.2620059784287,59.9512573102726));
#6466=CARTESIAN_POINT('Ctrl Pts',(2.55384135103432,-3.19049117914286,59.9570361401791));
#6467=CARTESIAN_POINT('Ctrl Pts',(2.64551273705809,-3.11489141383132,59.9628149700857));
#6468=CARTESIAN_POINT('Ctrl Pts',(2.73362866411939,-3.03553937986395,59.9685937999923));
#6469=CARTESIAN_POINT('Ctrl Pts',(2.82188055805937,-2.95606490210311,59.974381546896));
#6470=CARTESIAN_POINT('Ctrl Pts',(2.90656573841288,-2.87282687955783,59.9801692937997));
#6471=CARTESIAN_POINT('Ctrl Pts',(2.987364550522,-2.78619418603307,59.9859570407034));
#6472=CARTESIAN_POINT('Ctrl Pts',(3.05271165885833,-2.71612884891419,59.990637957589));
#6473=CARTESIAN_POINT('Ctrl Pts',(3.11551739932373,-2.64384379773319,59.9953188744746));
#6474=CARTESIAN_POINT('Ctrl Pts',(3.17563310416156,-2.56954847935454,59.9999997913602));
#6475=CARTESIAN_POINT('Origin',(0.,0.,46.4896150285955));
#6476=CARTESIAN_POINT('',(-2.31338095599002,-3.36682247118298,58.4531830718678));
#6477=CARTESIAN_POINT('',(-2.31338095599002,-3.36682247118299,58.5572666440642));
#6478=CARTESIAN_POINT('',(-2.31338095599002,-3.36682247118298,46.4896150285955));
#6479=CARTESIAN_POINT('',(-4.08799668051687,0.000978769805548399,59.6146155644207));
#6480=CARTESIAN_POINT('Ctrl Pts',(-2.31338095599002,-3.36682247118299,58.5572666440642));
#6481=CARTESIAN_POINT('Ctrl Pts',(-2.21480203430358,-3.43455713852685,58.5630789515449));
#6482=CARTESIAN_POINT('Ctrl Pts',(-2.11329234559576,-3.49792673610757,58.5688912590256));
#6483=CARTESIAN_POINT('Ctrl Pts',(-2.00928105362083,-3.55668590791489,58.5747035665063));
#6484=CARTESIAN_POINT('Ctrl Pts',(-1.90521720845016,-3.61547476863578,58.5805188107387));
#6485=CARTESIAN_POINT('Ctrl Pts',(-1.79864960515187,-3.66964837696318,58.586334054971));
#6486=CARTESIAN_POINT('Ctrl Pts',(-1.69003007411857,-3.71900838242868,58.5921492992033));
#6487=CARTESIAN_POINT('Ctrl Pts',(-1.58123532526954,-3.76844801217777,58.5979739242016));
#6488=CARTESIAN_POINT('Ctrl Pts',(-1.4703824130478,-3.81305836949707,58.6037985491998));
#6489=CARTESIAN_POINT('Ctrl Pts',(-1.35794170423633,-3.85268988213375,58.6096231741981));
#6490=CARTESIAN_POINT('Ctrl Pts',(-1.25108141854553,-3.89035448606127,58.6151587235372));
#6491=CARTESIAN_POINT('Ctrl Pts',(-1.14278744447073,-3.92352250021008,58.6206942728764));
#6492=CARTESIAN_POINT('Ctrl Pts',(-1.03347228199655,-3.95210830346852,58.6262298222155));
#6493=CARTESIAN_POINT('Ctrl Pts',(-0.918388533385041,-3.98220258610594,
58.6320574837599));
#6494=CARTESIAN_POINT('Ctrl Pts',(-0.80180629177334,-4.00731374478515,58.6378851453043));
#6495=CARTESIAN_POINT('Ctrl Pts',(-0.684194478847014,-4.02729473904199,
58.6437128068487));
#6496=CARTESIAN_POINT('Ctrl Pts',(-0.566729849994398,-4.04725072829245,
58.649533175427));
#6497=CARTESIAN_POINT('Ctrl Pts',(-0.448238611066349,-4.06208925536335,
58.6553535440054));
#6498=CARTESIAN_POINT('Ctrl Pts',(-0.329203545658992,-4.0717134016929,58.6611739125836));
#6499=CARTESIAN_POINT('Ctrl Pts',(-0.210286549509897,-4.08132800196293,
58.6669885080177));
#6500=CARTESIAN_POINT('Ctrl Pts',(-0.0908272040805449,-4.08573847844648,
58.6728031034518));
#6501=CARTESIAN_POINT('Ctrl Pts',(0.028683427381987,-4.08489929630996,58.6786176988859));
#6502=CARTESIAN_POINT('Ctrl Pts',(0.15188917382253,-4.08403416774137,58.6846120741305));
#6503=CARTESIAN_POINT('Ctrl Pts',(0.275148994387207,-4.07758940390421,58.6906064493751));
#6504=CARTESIAN_POINT('Ctrl Pts',(0.39792082571284,-4.06557302436742,58.6966008246197));
#6505=CARTESIAN_POINT('Ctrl Pts',(0.516878449304106,-4.05392996310137,58.7024089699109));
#6506=CARTESIAN_POINT('Ctrl Pts',(0.635377520845544,-4.03705639683912,58.7082171152021));
#6507=CARTESIAN_POINT('Ctrl Pts',(0.752927554220468,-4.01501246549691,58.7140252604934));
#6508=CARTESIAN_POINT('Ctrl Pts',(0.870460595530278,-3.99297172064395,58.7198325662069));
#6509=CARTESIAN_POINT('Ctrl Pts',(0.987044470944633,-3.96576217225358,58.7256398719205));
#6510=CARTESIAN_POINT('Ctrl Pts',(1.10219760709635,-3.93349532031132,58.7314471776341));
#6511=CARTESIAN_POINT('Ctrl Pts',(1.21736116147698,-3.90122554909599,58.737255008751));
#6512=CARTESIAN_POINT('Ctrl Pts',(1.33109332668071,-3.86389767461634,58.7430628398679));
#6513=CARTESIAN_POINT('Ctrl Pts',(1.44292705635254,-3.82167326050328,58.7488706709848));
#6514=CARTESIAN_POINT('Ctrl Pts',(1.55479718736688,-3.77943510254599,58.7546803925229));
#6515=CARTESIAN_POINT('Ctrl Pts',(1.66476727271772,-3.73229737908953,58.7604901140609));
#6516=CARTESIAN_POINT('Ctrl Pts',(1.77239022362783,-3.68046979272871,58.766299835599));
#6517=CARTESIAN_POINT('Ctrl Pts',(1.88013104605108,-3.62858544341932,58.7721159200983));
#6518=CARTESIAN_POINT('Ctrl Pts',(1.98551923548309,-3.57200115566269,58.7779320045977));
#6519=CARTESIAN_POINT('Ctrl Pts',(2.08813216743317,-3.51097266456617,58.783748089097));
#6520=CARTESIAN_POINT('Ctrl Pts',(2.19081247945898,-3.44990409953088,58.7895679926882));
#6521=CARTESIAN_POINT('Ctrl Pts',(2.29071356451001,-3.38438574219185,58.7953878962794));
#6522=CARTESIAN_POINT('Ctrl Pts',(2.3874430131871,-3.3147158036224,58.8012077998706));
#6523=CARTESIAN_POINT('Ctrl Pts',(2.48430817974334,-3.24494811347438,58.8070358691754));
#6524=CARTESIAN_POINT('Ctrl Pts',(2.57799250963747,-3.1710174681164,58.8128639384801));
#6525=CARTESIAN_POINT('Ctrl Pts',(2.66813771436471,-3.0932614078323,58.8186920077849));
#6526=CARTESIAN_POINT('Ctrl Pts',(2.68768181703163,-3.07640335720425,58.819955573442));
#6527=CARTESIAN_POINT('Ctrl Pts',(2.70705970490966,-3.0593656245969,58.8212191390991));
#6528=CARTESIAN_POINT('Ctrl Pts',(2.7262679680436,-3.04215186445703,58.8224827047561));
#6529=CARTESIAN_POINT('Ctrl Pts',(2.81485875306806,-2.9627599635142,58.8283104192511));
#6530=CARTESIAN_POINT('Ctrl Pts',(2.90011916689984,-2.87936917863925,58.8341381337461));
#6531=CARTESIAN_POINT('Ctrl Pts',(2.9816679295944,-2.79228962638697,58.8399658482411));
#6532=CARTESIAN_POINT('Ctrl Pts',(3.06311488129128,-2.70531879014458,58.8457862870227));
#6533=CARTESIAN_POINT('Ctrl Pts',(3.14085912268164,-2.61466864175858,58.8516067258043));
#6534=CARTESIAN_POINT('Ctrl Pts',(3.21455354374732,-2.52068850006928,58.8574271645859));
#6535=CARTESIAN_POINT('Ctrl Pts',(3.288175083505,-2.42680130158455,58.863241847149));
#6536=CARTESIAN_POINT('Ctrl Pts',(3.35775452088454,-2.32959098058406,58.869056529712));
#6537=CARTESIAN_POINT('Ctrl Pts',(3.42298304622498,-2.22944209730963,58.8748712122751));
#6538=CARTESIAN_POINT('Ctrl Pts',(3.49022705116358,-2.1261987391875,58.8808655612344));
#6539=CARTESIAN_POINT('Ctrl Pts',(3.55284659891326,-2.01983259477798,58.8868599101936));
#6540=CARTESIAN_POINT('Ctrl Pts',(3.61054944869451,-1.91080027175312,58.8928542591528));
#6541=CARTESIAN_POINT('Ctrl Pts',(3.66646109651549,-1.80515251138807,58.8986625325604));
#6542=CARTESIAN_POINT('Ctrl Pts',(3.71775657481677,-1.69700203731464,58.904470805968));
#6543=CARTESIAN_POINT('Ctrl Pts',(3.76421554653954,-1.58679120214037,58.9102790793755));
#6544=CARTESIAN_POINT('Ctrl Pts',(3.81066792155213,-1.47659601580442,58.9160865280663));
#6545=CARTESIAN_POINT('Ctrl Pts',(3.85228499748508,-1.36434142572157,58.921893976757));
#6546=CARTESIAN_POINT('Ctrl Pts',(3.88889419766639,-1.25049067143929,58.9277014254477));
#6547=CARTESIAN_POINT('Ctrl Pts',(3.9255068021072,-1.13662933026876,58.9335094141683));
#6548=CARTESIAN_POINT('Ctrl Pts',(3.95711048011525,-1.02117191786059,58.9393174028889));
#6549=CARTESIAN_POINT('Ctrl Pts',(3.98358242959187,-0.904597162634811,58.9451253916095));
#6550=CARTESIAN_POINT('Ctrl Pts',(4.01006306097334,-0.787984174828753,58.9509352851542));
#6551=CARTESIAN_POINT('Ctrl Pts',(4.03140852632769,-0.670253512687353,58.9567451786988));
#6552=CARTESIAN_POINT('Ctrl Pts',(4.04754718700238,-0.55189380227464,58.9625550722435));
#6553=CARTESIAN_POINT('Ctrl Pts',(4.06370357871512,-0.433404053776822,58.9683713489351));
#6554=CARTESIAN_POINT('Ctrl Pts',(4.07464169228339,-0.314284281622832,58.9741876256268));
#6555=CARTESIAN_POINT('Ctrl Pts',(4.08034178029111,-0.195028090312132,58.9800039023184));
#6556=CARTESIAN_POINT('Ctrl Pts',(4.08604562287243,-0.0756933465039628,
58.9858240101157));
#6557=CARTESIAN_POINT('Ctrl Pts',(4.08650456688263,0.0437775887584125,58.9916441179129));
#6558=CARTESIAN_POINT('Ctrl Pts',(4.08175096073643,0.162892892807668,58.9974642257101));
#6559=CARTESIAN_POINT('Ctrl Pts',(4.07699067235224,0.282175639590705,59.0032925149478));
#6560=CARTESIAN_POINT('Ctrl Pts',(4.06700324362255,0.401101352731584,59.0091208041854));
#6561=CARTESIAN_POINT('Ctrl Pts',(4.05187264766116,0.519184983541846,59.014949093423));
#6562=CARTESIAN_POINT('Ctrl Pts',(4.04859599096257,0.544756978252116,59.0162112580476));
#6563=CARTESIAN_POINT('Ctrl Pts',(4.04507832130802,0.570289527183952,59.0174734226722));
#6564=CARTESIAN_POINT('Ctrl Pts',(4.04132080248762,0.595777786914541,59.0187355872969));
#6565=CARTESIAN_POINT('Ctrl Pts',(4.02399372819974,0.713311987255443,59.0245558163521));
#6566=CARTESIAN_POINT('Ctrl Pts',(4.00150705452874,0.830279252287219,59.0303760454074));
#6567=CARTESIAN_POINT('Ctrl Pts',(3.9739082330223,0.946191500446708,59.0361962744627));
#6568=CARTESIAN_POINT('Ctrl Pts',(3.94634404342939,1.0619582980856,59.0420092001022));
#6569=CARTESIAN_POINT('Ctrl Pts',(3.91368055870973,1.17667231773673,59.0478221257416));
#6570=CARTESIAN_POINT('Ctrl Pts',(3.87601678876237,1.28985226023457,59.0536350513811));
#6571=CARTESIAN_POINT('Ctrl Pts',(3.8383904348959,1.4029197670976,59.0594422023226));
#6572=CARTESIAN_POINT('Ctrl Pts',(3.79577380602717,1.51445584284936,59.0652493532641));
#6573=CARTESIAN_POINT('Ctrl Pts',(3.74831645208154,1.62399161791399,59.0710565042056));
#6574=CARTESIAN_POINT('Ctrl Pts',(3.69930625825683,1.73711148491725,59.0770536694402));
#6575=CARTESIAN_POINT('Ctrl Pts',(3.64513321897757,1.84809746915126,59.0830508346749));
#6576=CARTESIAN_POINT('Ctrl Pts',(3.58601726917939,1.95645218319979,59.0890479999095));
#6577=CARTESIAN_POINT('Ctrl Pts',(3.52883750725453,2.06125802280622,59.0948487437276));
#6578=CARTESIAN_POINT('Ctrl Pts',(3.46703376658915,2.1636018711068,59.1006494875457));
#6579=CARTESIAN_POINT('Ctrl Pts',(3.40085273196375,2.26305671504157,59.1064502313638));
#6580=CARTESIAN_POINT('Ctrl Pts',(3.33468094939703,2.36249765526422,59.1122501642423));
#6581=CARTESIAN_POINT('Ctrl Pts',(3.26413331623943,2.45905005402977,59.1180500971208));
#6582=CARTESIAN_POINT('Ctrl Pts',(3.18950029622193,2.5523151961308,59.1238500299992));
#6583=CARTESIAN_POINT('Ctrl Pts',(3.11486004490109,2.64558937482895,59.1296505248418));
#6584=CARTESIAN_POINT('Ctrl Pts',(3.03613387514371,2.73557534438076,59.1354510196843));
#6585=CARTESIAN_POINT('Ctrl Pts',(2.95365262978066,2.82190735896659,59.1412515145268));
#6586=CARTESIAN_POINT('Ctrl Pts',(2.8711438702172,2.9082681722974,59.1470539443059));
#6587=CARTESIAN_POINT('Ctrl Pts',(2.78487782617163,2.99097231118155,59.152856374085));
#6588=CARTESIAN_POINT('Ctrl Pts',(2.69522181074791,3.06969125334597,59.1586588038641));
#6589=CARTESIAN_POINT('Ctrl Pts',(2.60546590609003,3.14849789932825,59.1644676983546));
#6590=CARTESIAN_POINT('Ctrl Pts',(2.51231279877493,3.22331021641309,59.1702765928451));
#6591=CARTESIAN_POINT('Ctrl Pts',(2.41616256541551,3.29384022950184,59.1760854873356));
#6592=CARTESIAN_POINT('Ctrl Pts',(2.31994826942968,3.36441723507018,59.1818982521551));
#6593=CARTESIAN_POINT('Ctrl Pts',(2.22073320978952,3.43070602817889,59.1877110169746));
#6594=CARTESIAN_POINT('Ctrl Pts',(2.11894467561774,3.49246309381663,59.1935237817942));
#6595=CARTESIAN_POINT('Ctrl Pts',(2.01701091720085,3.55430826980305,59.1993448398305));
#6596=CARTESIAN_POINT('Ctrl Pts',(1.91249671358373,3.61160861883483,59.2051658978668));
#6597=CARTESIAN_POINT('Ctrl Pts',(1.80585213975437,3.66416744286401,59.2109869559032));
#6598=CARTESIAN_POINT('Ctrl Pts',(1.7814155885564,3.6762107784804,59.2123207938813));
#6599=CARTESIAN_POINT('Ctrl Pts',(1.75686725501579,3.6880053628731,59.2136546318593));
#6600=CARTESIAN_POINT('Ctrl Pts',(1.7322126759275,3.69954919488254,59.2149884698374));
#6601=CARTESIAN_POINT('Ctrl Pts',(1.6243304851827,3.75006207860726,59.2208250068418));
#6602=CARTESIAN_POINT('Ctrl Pts',(1.51406786472336,3.79593132511904,59.2266615438461));
#6603=CARTESIAN_POINT('Ctrl Pts',(1.4018606953227,3.83692736325688,59.2324980808505));
#6604=CARTESIAN_POINT('Ctrl Pts',(1.28979407647794,3.87787204981014,59.2383273070161));
#6605=CARTESIAN_POINT('Ctrl Pts',(1.17578813223202,3.9139555320868,59.2441565331817));
#6606=CARTESIAN_POINT('Ctrl Pts',(1.0603013915889,3.94499505183399,59.2499857593473));
#6607=CARTESIAN_POINT('Ctrl Pts',(0.944929590676493,3.97600367908199,59.2558091838973));
#6608=CARTESIAN_POINT('Ctrl Pts',(0.828080315782685,4.0019782267766,59.2616326084472));
#6609=CARTESIAN_POINT('Ctrl Pts',(0.710229496298609,4.0227849883616,59.2674560329971));
#6610=CARTESIAN_POINT('Ctrl Pts',(0.588986277256128,4.04419068382862,59.2734470879713));
#6611=CARTESIAN_POINT('Ctrl Pts',(0.466683389476337,4.06012641257512,59.2794381429455));
#6612=CARTESIAN_POINT('Ctrl Pts',(0.343853381635293,4.07050240780398,59.2854291979197));
#6613=CARTESIAN_POINT('Ctrl Pts',(0.224595022545729,4.08057669003081,59.2912460451055));
#6614=CARTESIAN_POINT('Ctrl Pts',(0.104840207494035,4.08541006779284,59.2970628922913));
#6615=CARTESIAN_POINT('Ctrl Pts',(-0.0149166290420977,4.08497276541448,
59.3028797394771));
#6616=CARTESIAN_POINT('Ctrl Pts',(-0.134654890628517,4.08453553086414,59.3086956844376));
#6617=CARTESIAN_POINT('Ctrl Pts',(-0.254394766907548,4.07882924373015,59.3145116293981));
#6618=CARTESIAN_POINT('Ctrl Pts',(-0.373641271704787,4.0678762518148,59.3203275743586));
#6619=CARTESIAN_POINT('Ctrl Pts',(-0.492897068477597,4.05692240641587,59.3261439725116));
#6620=CARTESIAN_POINT('Ctrl Pts',(-0.611659012737289,4.04072108060403,59.3319603706646));
#6621=CARTESIAN_POINT('Ctrl Pts',(-0.729437304627361,4.01934649148565,59.3377767688175));
#6622=CARTESIAN_POINT('Ctrl Pts',(-0.853404820528018,3.99684867228755,59.3438988174476));
#6623=CARTESIAN_POINT('Ctrl Pts',(-0.976282000004267,3.96861920300436,59.3500208660776));
#6624=CARTESIAN_POINT('Ctrl Pts',(-1.09751133468474,3.93480544248868,59.3561429147077));
#6625=CARTESIAN_POINT('Ctrl Pts',(-1.21285000561375,3.90263472896237,59.3619674864107));
#6626=CARTESIAN_POINT('Ctrl Pts',(-1.32669682307987,3.86540981904723,59.3677920581137));
#6627=CARTESIAN_POINT('Ctrl Pts',(-1.43858953256563,3.82330814306048,59.3736166298167));
#6628=CARTESIAN_POINT('Ctrl Pts',(-1.55055517746741,3.78117902379108,59.3794449981706));
#6629=CARTESIAN_POINT('Ctrl Pts',(-1.66056380461322,3.73416696619259,59.3852733665245));
#6630=CARTESIAN_POINT('Ctrl Pts',(-1.76817536986392,3.68249655280308,59.3911017348784));
#6631=CARTESIAN_POINT('Ctrl Pts',(-1.87593288195363,3.63075606206188,59.396938007884));
#6632=CARTESIAN_POINT('Ctrl Pts',(-1.98128648734886,3.57434479807323,59.4027742808896));
#6633=CARTESIAN_POINT('Ctrl Pts',(-2.08382278545184,3.5135320688492,59.4086105538952));
#6634=CARTESIAN_POINT('Ctrl Pts',(-2.09922944064847,3.50439461442521,59.4094874867228));
#6635=CARTESIAN_POINT('Ctrl Pts',(-2.11457254781778,3.49515786583985,59.4103644195504));
#6636=CARTESIAN_POINT('Ctrl Pts',(-2.12985076712583,3.4858228167498,59.4112413523781));
#6637=CARTESIAN_POINT('Ctrl Pts',(-2.23144216804306,3.42375009115478,59.4170724530236));
#6638=CARTESIAN_POINT('Ctrl Pts',(-2.33047596081803,3.35713581779339,59.4229035536691));
#6639=CARTESIAN_POINT('Ctrl Pts',(-2.42652081805006,3.28621693130105,59.4287346543146));
#6640=CARTESIAN_POINT('Ctrl Pts',(-2.5224473135942,3.21538544229515,59.4345585689542));
#6641=CARTESIAN_POINT('Ctrl Pts',(-2.61539187581421,3.14026013195042,59.4403824835938));
#6642=CARTESIAN_POINT('Ctrl Pts',(-2.70494976812292,3.06112262935214,59.4462063982334));
#6643=CARTESIAN_POINT('Ctrl Pts',(-2.79442043709696,2.98206220133317,59.4520246407737));
#6644=CARTESIAN_POINT('Ctrl Pts',(-2.88051069512174,2.89899762343173,59.457842883314));
#6645=CARTESIAN_POINT('Ctrl Pts',(-2.96284716265808,2.81225206742372,59.4636611258543));
#6646=CARTESIAN_POINT('Ctrl Pts',(-3.04765735257003,2.72290032208913,59.4696541720653));
#6647=CARTESIAN_POINT('Ctrl Pts',(-3.12848427370886,2.62964318008027,59.4756472182763));
#6648=CARTESIAN_POINT('Ctrl Pts',(-3.20495877380643,2.53287667646911,59.4816402644873));
#6649=CARTESIAN_POINT('Ctrl Pts',(-3.27912323320859,2.43903316759487,59.4874522806737));
#6650=CARTESIAN_POINT('Ctrl Pts',(-3.34919416765684,2.34188960451496,59.4932642968601));
#6651=CARTESIAN_POINT('Ctrl Pts',(-3.41487480817952,2.24184188658809,59.4990763130465));
#6652=CARTESIAN_POINT('Ctrl Pts',(-3.48054681238641,2.14180732388749,59.5048875650136));
#6653=CARTESIAN_POINT('Ctrl Pts',(-3.54182944750191,2.0388697059567,59.5106988169808));
#6654=CARTESIAN_POINT('Ctrl Pts',(-3.59846916632478,1.93345407470927,59.516510068948));
#6655=CARTESIAN_POINT('Ctrl Pts',(-3.65511469235969,1.82802763530572,59.5223219167368));
#6656=CARTESIAN_POINT('Ctrl Pts',(-3.70711616289021,1.72012303589154,59.5281337645257));
#6657=CARTESIAN_POINT('Ctrl Pts',(-3.75426620079138,1.61018952101777,59.5339456123145));
#6658=CARTESIAN_POINT('Ctrl Pts',(-3.80143210680293,1.50021900856721,59.5397594160518));
#6659=CARTESIAN_POINT('Ctrl Pts',(-3.84374317245761,1.38821859637699,59.545573219789));
#6660=CARTESIAN_POINT('Ctrl Pts',(-3.8810405605059,1.27465649008196,59.5513870235263));
#6661=CARTESIAN_POINT('Ctrl Pts',(-3.91837924876688,1.16096863398541,59.5572072650155));
#6662=CARTESIAN_POINT('Ctrl Pts',(-3.9506930508458,1.04571601888337,59.5630275065047));
#6663=CARTESIAN_POINT('Ctrl Pts',(-3.9778732688924,0.929381114845428,59.5688477479938));
#6664=CARTESIAN_POINT('Ctrl Pts',(-4.00507154745216,0.812968909438439,59.5746718568746));
#6665=CARTESIAN_POINT('Ctrl Pts',(-4.02712937328489,0.695473381826771,59.5804959657555));
#6666=CARTESIAN_POINT('Ctrl Pts',(-4.04398960873745,0.577384658978328,59.5863200746363));
#6667=CARTESIAN_POINT('Ctrl Pts',(-4.06087359175116,0.459129608727532,59.5921523867466));
#6668=CARTESIAN_POINT('Ctrl Pts',(-4.07254533364047,0.340280099194447,59.597984698857));
#6669=CARTESIAN_POINT('Ctrl Pts',(-4.07899969437103,0.221328925631193,59.6038170109674));
#6670=CARTESIAN_POINT('Ctrl Pts',(-4.080356167837,0.196329685982205,59.6050427522845));
#6671=CARTESIAN_POINT('Ctrl Pts',(-4.0814823787454,0.171325945607201,59.6062684936016));
#6672=CARTESIAN_POINT('Ctrl Pts',(-4.0823785710486,0.146322256144288,59.6074942349187));
#6673=CARTESIAN_POINT('Ctrl Pts',(-4.08411401076354,0.0979036348743599,
59.6098678328109));
#6674=CARTESIAN_POINT('Ctrl Pts',(-4.08498814701933,0.0494523315283915,
59.6122414307032));
#6675=CARTESIAN_POINT('Ctrl Pts',(-4.0849998802783,0.000989002666605911,
59.6146150285954));
#6676=CARTESIAN_POINT('Ctrl Pts',(-4.09175882131913,0.000965923615931607,
59.6146162370882));
#6677=CARTESIAN_POINT('Ctrl Pts',(-4.08719829507769,-1.28836881771013,59.6776598638786));
#6678=CARTESIAN_POINT('Ctrl Pts',(-3.41121669487228,-2.60606765915847,59.7419022275068));
#6679=CARTESIAN_POINT('Ctrl Pts',(-2.3368437494292,-3.35778115892392,59.806144591135));
#6680=CARTESIAN_POINT('Ctrl Pts',(-2.31666171942481,-3.3716102527404,59.8073433279728));
#6681=CARTESIAN_POINT('',(-4.08499993153545,0.000747900661492352,59.5103849713657));
#6682=CARTESIAN_POINT('Ctrl Pts',(-4.08499993153559,0.000747899860698453,
59.5103849714045));
#6683=CARTESIAN_POINT('Ctrl Pts',(-4.08502251884219,-0.122623089693615,
59.5163621312386));
#6684=CARTESIAN_POINT('Ctrl Pts',(-4.07945188006652,-0.245929705076146,
59.5223392910726));
#6685=CARTESIAN_POINT('Ctrl Pts',(-4.06833157303784,-0.368650528039084,
59.5283164509067));
#6686=CARTESIAN_POINT('Ctrl Pts',(-4.05720221521403,-0.491471233228483,
59.5342984755389));
#6687=CARTESIAN_POINT('Ctrl Pts',(-4.04051422026161,-0.613704825425184,
59.5402805001711));
#6688=CARTESIAN_POINT('Ctrl Pts',(-4.01836273482416,-0.73483735028681,59.5462625248033));
#6689=CARTESIAN_POINT('Ctrl Pts',(-3.9961705780107,-0.856192281292652,59.5522555327699));
#6690=CARTESIAN_POINT('Ctrl Pts',(-3.96849495158413,-0.976441738099162,
59.5582485407366));
#6691=CARTESIAN_POINT('Ctrl Pts',(-3.93548191022,-1.09508316320322,59.5642415487032));
#6692=CARTESIAN_POINT('Ctrl Pts',(-3.90243773520088,-1.21383647564159,59.5702402085042));
#6693=CARTESIAN_POINT('Ctrl Pts',(-3.86404622307644,-1.3309783788317,59.5762388683053));
#6694=CARTESIAN_POINT('Ctrl Pts',(-3.82050237163993,-1.4460244217487,59.5822375281063));
#6695=CARTESIAN_POINT('Ctrl Pts',(-3.77686641892775,-1.56131380297785,59.5882488759035));
#6696=CARTESIAN_POINT('Ctrl Pts',(-3.72805648758539,-1.67449811914711,59.5942602237007));
#6697=CARTESIAN_POINT('Ctrl Pts',(-3.67431506519386,-1.78511450660438,59.6002715714979));
#6698=CARTESIAN_POINT('Ctrl Pts',(-3.62627846373096,-1.88398861679892,59.6056447958291));
#6699=CARTESIAN_POINT('Ctrl Pts',(-3.57430252124013,-1.98081123881028,59.6110180201603));
#6700=CARTESIAN_POINT('Ctrl Pts',(-3.51858962983403,-2.07527155255028,59.6163912444915));
#6701=CARTESIAN_POINT('Ctrl Pts',(-3.45806815647434,-2.17788473986254,59.6222282320362));
#6702=CARTESIAN_POINT('Ctrl Pts',(-3.39295931187634,-2.27800909715532,59.628065219581));
#6703=CARTESIAN_POINT('Ctrl Pts',(-3.32349327159169,-2.3752089326383,59.6339022071257));
#6704=CARTESIAN_POINT('Ctrl Pts',(-3.25413214706056,-2.47226196554062,59.6397303789679));
#6705=CARTESIAN_POINT('Ctrl Pts',(-3.1804271623573,-2.56639894232262,59.6455585508101));
#6706=CARTESIAN_POINT('Ctrl Pts',(-3.10265341324178,-2.65721034118474,59.6513867226522));
#6707=CARTESIAN_POINT('Ctrl Pts',(-3.02494795657119,-2.74794199935638,59.657209776828));
#6708=CARTESIAN_POINT('Ctrl Pts',(-2.94318110155858,-2.83535357887629,59.6630328310038));
#6709=CARTESIAN_POINT('Ctrl Pts',(-2.85767008583671,-2.91906606306093,59.6688558851796));
#6710=CARTESIAN_POINT('Ctrl Pts',(-2.77221688508832,-3.00272194827978,59.674675002322));
#6711=CARTESIAN_POINT('Ctrl Pts',(-2.68302484836093,-3.08268342973667,59.6804941194644));
#6712=CARTESIAN_POINT('Ctrl Pts',(-2.59044974432747,-3.15860651587275,59.6863132366068));
#6713=CARTESIAN_POINT('Ctrl Pts',(-2.50112581472979,-3.23186323507023,59.6919279903289));
#6714=CARTESIAN_POINT('Ctrl Pts',(-2.40865271670227,-3.30136019072068,59.697542744051));
#6715=CARTESIAN_POINT('Ctrl Pts',(-2.31338095599003,-3.36682247118298,59.7031574977731));
#6716=CARTESIAN_POINT('Ctrl Pts',(-2.31338095599002,-3.36682247118298,58.4531830718678));
#6717=CARTESIAN_POINT('Ctrl Pts',(-2.21522106941994,-3.434269214864,58.4590037287315));
#6718=CARTESIAN_POINT('Ctrl Pts',(-2.11397617042823,-3.49751096136364,58.4648243855952));
#6719=CARTESIAN_POINT('Ctrl Pts',(-2.01004239296545,-3.55625569644278,58.470645042459));
#6720=CARTESIAN_POINT('Ctrl Pts',(-1.90621654655831,-3.61493942747276,58.4764596548042));
#6721=CARTESIAN_POINT('Ctrl Pts',(-1.79970772942948,-3.66913523793015,58.4822742671494));
#6722=CARTESIAN_POINT('Ctrl Pts',(-1.69094135890495,-3.71859413229579,58.4880888794947));
#6723=CARTESIAN_POINT('Ctrl Pts',(-1.58225969137649,-3.76801451000858,58.4938989636472));
#6724=CARTESIAN_POINT('Ctrl Pts',(-1.4713243386094,-3.8127051437847,58.4997090477997));
#6725=CARTESIAN_POINT('Ctrl Pts',(-1.35858511553482,-3.85246304120458,58.5055191319523));
#6726=CARTESIAN_POINT('Ctrl Pts',(-1.24589412383802,-3.89220392965351,58.5113267304715));
#6727=CARTESIAN_POINT('Ctrl Pts',(-1.13140118013004,-3.92701614223388,58.5171343289908));
#6728=CARTESIAN_POINT('Ctrl Pts',(-1.01557543709463,-3.95674506780132,58.52294192751));
#6729=CARTESIAN_POINT('Ctrl Pts',(-0.899772102726297,-3.98646824174931,
58.5287484024402));
#6730=CARTESIAN_POINT('Ctrl Pts',(-0.78263687664277,-4.01110998312592,58.5345548773704));
#6731=CARTESIAN_POINT('Ctrl Pts',(-0.664652793827197,-4.03056592349731,
58.5403613523005));
#6732=CARTESIAN_POINT('Ctrl Pts',(-0.546663784263447,-4.05002267630472,
58.5461680696959));
#6733=CARTESIAN_POINT('Ctrl Pts',(-0.427826249896556,-4.06429313134262,
58.5519747870913));
#6734=CARTESIAN_POINT('Ctrl Pts',(-0.308631476980936,-4.07332439309915,
58.5577815044867));
#6735=CARTESIAN_POINT('Ctrl Pts',(-0.189403689256998,-4.08235815635276,
58.5635898302384));
#6736=CARTESIAN_POINT('Ctrl Pts',(-0.0698188726936143,-4.0861498095383,
58.5693981559901));
#6737=CARTESIAN_POINT('Ctrl Pts',(0.0496291692062076,-4.08469851342347,
58.5752064817418));
#6738=CARTESIAN_POINT('Ctrl Pts',(0.169205615726446,-4.08324565718991,58.5810210513452));
#6739=CARTESIAN_POINT('Ctrl Pts',(0.288644585880642,-4.07653860439837,58.5868356209487));
#6740=CARTESIAN_POINT('Ctrl Pts',(0.407454694668163,-4.06462860195035,58.5926501905521));
#6741=CARTESIAN_POINT('Ctrl Pts',(0.526337680284906,-4.0527112940363,58.5984683267493));
#6742=CARTESIAN_POINT('Ctrl Pts',(0.644590633258377,-4.03558473806075,58.6042864629465));
#6743=CARTESIAN_POINT('Ctrl Pts',(0.761731344424355,-4.01335151200608,58.6101045991437));
#6744=CARTESIAN_POINT('Ctrl Pts',(0.879043461512295,-3.99108575322583,58.6159312487176));
#6745=CARTESIAN_POINT('Ctrl Pts',(0.995239691297029,-3.96369849841228,58.6217578982915));
#6746=CARTESIAN_POINT('Ctrl Pts',(1.10985173705642,-3.93134253426903,58.6275845478654));
#6747=CARTESIAN_POINT('Ctrl Pts',(1.15930477629944,-3.91738151687404,58.6300986425064));
#6748=CARTESIAN_POINT('Ctrl Pts',(1.20846311401074,-3.90249605722148,58.6326127371474));
#6749=CARTESIAN_POINT('Ctrl Pts',(1.25729032293254,-3.88670117758752,58.6351268317883));
#6750=CARTESIAN_POINT('Ctrl Pts',(1.37045573134724,-3.850093842372,58.6409536761466));
#6751=CARTESIAN_POINT('Ctrl Pts',(1.48220101786181,-3.80848178787127,58.6467805205049));
#6752=CARTESIAN_POINT('Ctrl Pts',(1.59205196469652,-3.7619935594982,58.6526073648632));
#6753=CARTESIAN_POINT('Ctrl Pts',(1.70176552280632,-3.71556347316763,58.6584269216856));
#6754=CARTESIAN_POINT('Ctrl Pts',(1.80958908142062,-3.66426950082316,58.664246478508));
#6755=CARTESIAN_POINT('Ctrl Pts',(1.91506372861185,-3.60828988793241,58.6700660353305));
#6756=CARTESIAN_POINT('Ctrl Pts',(2.02043385696985,-3.55236574736586,58.675879825333));
#6757=CARTESIAN_POINT('Ctrl Pts',(2.12345934641995,-3.49176539371288,58.6816936153356));
#6758=CARTESIAN_POINT('Ctrl Pts',(2.22370197573578,-3.42671482955743,58.6875074053382));
#6759=CARTESIAN_POINT('Ctrl Pts',(2.32706354174668,-3.35964029024326,58.6935020848795));
#6760=CARTESIAN_POINT('Ctrl Pts',(2.42746583767444,-3.28783425661528,58.6994967644208));
#6761=CARTESIAN_POINT('Ctrl Pts',(2.52445626156305,-3.21159548876491,58.705491443962));
#6762=CARTESIAN_POINT('Ctrl Pts',(2.61841597281109,-3.13773899524804,58.7112988044842));
#6763=CARTESIAN_POINT('Ctrl Pts',(2.70917351844038,-3.05972293732472,58.7171061650065));
#6764=CARTESIAN_POINT('Ctrl Pts',(2.79634807355528,-2.97786206052659,58.7229135255287));
#6765=CARTESIAN_POINT('Ctrl Pts',(2.88351016067287,-2.89601289174568,58.7287200554627));
#6766=CARTESIAN_POINT('Ctrl Pts',(2.96708997926215,-2.81032027680275,58.7345265853967));
#6767=CARTESIAN_POINT('Ctrl Pts',(3.0467418741869,-2.72113743718984,58.7403331153308));
#6768=CARTESIAN_POINT('Ctrl Pts',(3.12640111095747,-2.63194637722438,58.7461401804768));
#6769=CARTESIAN_POINT('Ctrl Pts',(3.20213143257101,-2.53926475710069,58.7519472456228));
#6770=CARTESIAN_POINT('Ctrl Pts',(3.27362638703625,-2.44348015709152,58.7577543107688));
#6771=CARTESIAN_POINT('Ctrl Pts',(3.34514474677619,-2.34766420011609,58.7635632769714));
#6772=CARTESIAN_POINT('Ctrl Pts',(3.41242473802761,-2.24874356957999,58.769372243174));
#6773=CARTESIAN_POINT('Ctrl Pts',(3.4752026518956,-2.14713565669656,58.7751812093766));
#6774=CARTESIAN_POINT('Ctrl Pts',(3.53804953997439,-2.04541610701017,58.7809965579011));
#6775=CARTESIAN_POINT('Ctrl Pts',(3.59638426302548,-1.94100372876592,58.7868119064257));
#6776=CARTESIAN_POINT('Ctrl Pts',(3.64998851774923,-1.83434152226318,58.7926272549503));
#6777=CARTESIAN_POINT('Ctrl Pts',(3.70362807252076,-1.72760907542214,58.7984464330604));
#6778=CARTESIAN_POINT('Ctrl Pts',(3.75253078833386,-1.61862422079623,58.8042656111706));
#6779=CARTESIAN_POINT('Ctrl Pts',(3.79652669891199,-1.50784947008926,58.8100847892808));
#6780=CARTESIAN_POINT('Ctrl Pts',(3.84058450163022,-1.39691888475353,58.8159121536378));
#6781=CARTESIAN_POINT('Ctrl Pts',(3.87972158923193,-1.28419376169753,58.8217395179949));
#6782=CARTESIAN_POINT('Ctrl Pts',(3.91381792787329,-1.17015136946363,58.8275668823519));
#6783=CARTESIAN_POINT('Ctrl Pts',(3.92125431490904,-1.14527880540173,58.8288378263443));
#6784=CARTESIAN_POINT('Ctrl Pts',(3.9284511208704,-1.12034361763696,58.8301087703366));
#6785=CARTESIAN_POINT('Ctrl Pts',(3.93540742551294,-1.09535080920115,58.831379714329));
#6786=CARTESIAN_POINT('Ctrl Pts',(3.96729404086616,-0.980787674010631,58.8372055233328));
#6787=CARTESIAN_POINT('Ctrl Pts',(3.99422479012238,-0.864648383214477,58.8430313323366));
#6788=CARTESIAN_POINT('Ctrl Pts',(4.01604524613472,-0.747399211264446,58.8488571413404));
#6789=CARTESIAN_POINT('Ctrl Pts',(4.03783839578895,-0.630296766214877,58.8546756598628));
#6790=CARTESIAN_POINT('Ctrl Pts',(4.05453389821043,-0.512087600206339,58.8604941783853));
#6791=CARTESIAN_POINT('Ctrl Pts',(4.06602722001259,-0.393252649217582,58.8663126969078));
#6792=CARTESIAN_POINT('Ctrl Pts',(4.07750914731762,-0.274535511384376,58.8721254469419));
#6793=CARTESIAN_POINT('Ctrl Pts',(4.08379911534598,-0.155194226590116,58.877938196976));
#6794=CARTESIAN_POINT('Ctrl Pts',(4.08484383610604,-0.035718827339529,58.8837509470102));
#6795=CARTESIAN_POINT('Ctrl Pts',(4.08592132485717,0.0875039549122769,58.8897460157543));
#6796=CARTESIAN_POINT('Ctrl Pts',(4.08141902440324,0.210868969000254,58.8957410844985));
#6797=CARTESIAN_POINT('Ctrl Pts',(4.07133640056975,0.333833661268243,58.9017361532426));
#6798=CARTESIAN_POINT('Ctrl Pts',(4.06157121290607,0.452926996081961,58.9075424763099));
#6799=CARTESIAN_POINT('Ctrl Pts',(4.04657184074196,0.571644401307267,58.9133487993772));
#6800=CARTESIAN_POINT('Ctrl Pts',(4.02639068993385,0.689494751259203,58.9191551224445));
#6801=CARTESIAN_POINT('Ctrl Pts',(4.00621241647675,0.807328298560677,58.9249606176685));
#6802=CARTESIAN_POINT('Ctrl Pts',(3.98085390252483,0.924294634459594,58.9307661128925));
#6803=CARTESIAN_POINT('Ctrl Pts',(3.95041904743944,1.03991074118293,58.9365716081166));
#6804=CARTESIAN_POINT('Ctrl Pts',(3.91998136621631,1.15553758385502,58.9423776424307));
#6805=CARTESIAN_POINT('Ctrl Pts',(3.88446651049147,1.26981355354743,58.9481836767449));
#6806=CARTESIAN_POINT('Ctrl Pts',(3.84402866362447,1.38226937795551,58.953989711059));
#6807=CARTESIAN_POINT('Ctrl Pts',(3.8035775413578,1.49476212065002,58.9597976514446));
#6808=CARTESIAN_POINT('Ctrl Pts',(3.75820035165562,1.60543314600411,58.9656055918302));
#6809=CARTESIAN_POINT('Ctrl Pts',(3.70809972046971,1.71383239059496,58.9714135322158));
#6810=CARTESIAN_POINT('Ctrl Pts',(3.65794392604076,1.8223509880509,58.9772278674276));
#6811=CARTESIAN_POINT('Ctrl Pts',(3.60305448060662,1.92859244153204,58.9830422026393));
#6812=CARTESIAN_POINT('Ctrl Pts',(3.54368041622873,2.03213043568491,58.9888565378511));
#6813=CARTESIAN_POINT('Ctrl Pts',(3.48426718240505,2.13573673450739,58.9946747088166));
#6814=CARTESIAN_POINT('Ctrl Pts',(3.4203636553121,2.23663567827114,59.0004928797821));
#6815=CARTESIAN_POINT('Ctrl Pts',(3.35226180162721,2.33443051157046,59.0063110507475));
#6816=CARTESIAN_POINT('Ctrl Pts',(3.28406393522339,2.43236321993974,59.0121374244033));
#6817=CARTESIAN_POINT('Ctrl Pts',(3.21165617573436,2.52718276057776,59.0179637980591));
#6818=CARTESIAN_POINT('Ctrl Pts',(3.13537033821866,2.6185258910728,59.0237901717148));
#6819=CARTESIAN_POINT('Ctrl Pts',(3.11860046623421,2.63860579915201,59.0250709800998));
#6820=CARTESIAN_POINT('Ctrl Pts',(3.10164332450812,2.65851785412056,59.0263517884847));
#6821=CARTESIAN_POINT('Ctrl Pts',(3.0845026659662,2.67825844601439,59.0276325968696));
#6822=CARTESIAN_POINT('Ctrl Pts',(3.00651290656505,2.7680778662234,59.0334602573142));
#6823=CARTESIAN_POINT('Ctrl Pts',(2.92447268937666,2.85463067025238,59.0392879177588));
#6824=CARTESIAN_POINT('Ctrl Pts',(2.83868600491129,2.9375307258854,59.0451155782034));
#6825=CARTESIAN_POINT('Ctrl Pts',(2.75300667715892,3.02032703724229,59.0509359456925));
#6826=CARTESIAN_POINT('Ctrl Pts',(2.66359049839989,3.09947941171397,59.0567563131816));
#6827=CARTESIAN_POINT('Ctrl Pts',(2.57078120099155,3.17463525725845,59.0625766806707));
#6828=CARTESIAN_POINT('Ctrl Pts',(2.47806395968989,3.24971655688213,59.0683912750273));
#6829=CARTESIAN_POINT('Ctrl Pts',(2.38196061045916,3.32080895886833,59.074205869384));
#6830=CARTESIAN_POINT('Ctrl Pts',(2.28285073276569,3.38759760477999,59.0800204637406));
#6831=CARTESIAN_POINT('Ctrl Pts',(2.18067647926323,3.45645128715029,59.0860148393935));
#6832=CARTESIAN_POINT('Ctrl Pts',(2.07530707447446,3.52073044491613,59.0920092150464));
#6833=CARTESIAN_POINT('Ctrl Pts',(1.96719442957651,3.5801356226047,59.0980035906993));
#6834=CARTESIAN_POINT('Ctrl Pts',(1.86244059479987,3.63769521865695,59.1038117349485));
#6835=CARTESIAN_POINT('Ctrl Pts',(1.75511183269771,3.69067898844718,59.1096198791978));
#6836=CARTESIAN_POINT('Ctrl Pts',(1.64564691528913,3.73885961627331,59.115428023447));
#6837=CARTESIAN_POINT('Ctrl Pts',(1.53619782095155,3.78703327962613,59.1212353281334));
#6838=CARTESIAN_POINT('Ctrl Pts',(1.42461355843513,3.83040501766096,59.1270426328197));
#6839=CARTESIAN_POINT('Ctrl Pts',(1.31135454404858,3.86879493638564,59.1328499375061));
#6840=CARTESIAN_POINT('Ctrl Pts',(1.19808528248824,3.90718832846005,59.1386577676117));
#6841=CARTESIAN_POINT('Ctrl Pts',(1.08314135388968,3.94059887419651,59.1444655977172));
#6842=CARTESIAN_POINT('Ctrl Pts',(0.966999453192039,3.96889620140491,59.1502734278228));
#6843=CARTESIAN_POINT('Ctrl Pts',(0.850819748518538,3.99720273934145,59.1560831483664));
#6844=CARTESIAN_POINT('Ctrl Pts',(0.733441692089495,4.0203926522191,59.1618928689101));
#6845=CARTESIAN_POINT('Ctrl Pts',(0.615352688683319,4.03838656749576,59.1677025894537));
#6846=CARTESIAN_POINT('Ctrl Pts',(0.49713435044164,4.05640019028121,59.1735186729882));
#6847=CARTESIAN_POINT('Ctrl Pts',(0.37820391423102,4.06920639500047,59.1793347565227));
#6848=CARTESIAN_POINT('Ctrl Pts',(0.259054585734492,4.07677761493191,59.1851508400572));
#6849=CARTESIAN_POINT('Ctrl Pts',(0.139827018305857,4.08435380647477,59.1909707426998));
#6850=CARTESIAN_POINT('Ctrl Pts',(0.0203806789546916,4.08668815908609,59.1967906453424));
#6851=CARTESIAN_POINT('Ctrl Pts',(-0.0987921802569579,4.08380522370008,
59.202610547985));
#6852=CARTESIAN_POINT('Ctrl Pts',(-0.218132247600786,4.08091824334742,59.2084386163715));
#6853=CARTESIAN_POINT('Ctrl Pts',(-0.337197663778942,4.07279939271625,59.214266684758));
#6854=CARTESIAN_POINT('Ctrl Pts',(-0.455502130741042,4.059524948672,59.2200947531445));
#6855=CARTESIAN_POINT('Ctrl Pts',(-0.481151558105484,4.0566469348737,59.2213583285664));
#6856=CARTESIAN_POINT('Ctrl Pts',(-0.506765259176913,4.05352676730336,59.2226219039883));
#6857=CARTESIAN_POINT('Ctrl Pts',(-0.53233835602326,4.0501655367042,59.2238854794102));
#6858=CARTESIAN_POINT('Ctrl Pts',(-0.650283495193144,4.03466327613791,59.2297131888927));
#6859=CARTESIAN_POINT('Ctrl Pts',(-0.767737928515811,4.01398013173085,59.2355408983752));
#6860=CARTESIAN_POINT('Ctrl Pts',(-0.884211867592764,3.98815676387076,59.2413686078577));
#6861=CARTESIAN_POINT('Ctrl Pts',(-1.00054039203771,3.96236563580238,59.2471890415991));
#6862=CARTESIAN_POINT('Ctrl Pts',(-1.11589046253476,3.93144713644343,59.2530094753404));
#6863=CARTESIAN_POINT('Ctrl Pts',(-1.22977835674899,3.89549357505204,59.2588299090818));
#6864=CARTESIAN_POINT('Ctrl Pts',(-1.34355361914526,3.85957557068812,59.2646445865833));
#6865=CARTESIAN_POINT('Ctrl Pts',(-1.455869195571,3.81863253291981,59.2704592640848));
#6866=CARTESIAN_POINT('Ctrl Pts',(-1.56625307524593,3.77280748306651,59.2762739415864));
#6867=CARTESIAN_POINT('Ctrl Pts',(-1.68004781323775,3.72556644065275,59.2822682924349));
#6868=CARTESIAN_POINT('Ctrl Pts',(-1.79178910556303,3.67313687184631,59.2882626432834));
#6869=CARTESIAN_POINT('Ctrl Pts',(-1.90097793319669,3.61573061738554,59.2942569941319));
#6870=CARTESIAN_POINT('Ctrl Pts',(-2.00677721407015,3.56010642422207,59.3000652624577));
#6871=CARTESIAN_POINT('Ctrl Pts',(-2.11017977211938,3.49981016210914,59.3058735307836));
#6872=CARTESIAN_POINT('Ctrl Pts',(-2.21075398360769,3.43508250613617,59.3116817991094));
#6873=CARTESIAN_POINT('Ctrl Pts',(-2.31131391457538,3.37036404083555,59.3174892427198));
#6874=CARTESIAN_POINT('Ctrl Pts',(-2.40904595500098,3.30121565361789,59.3232966863303));
#6875=CARTESIAN_POINT('Ctrl Pts',(-2.50354610561273,3.22792222599482,59.3291041299408));
#6876=CARTESIAN_POINT('Ctrl Pts',(-2.59805504383908,3.15462198278055,59.3349121135882));
#6877=CARTESIAN_POINT('Ctrl Pts',(-2.68933117259142,3.07717618261264,59.3407200972356));
#6878=CARTESIAN_POINT('Ctrl Pts',(-2.7770028274467,2.99591059552067,59.3465280808831));
#6879=CARTESIAN_POINT('Ctrl Pts',(-2.86470323586026,2.91461835586011,59.3523379693674));
#6880=CARTESIAN_POINT('Ctrl Pts',(-2.94879652047481,2.82950411467823,59.3581478578516));
#6881=CARTESIAN_POINT('Ctrl Pts',(-3.02894765507416,2.74093070011278,59.3639577463359));
#6882=CARTESIAN_POINT('Ctrl Pts',(-3.10918684988492,2.65225997197029,59.3697740180112));
#6883=CARTESIAN_POINT('Ctrl Pts',(-3.18547497594834,2.56012278692757,59.3755902896866));
#6884=CARTESIAN_POINT('Ctrl Pts',(-3.25751702354118,2.46491538218646,59.381406561362));
#6885=CARTESIAN_POINT('Ctrl Pts',(-3.32960652458181,2.36964526518547,59.3872266641631));
#6886=CARTESIAN_POINT('Ctrl Pts',(-3.39744414603443,2.27130123557681,59.3930467669642));
#6887=CARTESIAN_POINT('Ctrl Pts',(-3.46077888069734,2.17030747566313,59.3988668697653));
#6888=CARTESIAN_POINT('Ctrl Pts',(-3.52420264704673,2.06917174555227,59.4046951540733));
#6889=CARTESIAN_POINT('Ctrl Pts',(-3.583110692876,1.96537920425242,59.4105234383813));
#6890=CARTESIAN_POINT('Ctrl Pts',(-3.63729844346071,1.85937759295907,59.4163517226893));
#6891=CARTESIAN_POINT('Ctrl Pts',(-3.6490337131111,1.83642115947586,59.4176139357765));
#6892=CARTESIAN_POINT('Ctrl Pts',(-3.66054777696709,1.81336118679001,59.4188761488637));
#6893=CARTESIAN_POINT('Ctrl Pts',(-3.67183886052013,1.79020233001028,59.4201383619509));
#6894=CARTESIAN_POINT('Ctrl Pts',(-3.72759460119396,1.67584313615196,59.4263712115471));
#6895=CARTESIAN_POINT('Ctrl Pts',(-3.77806724379518,1.55874737083152,59.4326040611434));
#6896=CARTESIAN_POINT('Ctrl Pts',(-3.82299955405977,1.43940939612703,59.4388369107396));
#6897=CARTESIAN_POINT('Ctrl Pts',(-3.86779625853553,1.32043158363325,59.4450509495851));
#6898=CARTESIAN_POINT('Ctrl Pts',(-3.9070858607795,1.19922535306526,59.4512649884307));
#6899=CARTESIAN_POINT('Ctrl Pts',(-3.94065870003593,1.07630572321767,59.4574790272762));
#6900=CARTESIAN_POINT('Ctrl Pts',(-3.97416997482929,0.953611498226502,59.4636816710782));
#6901=CARTESIAN_POINT('Ctrl Pts',(-4.00198528966692,0.829210439627046,59.4698843148802));
#6902=CARTESIAN_POINT('Ctrl Pts',(-4.02394358429263,0.703635580702222,59.4760869586822));
#6903=CARTESIAN_POINT('Ctrl Pts',(-4.04584137768624,0.578406715572335,59.4822725124689));
#6904=CARTESIAN_POINT('Ctrl Pts',(-4.06191427259615,0.452010811417527,59.4884580662555));
#6905=CARTESIAN_POINT('Ctrl Pts',(-4.07205165169264,0.324992839839935,59.4946436200422));
#6906=CARTESIAN_POINT('Ctrl Pts',(-4.08065104588121,0.217245305074713,59.49989073715));
#6907=CARTESIAN_POINT('Ctrl Pts',(-4.08498010299262,0.109050513921404,59.5051378542579));
#6908=CARTESIAN_POINT('Ctrl Pts',(-4.08499993153545,0.00074790066148241,
59.5103849713657));
#6909=CARTESIAN_POINT('Origin',(0.,0.,46.4896150285955));
#6910=CARTESIAN_POINT('',(-2.31338095599003,-3.36682247118298,57.2030181077425));
#6911=CARTESIAN_POINT('',(-2.31338095599002,-3.36682247118298,57.3074490595572));
#6912=CARTESIAN_POINT('',(-2.31338095599002,-3.36682247118298,46.4896150285955));
#6913=CARTESIAN_POINT('',(-4.08499891745875,-0.00297394700961989,58.3646150286342));
#6914=CARTESIAN_POINT('Ctrl Pts',(-2.31338095599002,-3.36682247118298,57.3074490595572));
#6915=CARTESIAN_POINT('Ctrl Pts',(-2.2136460283599,-3.43535144299583,57.3133350373661));
#6916=CARTESIAN_POINT('Ctrl Pts',(-2.11079358198057,-3.49949301292074,57.3192210151751));
#6917=CARTESIAN_POINT('Ctrl Pts',(-2.00524962729991,-3.55896037238595,57.325106992984));
#6918=CARTESIAN_POINT('Ctrl Pts',(-1.90112271487449,-3.61762931794462,57.3309139451463));
#6919=CARTESIAN_POINT('Ctrl Pts',(-1.79437649443802,-3.67174859926997,57.3367208973086));
#6920=CARTESIAN_POINT('Ctrl Pts',(-1.68544775461599,-3.72108732314359,57.3425278494708));
#6921=CARTESIAN_POINT('Ctrl Pts',(-1.57653124128274,-3.77042050909071,57.3483341498434));
#6922=CARTESIAN_POINT('Ctrl Pts',(-1.46543306721513,-3.81497403657739,57.3541404502159));
#6923=CARTESIAN_POINT('Ctrl Pts',(-1.35261202454224,-3.85456426993555,57.3599467505885));
#6924=CARTESIAN_POINT('Ctrl Pts',(-1.23977710421394,-3.89415937312652,57.3657537651703));
#6925=CARTESIAN_POINT('Ctrl Pts',(-1.12521927870738,-3.92878983321132,57.3715607797521));
#6926=CARTESIAN_POINT('Ctrl Pts',(-1.00941399117484,-3.95832141120709,57.3773677943339));
#6927=CARTESIAN_POINT('Ctrl Pts',(-0.890849090619016,-3.98855671982666,
57.3833131887204));
#6928=CARTESIAN_POINT('Ctrl Pts',(-0.770976956570396,-4.01344694300943,
57.3892585831069));
#6929=CARTESIAN_POINT('Ctrl Pts',(-0.650319266757598,-4.03290340217614,
57.3952039774934));
#6930=CARTESIAN_POINT('Ctrl Pts',(-0.532294865405861,-4.05193523470284,
57.4010196168807));
#6931=CARTESIAN_POINT('Ctrl Pts',(-0.413519261976091,-4.06576806349613,
57.4068352562681));
#6932=CARTESIAN_POINT('Ctrl Pts',(-0.294485206654571,-4.07437154209844,
57.4126508956554));
#6933=CARTESIAN_POINT('Ctrl Pts',(-0.171467428466069,-4.08326295405185,
57.4186611675415));
#6934=CARTESIAN_POINT('Ctrl Pts',(-0.0481740771729017,-4.08656885330446,
57.4246714394275));
#6935=CARTESIAN_POINT('Ctrl Pts',(0.0748529556290137,-4.08431414499835,
57.4306817113135));
#6936=CARTESIAN_POINT('Ctrl Pts',(0.197879988430929,-4.08205943669224,57.4366919831996));
#6937=CARTESIAN_POINT('Ctrl Pts',(0.320640233957287,-4.07424421589866,57.4427022550856));
#6938=CARTESIAN_POINT('Ctrl Pts',(0.442600890991567,-4.06095179130379,57.4487125269716));
#6939=CARTESIAN_POINT('Ctrl Pts',(0.560835448643127,-4.048065472221,57.4545391751309));
#6940=CARTESIAN_POINT('Ctrl Pts',(0.67869492964639,-4.02999076694206,57.4603658232901));
#6941=CARTESIAN_POINT('Ctrl Pts',(0.795688927702892,-4.00675730863887,57.4661924714494));
#6942=CARTESIAN_POINT('Ctrl Pts',(0.912536563359301,-3.98355291596962,57.4720118303269));
#6943=CARTESIAN_POINT('Ctrl Pts',(1.02852047313209,-3.9552026857757,57.4778311892045));
#6944=CARTESIAN_POINT('Ctrl Pts',(1.14315515176311,-3.92178802321052,57.483650548082));
#6945=CARTESIAN_POINT('Ctrl Pts',(1.25767620141708,-3.8884064821577,57.4894641386545));
#6946=CARTESIAN_POINT('Ctrl Pts',(1.37085029127783,-3.84997060923041,57.495277729227));
#6947=CARTESIAN_POINT('Ctrl Pts',(1.48220248464921,-3.80661277180904,57.5010913197995));
#6948=CARTESIAN_POINT('Ctrl Pts',(1.59702463614523,-3.76190381703945,57.5070860735376));
#6949=CARTESIAN_POINT('Ctrl Pts',(1.70990905028883,-3.71196120252409,57.5130808272756));
#6950=CARTESIAN_POINT('Ctrl Pts',(1.82035187681997,-3.65698565003447,57.5190755810136));
#6951=CARTESIAN_POINT('Ctrl Pts',(1.92733859398976,-3.6037304584553,57.5248827397293));
#6952=CARTESIAN_POINT('Ctrl Pts',(2.03203386317524,-3.54575282016584,57.530689898445));
#6953=CARTESIAN_POINT('Ctrl Pts',(2.13400094306043,-3.48328364837221,57.5364970571606));
#6954=CARTESIAN_POINT('Ctrl Pts',(2.23595342963761,-3.42082341703137,57.5423033847683));
#6955=CARTESIAN_POINT('Ctrl Pts',(2.33517815579904,-3.35387314361274,57.548109712376));
#6956=CARTESIAN_POINT('Ctrl Pts',(2.43126501140071,-3.28270855306083,57.5539160399836));
#6957=CARTESIAN_POINT('Ctrl Pts',(2.52736071919643,-3.21153740632845,57.5597229025109));
#6958=CARTESIAN_POINT('Ctrl Pts',(2.62031765393769,-3.13615141324877,57.5655297650381));
#6959=CARTESIAN_POINT('Ctrl Pts',(2.7097571218915,-3.05686789710617,57.5713366275653));
#6960=CARTESIAN_POINT('Ctrl Pts',(2.79922586962693,-2.97755842593396,57.577145391084));
#6961=CARTESIAN_POINT('Ctrl Pts',(2.88517455542489,-2.89434916448145,57.5829541546028));
#6962=CARTESIAN_POINT('Ctrl Pts',(2.96726029135002,-2.8075952990731,57.5887629181215));
#6963=CARTESIAN_POINT('Ctrl Pts',(3.04943623127523,-2.72074609985805,57.5945780648894));
#6964=CARTESIAN_POINT('Ctrl Pts',(3.12774046780224,-2.63034481823913,57.6003932116572));
#6965=CARTESIAN_POINT('Ctrl Pts',(3.20186937860885,-2.53678092911606,57.6062083584251));
#6966=CARTESIAN_POINT('Ctrl Pts',(3.27604711129668,-2.44315541808285,57.6120273350942));
#6967=CARTESIAN_POINT('Ctrl Pts',(3.34604380321781,-2.34636348092971,57.6178463117633));
#6968=CARTESIAN_POINT('Ctrl Pts',(3.41159920560623,-2.24682350448515,57.6236652884323));
#6969=CARTESIAN_POINT('Ctrl Pts',(3.47724685475701,-2.14714345963711,57.6294924533168));
#6970=CARTESIAN_POINT('Ctrl Pts',(3.53844053296473,-2.04470800660846,57.6353196182014));
#6971=CARTESIAN_POINT('Ctrl Pts',(3.5949658918695,-1.93996011203709,57.6411467830859));
#6972=CARTESIAN_POINT('Ctrl Pts',(3.60731319017287,-1.91707916928886,57.6424196585613));
#6973=CARTESIAN_POINT('Ctrl Pts',(3.61943792153851,-1.8940879618285,57.6436925340368));
#6974=CARTESIAN_POINT('Ctrl Pts',(3.63133816117021,-1.87099122371779,57.6449654095123));
#6975=CARTESIAN_POINT('Ctrl Pts',(3.68581231873255,-1.76526433165857,57.65079208371));
#6976=CARTESIAN_POINT('Ctrl Pts',(3.73575195601721,-1.6569881857762,57.6566187579076));
#6977=CARTESIAN_POINT('Ctrl Pts',(3.78091126622735,-1.54658817948253,57.6624454321053));
#6978=CARTESIAN_POINT('Ctrl Pts',(3.82601408348645,-1.43632628030613,57.6682648173072));
#6979=CARTESIAN_POINT('Ctrl Pts',(3.86634831518234,-1.32394617958235,57.6740842025091));
#6980=CARTESIAN_POINT('Ctrl Pts',(3.90171404063422,-1.20989774159545,57.679903587711));
#6981=CARTESIAN_POINT('Ctrl Pts',(3.9370447123089,-1.0959623460666,57.6857172048584));
#6982=CARTESIAN_POINT('Ctrl Pts',(3.96741655501291,-0.980362290389359,57.6915308220058));
#6983=CARTESIAN_POINT('Ctrl Pts',(3.99267798510178,-0.863566735859806,57.6973444391532));
#6984=CARTESIAN_POINT('Ctrl Pts',(4.0187264501716,-0.743132345891777,57.7033391830241));
#6985=CARTESIAN_POINT('Ctrl Pts',(4.03934068463659,-0.621427152793105,57.7093339268949));
#6986=CARTESIAN_POINT('Ctrl Pts',(4.05441017078938,-0.498982130942181,57.7153286707657));
#6987=CARTESIAN_POINT('Ctrl Pts',(4.0690081764639,-0.38036805839366,57.7211358565022));
#6988=CARTESIAN_POINT('Ctrl Pts',(4.07840316568417,-0.261060195461489,57.7269430422388));
#6989=CARTESIAN_POINT('Ctrl Pts',(4.08254682021603,-0.141550205736202,57.7327502279753));
#6990=CARTESIAN_POINT('Ctrl Pts',(4.08668988180302,-0.022057317542035,57.7385565827205));
#6991=CARTESIAN_POINT('Ctrl Pts',(4.08558308906477,0.0976372324661348,57.7443629374657));
#6992=CARTESIAN_POINT('Ctrl Pts',(4.07923019129494,0.217039273929551,57.7501692922109));
#6993=CARTESIAN_POINT('Ctrl Pts',(4.07287670816039,0.336452317260869,57.7559761819616));
#6994=CARTESIAN_POINT('Ctrl Pts',(4.06127618057952,0.45557239121489,57.7617830717123));
#6995=CARTESIAN_POINT('Ctrl Pts',(4.04448438480129,0.573908582527345,57.767589961463));
#6996=CARTESIAN_POINT('Ctrl Pts',(4.02768709176197,0.692283514481301,57.7733987522604));
#6997=CARTESIAN_POINT('Ctrl Pts',(4.00569520778615,0.809873649868988,57.7792075430579));
#6998=CARTESIAN_POINT('Ctrl Pts',(3.97861584184328,0.926197054105497,57.7850163338553));
#6999=CARTESIAN_POINT('Ctrl Pts',(3.95150671879472,1.04264828437166,57.7908315078451));
#7000=CARTESIAN_POINT('Ctrl Pts',(3.91929904742509,1.15782960765195,57.7966466818349));
#7001=CARTESIAN_POINT('Ctrl Pts',(3.8821501965648,1.27127292557966,57.8024618558247));
#7002=CARTESIAN_POINT('Ctrl Pts',(3.84497687931187,1.38479095776354,57.8082808597131));
#7003=CARTESIAN_POINT('Ctrl Pts',(3.80285604487924,1.49656832421439,57.8140998636015));
#7004=CARTESIAN_POINT('Ctrl Pts',(3.7559931034746,1.60615715502912,57.8199188674898));
#7005=CARTESIAN_POINT('Ctrl Pts',(3.70906422052781,1.71590018991832,57.8257460593851));
#7006=CARTESIAN_POINT('Ctrl Pts',(3.65738008911337,1.82344817681897,57.8315732512805));
#7007=CARTESIAN_POINT('Ctrl Pts',(3.60119194136111,1.92837797163206,57.8374004431758));
#7008=CARTESIAN_POINT('Ctrl Pts',(3.5889208588993,1.95129387500959,57.8386730594681));
#7009=CARTESIAN_POINT('Ctrl Pts',(3.57643511834042,1.97408501456058,57.8399456757605));
#7010=CARTESIAN_POINT('Ctrl Pts',(3.56373760472143,1.99674717595753,57.8412182920529));
#7011=CARTESIAN_POINT('Ctrl Pts',(3.50560341422508,2.10050342676706,57.8470448278764));
#7012=CARTESIAN_POINT('Ctrl Pts',(3.44284171951916,2.20188391439461,57.8528713636999));
#7013=CARTESIAN_POINT('Ctrl Pts',(3.37567171959562,2.30044896520709,57.8586978995233));
#7014=CARTESIAN_POINT('Ctrl Pts',(3.30858575265101,2.39889070628534,57.8645171460634));
#7015=CARTESIAN_POINT('Ctrl Pts',(3.23710267775894,2.49452368234317,57.8703363926036));
#7016=CARTESIAN_POINT('Ctrl Pts',(3.16148741778965,2.58693299239809,57.8761556391437));
#7017=CARTESIAN_POINT('Ctrl Pts',(3.0859471094282,2.67925070419134,57.881969117511));
#7018=CARTESIAN_POINT('Ctrl Pts',(3.00628302140393,2.76835079313342,57.8877825958784));
#7019=CARTESIAN_POINT('Ctrl Pts',(2.92280283701968,2.85384802957511,57.8935960742457));
#7020=CARTESIAN_POINT('Ctrl Pts',(2.83671897618786,2.94201185261453,57.8995908700935));
#7021=CARTESIAN_POINT('Ctrl Pts',(2.74657732364043,3.02634403411968,57.9055856659414));
#7022=CARTESIAN_POINT('Ctrl Pts',(2.65275981030388,3.10645946196575,57.9115804617892));
#7023=CARTESIAN_POINT('Ctrl Pts',(2.56188052521919,3.18406579097584,57.9173875093382));
#7024=CARTESIAN_POINT('Ctrl Pts',(2.46755252109992,3.25771526527268,57.9231945568873));
#7025=CARTESIAN_POINT('Ctrl Pts',(2.37015921714246,3.32709637452759,57.9290016044364));
#7026=CARTESIAN_POINT('Ctrl Pts',(2.27277984248461,3.39646756081842,57.9348078214549));
#7027=CARTESIAN_POINT('Ctrl Pts',(2.17233637196149,3.46157135960054,57.9406140384735));
#7028=CARTESIAN_POINT('Ctrl Pts',(2.06924303801145,3.52213830643278,57.9464202554921));
#7029=CARTESIAN_POINT('Ctrl Pts',(1.96614019381764,3.58271084049754,57.9522270081277));
#7030=CARTESIAN_POINT('Ctrl Pts',(1.86038735182497,3.63874548390321,57.9580337607633));
#7031=CARTESIAN_POINT('Ctrl Pts',(1.75242472752776,3.69001796396024,57.9638405133988));
#7032=CARTESIAN_POINT('Ctrl Pts',(1.64442674365151,3.74130723661862,57.9696491678438));
#7033=CARTESIAN_POINT('Ctrl Pts',(1.53421790628161,3.78783106914006,57.9754578222887));
#7034=CARTESIAN_POINT('Ctrl Pts',(1.42225925843097,3.82941295785756,57.9812664767336));
#7035=CARTESIAN_POINT('Ctrl Pts',(1.31017754328291,3.87104055426057,57.9870815161735));
#7036=CARTESIAN_POINT('Ctrl Pts',(1.19634256096252,3.90771522184106,57.9928965556134));
#7037=CARTESIAN_POINT('Ctrl Pts',(1.08123153847864,3.93931001067434,57.9987115950533));
#7038=CARTESIAN_POINT('Ctrl Pts',(0.966044683761101,3.97092561335636,58.0045304652943));
#7039=CARTESIAN_POINT('Ctrl Pts',(0.849580511417873,3.99745458213876,58.0103493355353));
#7040=CARTESIAN_POINT('Ctrl Pts',(0.732325876425768,4.01882119665919,58.0161682057763));
#7041=CARTESIAN_POINT('Ctrl Pts',(0.614906200508081,4.04021788560558,58.0219952663266));
#7042=CARTESIAN_POINT('Ctrl Pts',(0.496694243903159,4.05643766298363,58.0278223268769));
#7043=CARTESIAN_POINT('Ctrl Pts',(0.378181514051322,4.06745666755404,58.0336493874272));
#7044=CARTESIAN_POINT('Ctrl Pts',(0.352271913713808,4.06986567462774,58.0349233164827));
#7045=CARTESIAN_POINT('Ctrl Pts',(0.326347934062307,4.07202630341459,58.0361972455381));
#7046=CARTESIAN_POINT('Ctrl Pts',(0.300414697640057,4.07393863594456,58.0374711745936));
#7047=CARTESIAN_POINT('Ctrl Pts',(0.181800445423052,4.08268532260331,58.0432979113661));
#7048=CARTESIAN_POINT('Ctrl Pts',(0.0626151280544477,4.08626138513636,58.0491246481386));
#7049=CARTESIAN_POINT('Ctrl Pts',(-0.0566535826103796,4.08460712573161,
58.0549513849111));
#7050=CARTESIAN_POINT('Ctrl Pts',(-0.175773077047609,4.08295493595891,58.0607708318951));
#7051=CARTESIAN_POINT('Ctrl Pts',(-0.294975353010617,4.07608544540713,58.0665902788791));
#7052=CARTESIAN_POINT('Ctrl Pts',(-0.413768179883462,4.06399075950179,58.072409725863));
#7053=CARTESIAN_POINT('Ctrl Pts',(-0.53244324554876,4.05190806324982,58.0782234039372));
#7054=CARTESIAN_POINT('Ctrl Pts',(-0.650709266199974,4.03461051768562,58.0840370820113));
#7055=CARTESIAN_POINT('Ctrl Pts',(-0.768075172731697,4.0121422618139,58.0898507600855));
#7056=CARTESIAN_POINT('Ctrl Pts',(-0.889095948495576,3.98897432628638,58.0958454807959));
#7057=CARTESIAN_POINT('Ctrl Pts',(-1.00915919048552,3.96030837484129,58.1018402015062));
#7058=CARTESIAN_POINT('Ctrl Pts',(-1.12773304273466,3.92625052490597,58.1078349222166));
#7059=CARTESIAN_POINT('Ctrl Pts',(-1.24259866302598,3.89325778675668,58.1136421663923));
#7060=CARTESIAN_POINT('Ctrl Pts',(-1.35606624184807,3.85520549333451,58.1194494105681));
#7061=CARTESIAN_POINT('Ctrl Pts',(-1.46766442048272,3.81224161732295,58.1252566547438));
#7062=CARTESIAN_POINT('Ctrl Pts',(-1.57924661033535,3.76928389678863,58.1310630669099));
#7063=CARTESIAN_POINT('Ctrl Pts',(-1.68895955219553,3.7214161396405,58.136869479076));
#7064=CARTESIAN_POINT('Ctrl Pts',(-1.79634995928534,3.66883521349427,58.1426758912421));
#7065=CARTESIAN_POINT('Ctrl Pts',(-1.90375024145776,3.61624945227009,58.1484828373367));
#7066=CARTESIAN_POINT('Ctrl Pts',(-2.0088271979684,3.55894983967916,58.1542897834313));
#7067=CARTESIAN_POINT('Ctrl Pts',(-2.11115090204654,3.49717984507347,58.1600967295259));
#7068=CARTESIAN_POINT('Ctrl Pts',(-2.21350808428251,3.43538964062836,58.1659055755308));
#7069=CARTESIAN_POINT('Ctrl Pts',(-2.31310987362147,3.36912635593796,58.1717144215357));
#7070=CARTESIAN_POINT('Ctrl Pts',(-2.4095546966394,3.29867718394859,58.1775232675406));
#7071=CARTESIAN_POINT('Ctrl Pts',(-2.50610546819611,3.22815062069449,58.1833384947977));
#7072=CARTESIAN_POINT('Ctrl Pts',(-2.59949202165173,3.15342923237338,58.1891537220549));
#7073=CARTESIAN_POINT('Ctrl Pts',(-2.6893451871139,3.07484104703761,58.1949689493121));
#7074=CARTESIAN_POINT('Ctrl Pts',(-2.77925751311814,2.99620111817537,58.2007880053937));
#7075=CARTESIAN_POINT('Ctrl Pts',(-2.86563152368462,2.91368960285899,58.2066070614753));
#7076=CARTESIAN_POINT('Ctrl Pts',(-2.94813546623174,2.82767082114354,58.2124261175569));
#7077=CARTESIAN_POINT('Ctrl Pts',(-3.03075547280752,2.74153103083094,58.218253359709));
#7078=CARTESIAN_POINT('Ctrl Pts',(-3.10949427745213,2.6518744321804,58.2240806018611));
#7079=CARTESIAN_POINT('Ctrl Pts',(-3.18406081488101,2.55909783461659,58.2299078440133));
#7080=CARTESIAN_POINT('Ctrl Pts',(-3.20033848626719,2.53884495685741,58.2311799150536));
#7081=CARTESIAN_POINT('Ctrl Pts',(-3.21641750014398,2.51844350545445,58.2324519860939));
#7082=CARTESIAN_POINT('Ctrl Pts',(-3.23229511105798,2.49789777913963,58.2337240571342));
#7083=CARTESIAN_POINT('Ctrl Pts',(-3.30497237932344,2.40385294637613,58.2395467623731));
#7084=CARTESIAN_POINT('Ctrl Pts',(-3.37366200923957,2.30647812772046,58.245369467612));
#7085=CARTESIAN_POINT('Ctrl Pts',(-3.43804411656929,2.20614542868852,58.2511921728509));
#7086=CARTESIAN_POINT('Ctrl Pts',(-3.50234761952142,2.10593522625831,58.2570077691252));
#7087=CARTESIAN_POINT('Ctrl Pts',(-3.56235383823522,2.00277466344739,58.2628233653995));
#7088=CARTESIAN_POINT('Ctrl Pts',(-3.61778331695694,1.89706849416356,58.2686389616738));
#7089=CARTESIAN_POINT('Ctrl Pts',(-3.67315817556485,1.7914664875587,58.2744488272695));
#7090=CARTESIAN_POINT('Ctrl Pts',(-3.72396507498049,1.68332422195153,58.2802586928651));
#7091=CARTESIAN_POINT('Ctrl Pts',(-3.76996840064677,1.57307446045153,58.2860685584607));
#7092=CARTESIAN_POINT('Ctrl Pts',(-3.8159372266017,1.46290737960325,58.2918740670086));
#7093=CARTESIAN_POINT('Ctrl Pts',(-3.85710948865528,1.35063632196236,58.2976795755566));
#7094=CARTESIAN_POINT('Ctrl Pts',(-3.89329627824057,1.23671706135161,58.3034850841045));
#7095=CARTESIAN_POINT('Ctrl Pts',(-3.92946682042483,1.12284894901713,58.309287986054));
#7096=CARTESIAN_POINT('Ctrl Pts',(-3.96065621842049,1.00733449342105,58.3150908880036));
#7097=CARTESIAN_POINT('Ctrl Pts',(-3.98672452292116,0.890647280543241,58.3208937899532));
#7098=CARTESIAN_POINT('Ctrl Pts',(-4.01278586190416,0.773991246787297,58.3266951413525));
#7099=CARTESIAN_POINT('Ctrl Pts',(-4.03372874412109,0.656163477712639,58.3324964927518));
#7100=CARTESIAN_POINT('Ctrl Pts',(-4.04946387960724,0.537649781694597,58.3382978441512));
#7101=CARTESIAN_POINT('Ctrl Pts',(-4.06520193070151,0.419114125935964,58.3441002704994));
#7102=CARTESIAN_POINT('Ctrl Pts',(-4.07573025238781,0.299892693576237,58.3499026968477));
#7103=CARTESIAN_POINT('Ctrl Pts',(-4.08101122655926,0.180478166815966,58.3557051231959));
#7104=CARTESIAN_POINT('Ctrl Pts',(-4.08371429004001,0.119355912497564,58.3586750916625));
#7105=CARTESIAN_POINT('Ctrl Pts',(-4.08504344081981,0.0581831381100053,
58.361645060129));
#7106=CARTESIAN_POINT('Ctrl Pts',(-4.08499891745933,-0.00297394621324721,
58.3646150285955));
#7107=CARTESIAN_POINT('Ctrl Pts',(-4.08499891745875,-0.00297394700961363,
58.3646150286342));
#7108=CARTESIAN_POINT('Ctrl Pts',(-4.08489785974511,-0.14178632311568,58.3713561672016));
#7109=CARTESIAN_POINT('Ctrl Pts',(-4.07771738177627,-0.28031599001206,58.378097305769));
#7110=CARTESIAN_POINT('Ctrl Pts',(-4.06356739568884,-0.417905516468299,
58.3848384443363));
#7111=CARTESIAN_POINT('Ctrl Pts',(-4.0493356015318,-0.556290516042897,58.3916185567607));
#7112=CARTESIAN_POINT('Ctrl Pts',(-4.02805358644635,-0.693724362004736,
58.398398669185));
#7113=CARTESIAN_POINT('Ctrl Pts',(-3.99988246908372,-0.829557251500295,
58.4051787816093));
#7114=CARTESIAN_POINT('Ctrl Pts',(-3.97153196598098,-0.966255086574672,
58.4120020678797));
#7115=CARTESIAN_POINT('Ctrl Pts',(-3.93620442598652,-1.10133140441473,58.4188253541501));
#7116=CARTESIAN_POINT('Ctrl Pts',(-3.8941124171469,-1.23414483859161,58.4256486404205));
#7117=CARTESIAN_POINT('Ctrl Pts',(-3.88521216960954,-1.26222789932092,58.4270914068386));
#7118=CARTESIAN_POINT('Ctrl Pts',(-3.87600965127867,-1.29020986379836,58.4285341732567));
#7119=CARTESIAN_POINT('Ctrl Pts',(-3.86650714144293,-1.31808479437811,58.4299769396749));
#7120=CARTESIAN_POINT('Ctrl Pts',(-3.82814300626743,-1.4306232314074,58.4358017677306));
#7121=CARTESIAN_POINT('Ctrl Pts',(-3.78480033911442,-1.54166471466195,58.4416265957864));
#7122=CARTESIAN_POINT('Ctrl Pts',(-3.73661489342043,-1.65073745285815,58.4474514238421));
#7123=CARTESIAN_POINT('Ctrl Pts',(-3.68848594587143,-1.75968230166186,58.4532694222012));
#7124=CARTESIAN_POINT('Ctrl Pts',(-3.63552567337794,-1.86666262561796,58.4590874205602));
#7125=CARTESIAN_POINT('Ctrl Pts',(-3.57791929970426,-1.97122258631636,58.4649054189193));
#7126=CARTESIAN_POINT('Ctrl Pts',(-3.52036690180499,-2.07568457686856,58.470717965955));
#7127=CARTESIAN_POINT('Ctrl Pts',(-3.45817725636424,-2.17773035931255,58.4765305129908));
#7128=CARTESIAN_POINT('Ctrl Pts',(-3.39158304093662,-2.27692544375769,58.4823430600265));
#7129=CARTESIAN_POINT('Ctrl Pts',(-3.32503554001746,-2.37605094483762,58.4881515296769));
#7130=CARTESIAN_POINT('Ctrl Pts',(-3.25408984261685,-2.47232938875589,58.4939599993273));
#7131=CARTESIAN_POINT('Ctrl Pts',(-3.17902346303331,-2.56535276745396,58.4997684689777));
#7132=CARTESIAN_POINT('Ctrl Pts',(-3.10398684139246,-2.65833926966502,58.5055746360247));
#7133=CARTESIAN_POINT('Ctrl Pts',(-3.02483304191969,-2.74807295587033,58.5113808030716));
#7134=CARTESIAN_POINT('Ctrl Pts',(-2.94188130048249,-2.83417702585274,58.5171869701185));
#7135=CARTESIAN_POINT('Ctrl Pts',(-2.85894811056118,-2.92026183932533,58.5229918386611));
#7136=CARTESIAN_POINT('Ctrl Pts',(-2.77221895421885,-3.00271836067829,58.5287967072036));
#7137=CARTESIAN_POINT('Ctrl Pts',(-2.6820510311498,-3.08120548914029,58.5346015757461));
#7138=CARTESIAN_POINT('Ctrl Pts',(-2.59186613596601,-3.15970739106613,58.5404075369266));
#7139=CARTESIAN_POINT('Ctrl Pts',(-2.49824148995269,-3.2342381411996,58.5462134981071));
#7140=CARTESIAN_POINT('Ctrl Pts',(-2.40156828346354,-3.30449614614119,58.5520194592876));
#7141=CARTESIAN_POINT('Ctrl Pts',(-2.37244521715133,-3.32566156116347,58.5537685208798));
#7142=CARTESIAN_POINT('Ctrl Pts',(-2.3430456986581,-3.34643949841264,58.555517582472));
#7143=CARTESIAN_POINT('Ctrl Pts',(-2.31338095599002,-3.36682247118299,58.5572666440642));
#7144=CARTESIAN_POINT('',(-4.08499950778543,0.00200534106489888,58.2603849714451));
#7145=CARTESIAN_POINT('Ctrl Pts',(-4.08499950778543,0.00200534106489888,
58.2603849714451));
#7146=CARTESIAN_POINT('Ctrl Pts',(-4.08505725975092,-0.115638861568439,
58.2661416094535));
#7147=CARTESIAN_POINT('Ctrl Pts',(-4.0800287331631,-0.233480689917119,58.271898247462));
#7148=CARTESIAN_POINT('Ctrl Pts',(-4.06988904518043,-0.351038687213156,
58.2776548854704));
#7149=CARTESIAN_POINT('Ctrl Pts',(-4.05976110079072,-0.468460531082006,
58.2834048562506));
#7150=CARTESIAN_POINT('Ctrl Pts',(-4.04453380004621,-0.585598784051002,
58.2891548270309));
#7151=CARTESIAN_POINT('Ctrl Pts',(-4.0242342774865,-0.70197113893855,58.2949047978111));
#7152=CARTESIAN_POINT('Ctrl Pts',(-4.00305659713254,-0.823377764468657,
58.3009035124543));
#7153=CARTESIAN_POINT('Ctrl Pts',(-3.97635795742803,-0.943950276068998,
58.3069022270975));
#7154=CARTESIAN_POINT('Ctrl Pts',(-3.94422954554652,-1.06314547077899,58.3129009417407));
#7155=CARTESIAN_POINT('Ctrl Pts',(-3.91347786077154,-1.17723305991762,58.3186426068577));
#7156=CARTESIAN_POINT('Ctrl Pts',(-3.87775224096607,-1.2900584790373,58.3243842719746));
#7157=CARTESIAN_POINT('Ctrl Pts',(-3.83718484198393,-1.40115576880259,58.3301259370915));
#7158=CARTESIAN_POINT('Ctrl Pts',(-3.79662751282597,-1.51222548149362,58.3358661769862));
#7159=CARTESIAN_POINT('Ctrl Pts',(-3.75123093677261,-1.6215675247441,58.341606416881));
#7160=CARTESIAN_POINT('Ctrl Pts',(-3.70117666229399,-1.72873257460207,58.3473466567757));
#7161=CARTESIAN_POINT('Ctrl Pts',(-3.65112234603474,-1.83589771391142,58.3530869014618));
#7162=CARTESIAN_POINT('Ctrl Pts',(-3.59641050129044,-1.94088547743368,58.3588271461479));
#7163=CARTESIAN_POINT('Ctrl Pts',(-3.53726987536132,-2.04326866291765,58.3645673908341));
#7164=CARTESIAN_POINT('Ctrl Pts',(-3.47811446962349,-2.14567743494004,58.3703090700623));
#7165=CARTESIAN_POINT('Ctrl Pts',(-3.41452829257581,-2.24547997336317,58.3760507492905));
#7166=CARTESIAN_POINT('Ctrl Pts',(-3.346784472902,-2.34227639102265,58.3817924285188));
#7167=CARTESIAN_POINT('Ctrl Pts',(-3.27897005430982,-2.43917368463542,58.3875400914123));
#7168=CARTESIAN_POINT('Ctrl Pts',(-3.20698958588826,-2.53305826224156,58.3932877543059));
#7169=CARTESIAN_POINT('Ctrl Pts',(-3.13115769800021,-2.62356179082064,58.3990354171994));
#7170=CARTESIAN_POINT('Ctrl Pts',(-3.05527922424442,-2.7141209185089,58.4047866110596));
#7171=CARTESIAN_POINT('Ctrl Pts',(-2.97554490342206,-2.80129455509581,58.4105378049197));
#7172=CARTESIAN_POINT('Ctrl Pts',(-2.89230634090281,-2.88475112104552,58.4162889987798));
#7173=CARTESIAN_POINT('Ctrl Pts',(-2.80894935200499,-2.96832642353483,58.4220483750622));
#7174=CARTESIAN_POINT('Ctrl Pts',(-2.72207847987514,-3.0481738209203,58.4278077513445));
#7175=CARTESIAN_POINT('Ctrl Pts',(-2.6320784946416,-3.12400188829091,58.4335671276269));
#7176=CARTESIAN_POINT('Ctrl Pts',(-2.60443580996555,-3.14729179606681,58.4353360681671));
#7177=CARTESIAN_POINT('Ctrl Pts',(-2.57649814378481,-3.17020284775017,58.4371050087074));
#7178=CARTESIAN_POINT('Ctrl Pts',(-2.54827716476554,-3.19272743771442,58.4388739492477));
#7179=CARTESIAN_POINT('Ctrl Pts',(-2.47218313370533,-3.25346193056061,58.4436436567877));
#7180=CARTESIAN_POINT('Ctrl Pts',(-2.3938175737227,-3.31155358153415,58.4484133643277));
#7181=CARTESIAN_POINT('Ctrl Pts',(-2.31338095599002,-3.36682247118298,58.4531830718678));
#7182=CARTESIAN_POINT('Ctrl Pts',(-2.31338095599003,-3.36682247118298,57.2030181077425));
#7183=CARTESIAN_POINT('Ctrl Pts',(-2.21482775942375,-3.43453946251228,57.2088328619545));
#7184=CARTESIAN_POINT('Ctrl Pts',(-2.11336204419633,-3.4978821844165,57.2146476161665));
#7185=CARTESIAN_POINT('Ctrl Pts',(-2.00941524034814,-3.5566100983741,57.2204623703784));
#7186=CARTESIAN_POINT('Ctrl Pts',(-1.90540266148345,-3.61537517393135,57.2262808040259));
#7187=CARTESIAN_POINT('Ctrl Pts',(-1.79890622990321,-3.66951944100108,57.2320992376733));
#7188=CARTESIAN_POINT('Ctrl Pts',(-1.69037935165581,-3.71884964034521,57.2379176713207));
#7189=CARTESIAN_POINT('Ctrl Pts',(-1.58169626272958,-3.76825084425568,57.2437444798655));
#7190=CARTESIAN_POINT('Ctrl Pts',(-1.47097727010335,-3.81282399589916,57.2495712884103));
#7191=CARTESIAN_POINT('Ctrl Pts',(-1.35869317216081,-3.85242493293816,57.2553980969551));
#7192=CARTESIAN_POINT('Ctrl Pts',(-1.32041886367163,-3.86592371423012,57.257384282638));
#7193=CARTESIAN_POINT('Ctrl Pts',(-1.28196280673188,-3.87884519555452,57.2593704683209));
#7194=CARTESIAN_POINT('Ctrl Pts',(-1.24334393029046,-3.89118502143111,57.2613566540038));
#7195=CARTESIAN_POINT('Ctrl Pts',(-1.1300522447437,-3.92738492680728,57.2671832948738));
#7196=CARTESIAN_POINT('Ctrl Pts',(-1.0149980085889,-3.95869061724581,57.2730099357437));
#7197=CARTESIAN_POINT('Ctrl Pts',(-0.898641461870173,-3.98493017793384,
57.2788365766136));
#7198=CARTESIAN_POINT('Ctrl Pts',(-0.782430478763564,-4.01113691257692,
57.2846559282771));
#7199=CARTESIAN_POINT('Ctrl Pts',(-0.664920820055686,-4.03229003468466,
57.2904752799406));
#7200=CARTESIAN_POINT('Ctrl Pts',(-0.546589254619076,-4.0482669362006,57.2962946316041));
#7201=CARTESIAN_POINT('Ctrl Pts',(-0.428374981075478,-4.0642280011896,57.3021082150453));
#7202=CARTESIAN_POINT('Ctrl Pts',(-0.309340823453885,-4.07502299865065,
57.3079217984865));
#7203=CARTESIAN_POINT('Ctrl Pts',(-0.189974570917122,-4.08058018698381,
57.3137353819277));
#7204=CARTESIAN_POINT('Ctrl Pts',(-0.0668884195559605,-4.08631055808772,
57.3197301383701));
#7205=CARTESIAN_POINT('Ctrl Pts',(0.0565504337260151,-4.08647121584311,
57.3257248948125));
#7206=CARTESIAN_POINT('Ctrl Pts',(0.179800033968628,-4.08104115977588,57.3317196512548));
#7207=CARTESIAN_POINT('Ctrl Pts',(0.299192564565407,-4.07578103614163,57.3375268030878));
#7208=CARTESIAN_POINT('Ctrl Pts',(0.418407073487605,-4.06527491997163,57.3433339549208));
#7209=CARTESIAN_POINT('Ctrl Pts',(0.53695069273696,-4.04955663666645,57.3491411067538));
#7210=CARTESIAN_POINT('Ctrl Pts',(0.655477348374434,-4.03384060265026,57.3549474275824));
#7211=CARTESIAN_POINT('Ctrl Pts',(0.773332901105097,-4.01291393846466,57.360753748411));
#7212=CARTESIAN_POINT('Ctrl Pts',(0.890030639190593,-3.98686223254604,57.3665600692396));
#7213=CARTESIAN_POINT('Ctrl Pts',(1.00673913052452,-3.96080812606276,57.3723669250983));
#7214=CARTESIAN_POINT('Ctrl Pts',(1.12228919706243,-3.92962812775035,57.3781737809571));
#7215=CARTESIAN_POINT('Ctrl Pts',(1.2362059608438,-3.89345859389493,57.3839806368159));
#7216=CARTESIAN_POINT('Ctrl Pts',(1.35016001988649,-3.8572772184793,57.3897893937838));
#7217=CARTESIAN_POINT('Ctrl Pts',(1.4624793242187,-3.81610318208682,57.3955981507518));
#7218=CARTESIAN_POINT('Ctrl Pts',(1.57270635715591,-3.77012197603226,57.4014069077197));
#7219=CARTESIAN_POINT('Ctrl Pts',(1.68305452258816,-3.72409023955819,57.4072220481419));
#7220=CARTESIAN_POINT('Ctrl Pts',(1.79130545065884,-3.67324094598739,57.4130371885642));
#7221=CARTESIAN_POINT('Ctrl Pts',(1.89702359857503,-3.61780685864371,57.4188523289864));
#7222=CARTESIAN_POINT('Ctrl Pts',(2.00281137541744,-3.56233626086114,57.4246712994226));
#7223=CARTESIAN_POINT('Ctrl Pts',(2.10606269816485,-3.50227505996777,57.4304902698588));
#7224=CARTESIAN_POINT('Ctrl Pts',(2.20636993423211,-3.43790004411364,57.436309240295));
#7225=CARTESIAN_POINT('Ctrl Pts',(2.30681832211101,-3.37343444007796,57.4421363991556));
#7226=CARTESIAN_POINT('Ctrl Pts',(2.40431402286169,-3.30464313994416,57.4479635580161));
#7227=CARTESIAN_POINT('Ctrl Pts',(2.49848138145923,-3.23184402261334,57.4537907168767));
#7228=CARTESIAN_POINT('Ctrl Pts',(2.51905219304851,-3.21594109246024,57.455063656766));
#7229=CARTESIAN_POINT('Ctrl Pts',(2.53946431287178,-3.19984705051002,57.4563365966552));
#7230=CARTESIAN_POINT('Ctrl Pts',(2.55971406016711,-3.1835654430501,57.4576095365444));
#7231=CARTESIAN_POINT('Ctrl Pts',(2.65240351183048,-3.10903941338426,57.4634361821125));
#7232=CARTESIAN_POINT('Ctrl Pts',(2.74198304034683,-3.03034344430009,57.4692628276806));
#7233=CARTESIAN_POINT('Ctrl Pts',(2.82805536971624,-2.94776658265527,57.4750894732486));
#7234=CARTESIAN_POINT('Ctrl Pts',(2.91402002204039,-2.8652930252028,57.4809088296451));
#7235=CARTESIAN_POINT('Ctrl Pts',(2.99648591045966,-2.77894851193904,57.4867281860416));
#7236=CARTESIAN_POINT('Ctrl Pts',(3.07508776726771,-2.68906307542246,57.4925475424381));
#7237=CARTESIAN_POINT('Ctrl Pts',(3.15361171327372,-2.59926673408423,57.498361130641));
#7238=CARTESIAN_POINT('Ctrl Pts',(3.22827898041083,-2.50593675729864,57.5041747188439));
#7239=CARTESIAN_POINT('Ctrl Pts',(3.29876064887406,-2.40944042911212,57.5099883070468));
#7240=CARTESIAN_POINT('Ctrl Pts',(3.37143870867106,-2.30993702541801,57.5159830617151));
#7241=CARTESIAN_POINT('Ctrl Pts',(3.43966570994165,-2.20706700003783,57.5219778163833));
#7242=CARTESIAN_POINT('Ctrl Pts',(3.50312517674191,-2.10127080503133,57.5279725710516));
#7243=CARTESIAN_POINT('Ctrl Pts',(3.56459876224643,-1.99878536404491,57.5337797276865));
#7244=CARTESIAN_POINT('Ctrl Pts',(3.62159852602436,-1.89355453901573,57.5395868843215));
#7245=CARTESIAN_POINT('Ctrl Pts',(3.67388079862009,-1.78600808439676,57.5453940409564));
#7246=CARTESIAN_POINT('Ctrl Pts',(3.72615558967732,-1.67847701956292,57.5512003665933));
#7247=CARTESIAN_POINT('Ctrl Pts',(3.77371405387893,-1.56863135083147,57.5570066922302));
#7248=CARTESIAN_POINT('Ctrl Pts',(3.81635909262693,-1.45692425201992,57.5628130178671));
#7249=CARTESIAN_POINT('Ctrl Pts',(3.8590080609555,-1.34520685981764,57.5686198785351));
#7250=CARTESIAN_POINT('Ctrl Pts',(3.89674255819498,-1.23162807751074,57.5744267392031));
#7251=CARTESIAN_POINT('Ctrl Pts',(3.9294143584382,-1.11665921377103,57.5802335998712));
#7252=CARTESIAN_POINT('Ctrl Pts',(3.96209685508355,-1.00165271044029,57.5860423616441));
#7253=CARTESIAN_POINT('Ctrl Pts',(3.9897132469091,-0.885255612638544,57.5918511234169));
#7254=CARTESIAN_POINT('Ctrl Pts',(4.01216586793536,-0.767951852771041,57.5976598851898));
#7255=CARTESIAN_POINT('Ctrl Pts',(4.03464316282455,-0.650519184261271,57.6034750303863));
#7256=CARTESIAN_POINT('Ctrl Pts',(4.05194528354712,-0.532178265681518,57.6092901755828));
#7257=CARTESIAN_POINT('Ctrl Pts',(4.06402611460516,-0.41342077815135,57.6151053207793));
#7258=CARTESIAN_POINT('Ctrl Pts',(4.0761149024035,-0.294585073942095,57.6209242959772));
#7259=CARTESIAN_POINT('Ctrl Pts',(4.08297552839478,-0.17533266054159,57.6267432711751));
#7260=CARTESIAN_POINT('Ctrl Pts',(4.08461399380378,-0.0561562251430488,
57.632562246373));
#7261=CARTESIAN_POINT('Ctrl Pts',(4.08625476483559,0.0631879134646265,57.6383894099415));
#7262=CARTESIAN_POINT('Ctrl Pts',(4.08265872117685,0.18245545458868,57.64421657351));
#7263=CARTESIAN_POINT('Ctrl Pts',(4.07388377719373,0.301157716018913,57.6500437370785));
#7264=CARTESIAN_POINT('Ctrl Pts',(4.07196696579233,0.327087208961452,57.6513166310807));
#7265=CARTESIAN_POINT('Ctrl Pts',(4.06980322869673,0.352989764867805,57.6525895250829));
#7266=CARTESIAN_POINT('Ctrl Pts',(4.06739349327876,0.378860357959995,57.6538624190851));
#7267=CARTESIAN_POINT('Ctrl Pts',(4.05636301354315,0.497282094522663,57.6596890469349));
#7268=CARTESIAN_POINT('Ctrl Pts',(4.040138935536,0.615410174995458,57.6655156747847));
#7269=CARTESIAN_POINT('Ctrl Pts',(4.01874319674208,0.732753791282729,57.6713423026346));
#7270=CARTESIAN_POINT('Ctrl Pts',(3.99737422432736,0.849950609006079,57.6771616412885));
#7271=CARTESIAN_POINT('Ctrl Pts',(3.97084653240757,0.966364516798952,57.6829809799425));
#7272=CARTESIAN_POINT('Ctrl Pts',(3.93923390095314,1.08150879496263,57.6888003185965));
#7273=CARTESIAN_POINT('Ctrl Pts',(3.9076526043076,1.19653894077522,57.6946138890541));
#7274=CARTESIAN_POINT('Ctrl Pts',(3.87099650278965,1.31030156956013,57.7004274595118));
#7275=CARTESIAN_POINT('Ctrl Pts',(3.82939049808816,1.42231972957986,57.7062410299694));
#7276=CARTESIAN_POINT('Ctrl Pts',(3.7864877639697,1.53782914631539,57.7122357912884));
#7277=CARTESIAN_POINT('Ctrl Pts',(3.73832160506255,1.65148313922527,57.7182305526075));
#7278=CARTESIAN_POINT('Ctrl Pts',(3.68508481835105,1.76277476767698,57.7242253139265));
#7279=CARTESIAN_POINT('Ctrl Pts',(3.63351422134615,1.87058322260879,57.7300324529223));
#7280=CARTESIAN_POINT('Ctrl Pts',(3.57718584971938,1.97617458602078,57.7358395919181));
#7281=CARTESIAN_POINT('Ctrl Pts',(3.51632373812308,2.0791085514499,57.7416467309139));
#7282=CARTESIAN_POINT('Ctrl Pts',(3.45547033512344,2.18202778833342,57.7474530389817));
#7283=CARTESIAN_POINT('Ctrl Pts',(3.39008468984156,2.2822900325073,57.7532593470495));
#7284=CARTESIAN_POINT('Ctrl Pts',(3.3204360607725,2.3794809027016,57.7590656551173));
#7285=CARTESIAN_POINT('Ctrl Pts',(3.2507810127535,2.47668073019108,57.7648724983056));
#7286=CARTESIAN_POINT('Ctrl Pts',(3.176862437355,2.57080828940431,57.7706793414938));
#7287=CARTESIAN_POINT('Ctrl Pts',(3.09899167892451,2.66147995933779,57.776486184682));
#7288=CARTESIAN_POINT('Ctrl Pts',(3.02109542489957,2.75218131600055,57.7822949290834));
#7289=CARTESIAN_POINT('Ctrl Pts',(2.93924467991378,2.83942422385016,57.7881036734849));
#7290=CARTESIAN_POINT('Ctrl Pts',(2.85378920812506,2.92286026959705,57.7939124178864));
#7291=CARTESIAN_POINT('Ctrl Pts',(2.76823982283651,3.00638800954332,57.7997275459577));
#7292=CARTESIAN_POINT('Ctrl Pts',(2.67907809544267,3.08610025169248,57.8055426740289));
#7293=CARTESIAN_POINT('Ctrl Pts',(2.5866886901372,3.16168730590429,57.8113578021002));
#7294=CARTESIAN_POINT('Ctrl Pts',(2.49423843267743,3.23732414542503,57.8171767602976));
#7295=CARTESIAN_POINT('Ctrl Pts',(2.39855658930083,3.30883014224941,57.822995718495));
#7296=CARTESIAN_POINT('Ctrl Pts',(2.3000574125857,3.37593852118334,57.8288146766923));
#7297=CARTESIAN_POINT('Ctrl Pts',(2.20141962377296,3.44314133779159,57.8346418235673));
#7298=CARTESIAN_POINT('Ctrl Pts',(2.09995693434531,3.50593397156601,57.8404689704423));
#7299=CARTESIAN_POINT('Ctrl Pts',(1.99610889330301,3.56409515670901,57.8462961173172));
#7300=CARTESIAN_POINT('Ctrl Pts',(1.97342112875701,3.57680167732314,57.8475691787534));
#7301=CARTESIAN_POINT('Ctrl Pts',(1.95061958949687,3.58928732321926,57.8488422401896));
#7302=CARTESIAN_POINT('Ctrl Pts',(1.92770898090545,3.60155009474205,57.8501153016258));
#7303=CARTESIAN_POINT('Ctrl Pts',(1.82284989761685,3.65767531617936,57.8559419497759));
#7304=CARTESIAN_POINT('Ctrl Pts',(1.71537077353199,3.70930660615456,57.8617685979261));
#7305=CARTESIAN_POINT('Ctrl Pts',(1.60569308936343,3.75619151572048,57.8675952460762));
#7306=CARTESIAN_POINT('Ctrl Pts',(1.49615261469705,3.8030177711021,57.8734146049451));
#7307=CARTESIAN_POINT('Ctrl Pts',(1.38441942247576,3.84510929777986,57.879233963814));
#7308=CARTESIAN_POINT('Ctrl Pts',(1.2709401812882,3.88225914328077,57.8850533226828));
#7309=CARTESIAN_POINT('Ctrl Pts',(1.1575734237696,3.91937216485794,57.890866913247));
#7310=CARTESIAN_POINT('Ctrl Pts',(1.04246444587559,3.95155312403871,57.8966805038112));
#7311=CARTESIAN_POINT('Ctrl Pts',(0.926079969253856,3.97864309665328,57.9024940943754));
#7312=CARTESIAN_POINT('Ctrl Pts',(0.806068718211667,4.00657724731101,57.9084888481167));
#7313=CARTESIAN_POINT('Ctrl Pts',(0.684701578090561,4.02909774990616,57.914483601858));
#7314=CARTESIAN_POINT('Ctrl Pts',(0.562507729921121,4.0460857694541,57.9204783555993));
#7315=CARTESIAN_POINT('Ctrl Pts',(0.444137718385236,4.06254217949426,57.9262855143077));
#7316=CARTESIAN_POINT('Ctrl Pts',(0.324992401423549,4.07380714096769,57.9320926730161));
#7317=CARTESIAN_POINT('Ctrl Pts',(0.205562620331488,4.07982462970192,57.9378998317245));
#7318=CARTESIAN_POINT('Ctrl Pts',(0.0861499317634045,4.08584125722659,57.9437061593253));
#7319=CARTESIAN_POINT('Ctrl Pts',(-0.0335467327789725,4.08661188510273,
57.9495124869261));
#7320=CARTESIAN_POINT('Ctrl Pts',(-0.153033208793098,4.08213251095631,57.9553188145269));
#7321=CARTESIAN_POINT('Ctrl Pts',(-0.272530692746211,4.07765272413828,57.9611256770477));
#7322=CARTESIAN_POINT('Ctrl Pts',(-0.391817542131322,4.06792198892883,57.9669325395684));
#7323=CARTESIAN_POINT('Ctrl Pts',(-0.51040203308808,4.05298837459714,57.9727394020892));
#7324=CARTESIAN_POINT('Ctrl Pts',(-0.629025345035767,4.03804987144987,57.9785481656018));
#7325=CARTESIAN_POINT('Ctrl Pts',(-0.746945436868593,4.01790515262829,57.9843569291145));
#7326=CARTESIAN_POINT('Ctrl Pts',(-0.863678757197371,3.99265375463062,57.9901656926271));
#7327=CARTESIAN_POINT('Ctrl Pts',(-0.980540355762733,3.96737460787366,57.9959808393896));
#7328=CARTESIAN_POINT('Ctrl Pts',(-1.09621218093062,3.93697766708333,58.001795986152));
#7329=CARTESIAN_POINT('Ctrl Pts',(-1.21022372759133,3.90161293943607,58.0076111329144));
#7330=CARTESIAN_POINT('Ctrl Pts',(-1.32431036315668,3.86622492030001,58.0134301095784));
#7331=CARTESIAN_POINT('Ctrl Pts',(-1.43673415956687,3.82586273569657,58.0192490862424));
#7332=CARTESIAN_POINT('Ctrl Pts',(-1.54704408431669,3.78072474549269,58.0250680629064));
#7333=CARTESIAN_POINT('Ctrl Pts',(-1.65750923249171,3.73552323903257,58.0308952277864));
#7334=CARTESIAN_POINT('Ctrl Pts',(-1.76585420343812,3.68553268467108,58.0367223926664));
#7335=CARTESIAN_POINT('Ctrl Pts',(-1.87165196886338,3.63099764630189,58.0425495575463));
#7336=CARTESIAN_POINT('Ctrl Pts',(-1.89476224471286,3.6190851094434,58.0438224330863));
#7337=CARTESIAN_POINT('Ctrl Pts',(-1.91775108931573,3.60695589583663,58.0450953086263));
#7338=CARTESIAN_POINT('Ctrl Pts',(-1.9406142410025,3.59461282582955,58.0463681841663));
#7339=CARTESIAN_POINT('Ctrl Pts',(-2.04527186694745,3.53811158656426,58.0521948581947));
#7340=CARTESIAN_POINT('Ctrl Pts',(-2.14762643153128,3.47694596369644,58.0580215322231));
#7341=CARTESIAN_POINT('Ctrl Pts',(-2.24723486545104,3.41132825443423,58.0638482062514));
#7342=CARTESIAN_POINT('Ctrl Pts',(-2.34671869217198,3.34579263098163,58.0696675912833));
#7343=CARTESIAN_POINT('Ctrl Pts',(-2.44346288362712,3.27581622138491,58.0754869763151));
#7344=CARTESIAN_POINT('Ctrl Pts',(-2.53704842444072,3.20165742890192,58.081306361347));
#7345=CARTESIAN_POINT('Ctrl Pts',(-2.63054120518579,3.12757214109297,58.0871199783237));
#7346=CARTESIAN_POINT('Ctrl Pts',(-2.72088124599173,3.0493129694803,58.0929335953005));
#7347=CARTESIAN_POINT('Ctrl Pts',(-2.80767852963759,2.96718153711769,58.0987472122773));
#7348=CARTESIAN_POINT('Ctrl Pts',(-2.89718003820848,2.88249124741308,58.1047419562118));
#7349=CARTESIAN_POINT('Ctrl Pts',(-2.98291405199093,2.79368370286021,58.1107367001464));
#7350=CARTESIAN_POINT('Ctrl Pts',(-3.06448954424795,2.70113473066321,58.116731444081));
#7351=CARTESIAN_POINT('Ctrl Pts',(-3.14351277298175,2.61148135074906,58.1225386296466));
#7352=CARTESIAN_POINT('Ctrl Pts',(-3.21863352764701,2.51831749814447,58.1283458152122));
#7353=CARTESIAN_POINT('Ctrl Pts',(-3.28953431352081,2.42202167623851,58.1341530007778));
#7354=CARTESIAN_POINT('Ctrl Pts',(-3.36042495370079,2.32573963398128,58.1399593553522));
#7355=CARTESIAN_POINT('Ctrl Pts',(-3.4270965843326,2.22632684206686,58.1457657099267));
#7356=CARTESIAN_POINT('Ctrl Pts',(-3.48927326829827,2.12419327254822,58.1515720645011));
#7357=CARTESIAN_POINT('Ctrl Pts',(-3.55145568131312,2.02205029229544,58.1573789540814));
#7358=CARTESIAN_POINT('Ctrl Pts',(-3.60914211212391,1.91718638434116,58.1631858436618));
#7359=CARTESIAN_POINT('Ctrl Pts',(-3.66210140227677,1.81003820938745,58.1689927332421));
#7360=CARTESIAN_POINT('Ctrl Pts',(-3.71507803013084,1.70285495648919,58.1748015238697));
#7361=CARTESIAN_POINT('Ctrl Pts',(-3.76332425891592,1.59338631471032,58.1806103144973));
#7362=CARTESIAN_POINT('Ctrl Pts',(-3.80665636654012,1.48209051919225,58.186419105125));
#7363=CARTESIAN_POINT('Ctrl Pts',(-3.85003609117596,1.37067242237198,58.1922342789466));
#7364=CARTESIAN_POINT('Ctrl Pts',(-3.88849076799865,1.25742354435471,58.1980494527683));
#7365=CARTESIAN_POINT('Ctrl Pts',(-3.92188596860426,1.14281907984817,58.20386462659));
#7366=CARTESIAN_POINT('Ctrl Pts',(-3.95530316343759,1.02813913633134,58.209683630311));
#7367=CARTESIAN_POINT('Ctrl Pts',(-3.98365414917503,0.912102223470705,58.215502634032));
#7368=CARTESIAN_POINT('Ctrl Pts',(-4.00685556947186,0.795193967150351,58.221321637753));
#7369=CARTESIAN_POINT('Ctrl Pts',(-4.03008963684286,0.678121207430407,58.2271488294834));
#7370=CARTESIAN_POINT('Ctrl Pts',(-4.04815961548415,0.560175058809684,58.2329760212138));
#7371=CARTESIAN_POINT('Ctrl Pts',(-4.0610339287282,0.441846613338161,58.2388032129441));
#7372=CARTESIAN_POINT('Ctrl Pts',(-4.06384558870313,0.416004508386912,58.2400758308651));
#7373=CARTESIAN_POINT('Ctrl Pts',(-4.06640963620481,0.390144169142279,58.241348448786));
#7374=CARTESIAN_POINT('Ctrl Pts',(-4.06872607274419,0.364270702873046,58.242621066707));
#7375=CARTESIAN_POINT('Ctrl Pts',(-4.0795041068123,0.243885319475625,58.2485423682728));
#7376=CARTESIAN_POINT('Ctrl Pts',(-4.0849401038509,0.123014653272814,58.2544636698387));
#7377=CARTESIAN_POINT('Ctrl Pts',(-4.08499950778502,0.0020053418937903,
58.2603849714045));
#7378=CARTESIAN_POINT('Origin',(0.,0.,46.4896150285955));
#7379=CARTESIAN_POINT('',(-2.31338095599003,-3.36682247118298,55.9532017097085));
#7380=CARTESIAN_POINT('',(-2.31338095599004,-3.36682247118297,56.0572684648156));
#7381=CARTESIAN_POINT('',(-2.31338095599002,-3.36682247118298,46.4896150285955));
#7382=CARTESIAN_POINT('',(-4.08499865687907,0.00331259659223695,57.114615028566));
#7383=CARTESIAN_POINT('Ctrl Pts',(-2.31338095599003,-3.36682247118297,56.0572684648156));
#7384=CARTESIAN_POINT('Ctrl Pts',(-2.21397890120566,-3.43512272238204,56.0631597596061));
#7385=CARTESIAN_POINT('Ctrl Pts',(-2.1116806615307,-3.49892710534314,56.0690510543966));
#7386=CARTESIAN_POINT('Ctrl Pts',(-2.00693994771235,-3.55800745449983,56.0749423491871));
#7387=CARTESIAN_POINT('Ctrl Pts',(-1.90334871876782,-3.61643942190295,56.080768989518));
#7388=CARTESIAN_POINT('Ctrl Pts',(-1.79703864418861,-3.670436550343,56.0865956298489));
#7389=CARTESIAN_POINT('Ctrl Pts',(-1.68842551388699,-3.71973712566566,56.0924222701799));
#7390=CARTESIAN_POINT('Ctrl Pts',(-1.57994825985969,-3.76897602540198,56.0982416213167));
#7391=CARTESIAN_POINT('Ctrl Pts',(-1.46917404899166,-3.81352989142549,56.1040609724536));
#7392=CARTESIAN_POINT('Ctrl Pts',(-1.35654485975385,-3.85318193749989,56.1098803235905));
#7393=CARTESIAN_POINT('Ctrl Pts',(-1.24402730989515,-3.89279467999913,56.115693906518));
#7394=CARTESIAN_POINT('Ctrl Pts',(-1.12965882212408,-3.92751513407801,56.1215074894455));
#7395=CARTESIAN_POINT('Ctrl Pts',(-1.0139024859278,-3.9571740862678,56.127321072373));
#7396=CARTESIAN_POINT('Ctrl Pts',(-0.894538734921794,-3.98775732603343,
56.1333158290128));
#7397=CARTESIAN_POINT('Ctrl Pts',(-0.773699619115147,-4.01295824181281,
56.1393105856525));
#7398=CARTESIAN_POINT('Ctrl Pts',(-0.651911561980285,-4.03264631667053,
56.1453053422923));
#7399=CARTESIAN_POINT('Ctrl Pts',(-0.533934849427476,-4.05171825527315,
56.1511124936465));
#7400=CARTESIAN_POINT('Ctrl Pts',(-0.415068135911994,-4.06561718497902,
56.1569196450007));
#7401=CARTESIAN_POINT('Ctrl Pts',(-0.29580090182949,-4.07427623345262,56.1627267963549));
#7402=CARTESIAN_POINT('Ctrl Pts',(-0.176550734628493,-4.08293404283524,
56.1685331167184));
#7403=CARTESIAN_POINT('Ctrl Pts',(-0.0569005674815752,-4.08635343270106,
56.1743394370819));
#7404=CARTESIAN_POINT('Ctrl Pts',(0.0626556456337905,-4.08451946623715,
56.1801457574454));
#7405=CARTESIAN_POINT('Ctrl Pts',(0.182222875687124,-4.08268533077579,56.1859526128532));
#7406=CARTESIAN_POINT('Ctrl Pts',(0.301695726716485,-4.07559688275356,56.191759468261));
#7407=CARTESIAN_POINT('Ctrl Pts',(0.420581532512456,-4.06329129825927,56.1975663236687));
#7408=CARTESIAN_POINT('Ctrl Pts',(0.539506260688669,-4.05098168500279,56.2033750802003));
#7409=CARTESIAN_POINT('Ctrl Pts',(0.657843155966779,-4.03345158023778,56.2091838367319));
#7410=CARTESIAN_POINT('Ctrl Pts',(0.775106583720403,-4.01078979552323,56.2149925932635));
#7411=CARTESIAN_POINT('Ctrl Pts',(0.892498877004137,-3.98810310685562,56.2208077332729));
#7412=CARTESIAN_POINT('Ctrl Pts',(1.00881494749444,-3.96027355928179,56.2266228732823));
#7413=CARTESIAN_POINT('Ctrl Pts',(1.12358108680821,-3.92744071137514,56.2324380132917));
#7414=CARTESIAN_POINT('Ctrl Pts',(1.23842281457585,-3.89458623876086,56.2382569833284));
#7415=CARTESIAN_POINT('Ctrl Pts',(1.35171219223955,-3.85672203189154,56.244075953365));
#7416=CARTESIAN_POINT('Ctrl Pts',(1.46299390931844,-3.81403642107638,56.2498949234017));
#7417=CARTESIAN_POINT('Ctrl Pts',(1.57443222187445,-3.7712907431292,56.2557220818849));
#7418=CARTESIAN_POINT('Ctrl Pts',(1.68385686272124,-3.72371028227369,56.2615492403681));
#7419=CARTESIAN_POINT('Ctrl Pts',(1.79083549731539,-3.67153009269366,56.2673763988513));
#7420=CARTESIAN_POINT('Ctrl Pts',(1.81420500797559,-3.66013131665518,56.2686493431434));
#7421=CARTESIAN_POINT('Ctrl Pts',(1.83745789961868,-3.64851320605675,56.2699222874356));
#7422=CARTESIAN_POINT('Ctrl Pts',(1.86058984850693,-3.63667848670087,56.2711952317278));
#7423=CARTESIAN_POINT('Ctrl Pts',(1.9664715829446,-3.58250749496832,56.2770218721959));
#7424=CARTESIAN_POINT('Ctrl Pts',(2.07015408541998,-3.52362234382874,56.282848512664));
#7425=CARTESIAN_POINT('Ctrl Pts',(2.17118969993181,-3.4602254676408,56.2886751531321));
#7426=CARTESIAN_POINT('Ctrl Pts',(2.27209891769834,-3.39690790169264,56.2944945044042));
#7427=CARTESIAN_POINT('Ctrl Pts',(2.37036749133301,-3.32909005218638,56.3003138556764));
#7428=CARTESIAN_POINT('Ctrl Pts',(2.46557079210723,-3.25702098075952,56.3061332069485));
#7429=CARTESIAN_POINT('Ctrl Pts',(2.56067972621684,-3.185023345069,56.3119467900092));
#7430=CARTESIAN_POINT('Ctrl Pts',(2.65272910873421,-3.10878311546493,56.3177603730699));
#7431=CARTESIAN_POINT('Ctrl Pts',(2.74132234518034,-3.02859320474292,56.3235739561306));
#7432=CARTESIAN_POINT('Ctrl Pts',(2.83267648640232,-2.94590426907986,56.3295687127197));
#7433=CARTESIAN_POINT('Ctrl Pts',(2.92035516540868,-2.85901568002512,56.3355634693088));
#7434=CARTESIAN_POINT('Ctrl Pts',(3.00395912684207,-2.76829452267316,56.3415582258978));
#7435=CARTESIAN_POINT('Ctrl Pts',(3.08494671345783,-2.68041247183545,56.3473653773794));
#7436=CARTESIAN_POINT('Ctrl Pts',(3.16211051804336,-2.58893447666136,56.3531725288609));
#7437=CARTESIAN_POINT('Ctrl Pts',(3.23512474935081,-2.49423191707144,56.3589796803424));
#7438=CARTESIAN_POINT('Ctrl Pts',(3.3081285324509,-2.39954290925029,56.3647860008308));
#7439=CARTESIAN_POINT('Ctrl Pts',(3.37698367428118,-2.30163057759057,56.3705923213192));
#7440=CARTESIAN_POINT('Ctrl Pts',(3.44140523452848,-2.20089868275665,56.3763986418076));
#7441=CARTESIAN_POINT('Ctrl Pts',(3.50583273110447,-2.10015750566328,56.3822054973378));
#7442=CARTESIAN_POINT('Ctrl Pts',(3.56582561408171,-1.99659659238912,56.388012352868));
#7443=CARTESIAN_POINT('Ctrl Pts',(3.62114312018653,-1.89064737672729,56.3938192083982));
#7444=CARTESIAN_POINT('Ctrl Pts',(3.67647873682983,-1.7846634740833,56.3996279650495));
#7445=CARTESIAN_POINT('Ctrl Pts',(3.72713574371208,-1.67629007528272,56.4054367217009));
#7446=CARTESIAN_POINT('Ctrl Pts',(3.77292032486235,-1.56598123304226,56.4112454783522));
#7447=CARTESIAN_POINT('Ctrl Pts',(3.81875522050688,-1.4555511680349,56.4170606184769));
#7448=CARTESIAN_POINT('Ctrl Pts',(3.85970684631127,-1.34318179103272,56.4228757586015));
#7449=CARTESIAN_POINT('Ctrl Pts',(3.89563029261868,-1.22934520100404,56.4286908987262));
#7450=CARTESIAN_POINT('Ctrl Pts',(3.9315773991796,-1.11543363480088,56.4345098688757));
#7451=CARTESIAN_POINT('Ctrl Pts',(3.96248962543841,-1.00005332399803,56.4403288390251));
#7452=CARTESIAN_POINT('Ctrl Pts',(3.98827289048495,-0.883687926262892,56.4461478091746));
#7453=CARTESIAN_POINT('Ctrl Pts',(4.0140924376858,-0.767158779394006,56.4519749677662));
#7454=CARTESIAN_POINT('Ctrl Pts',(4.03476854853154,-0.649642179103727,56.4578021263577));
#7455=CARTESIAN_POINT('Ctrl Pts',(4.05025878816471,-0.531628393612036,56.4636292849493));
#7456=CARTESIAN_POINT('Ctrl Pts',(4.05364263184212,-0.505848275851416,56.4649022280556));
#7457=CARTESIAN_POINT('Ctrl Pts',(4.05677920100932,-0.480044436119279,56.466175171162));
#7458=CARTESIAN_POINT('Ctrl Pts',(4.05966838410138,-0.45422198441695,56.4674481142684));
#7459=CARTESIAN_POINT('Ctrl Pts',(4.0728930390211,-0.336024901690661,56.4732747554947));
#7460=CARTESIAN_POINT('Ctrl Pts',(4.08097250548031,-0.217061679068132,56.4791013967209));
#7461=CARTESIAN_POINT('Ctrl Pts',(4.08382868912331,-0.097817370100766,56.4849280379471));
#7462=CARTESIAN_POINT('Ctrl Pts',(4.08668129964938,0.0212777629340403,56.4907473899816));
#7463=CARTESIAN_POINT('Ctrl Pts',(4.08432361485388,0.140652878697699,56.496566742016));
#7464=CARTESIAN_POINT('Ctrl Pts',(4.07672913418456,0.259816409202425,56.5023860940504));
#7465=CARTESIAN_POINT('Ctrl Pts',(4.06914218125131,0.378861823453182,56.5081996778766));
#7466=CARTESIAN_POINT('Ctrl Pts',(4.05632878498824,0.497695664977626,56.5140132617028));
#7467=CARTESIAN_POINT('Ctrl Pts',(4.03831448513832,0.615825559003558,56.5198268455289));
#7468=CARTESIAN_POINT('Ctrl Pts',(4.01973879399759,0.737636811408265,56.5258216018323));
#7469=CARTESIAN_POINT('Ctrl Pts',(3.99563272050162,0.858699081083083,56.5318163581356));
#7470=CARTESIAN_POINT('Ctrl Pts',(3.96608220262526,0.97847685819296,56.537811114439));
#7471=CARTESIAN_POINT('Ctrl Pts',(3.93745645911073,1.09450622663358,56.5436182666889));
#7472=CARTESIAN_POINT('Ctrl Pts',(3.90372205868959,1.20932987424057,56.5494254189388));
#7473=CARTESIAN_POINT('Ctrl Pts',(3.86500904691189,1.3224711971492,56.5552325711887));
#7474=CARTESIAN_POINT('Ctrl Pts',(3.82630157489878,1.43559632973149,56.5610388924452));
#7475=CARTESIAN_POINT('Ctrl Pts',(3.78261704040561,1.54703923064694,56.5668452137017));
#7476=CARTESIAN_POINT('Ctrl Pts',(3.73413503207612,1.65633950693145,56.5726515349582));
#7477=CARTESIAN_POINT('Ctrl Pts',(3.68564855622843,1.76564985501351,56.5784583912554));
#7478=CARTESIAN_POINT('Ctrl Pts',(3.63236389294896,1.87281681311143,56.5842652475526));
#7479=CARTESIAN_POINT('Ctrl Pts',(3.57450808220949,1.97740157029851,56.5900721038498));
#7480=CARTESIAN_POINT('Ctrl Pts',(3.51663332993176,2.08202056771409,56.5958808612662));
#7481=CARTESIAN_POINT('Ctrl Pts',(3.45418465111976,2.18405532623511,56.6016896186825));
#7482=CARTESIAN_POINT('Ctrl Pts',(3.38743384960093,2.28309371568007,56.6074983760989));
#7483=CARTESIAN_POINT('Ctrl Pts',(3.32060969306293,2.3822409422145,56.6133135169818));
#7484=CARTESIAN_POINT('Ctrl Pts',(3.24947420514158,2.47838488878098,56.6191286578648));
#7485=CARTESIAN_POINT('Ctrl Pts',(3.17434122017362,2.57114426236776,56.6249437987477));
#7486=CARTESIAN_POINT('Ctrl Pts',(3.09915875042669,2.66396472998802,56.6307627696523));
#7487=CARTESIAN_POINT('Ctrl Pts',(3.01997380978192,2.75339588044843,56.636581740557));
#7488=CARTESIAN_POINT('Ctrl Pts',(2.93713791238661,2.83909244013315,56.6424007114616));
#7489=CARTESIAN_POINT('Ctrl Pts',(2.85418544865644,2.92490959166497,56.6482278707982));
#7490=CARTESIAN_POINT('Ctrl Pts',(2.76757206935306,3.00698138434765,56.6540550301348));
#7491=CARTESIAN_POINT('Ctrl Pts',(2.6776832921065,3.08500197523011,56.6598821894714));
#7492=CARTESIAN_POINT('Ctrl Pts',(2.65804719944135,3.10204547720317,56.6611551252506));
#7493=CARTESIAN_POINT('Ctrl Pts',(2.63825491743007,3.11889581892209,56.6624280610299));
#7494=CARTESIAN_POINT('Ctrl Pts',(2.61831064663882,3.13555008853276,56.6637009968091));
#7495=CARTESIAN_POINT('Ctrl Pts',(2.52701926482561,3.21178207022621,56.6695276358204));
#7496=CARTESIAN_POINT('Ctrl Pts',(2.43225059821607,3.28414515213955,56.6753542748318));
#7497=CARTESIAN_POINT('Ctrl Pts',(2.33436614355047,3.35230662497411,56.6811809138431));
#7498=CARTESIAN_POINT('Ctrl Pts',(2.23660414347771,3.42038282701228,56.6870002636612));
#7499=CARTESIAN_POINT('Ctrl Pts',(2.13573444020168,3.48426764386979,56.6928196134793));
#7500=CARTESIAN_POINT('Ctrl Pts',(2.03215242496763,3.54366780634108,56.6986389632974));
#7501=CARTESIAN_POINT('Ctrl Pts',(1.92867308142941,3.60300909068183,56.7044525449084));
#7502=CARTESIAN_POINT('Ctrl Pts',(1.8224871262917,3.6578743624604,56.7102661265194));
#7503=CARTESIAN_POINT('Ctrl Pts',(1.71401933092749,3.70801331351532,56.7160797081304));
#7504=CARTESIAN_POINT('Ctrl Pts',(1.6021712253028,3.75971480403306,56.7220744652645));
#7505=CARTESIAN_POINT('Ctrl Pts',(1.4878970886374,3.8063903121024,56.7280692223986));
#7506=CARTESIAN_POINT('Ctrl Pts',(1.37169098913703,3.84781611181203,56.7340639795328));
#7507=CARTESIAN_POINT('Ctrl Pts',(1.25912158196543,3.88794548311847,56.7398711295845));
#7508=CARTESIAN_POINT('Ctrl Pts',(1.14473974319271,3.92314868019171,56.7456782796363));
#7509=CARTESIAN_POINT('Ctrl Pts',(1.02901473885685,3.95327126152701,56.751485429688));
#7510=CARTESIAN_POINT('Ctrl Pts',(0.913306294372153,3.98338953242425,56.7572917487565));
#7511=CARTESIAN_POINT('Ctrl Pts',(0.796255461136269,4.0084285307815,56.763098067825));
#7512=CARTESIAN_POINT('Ctrl Pts',(0.67834531354043,4.02828408079641,56.7689043868935));
#7513=CARTESIAN_POINT('Ctrl Pts',(0.560424300506985,4.04814146050319,56.7747112410152));
#7514=CARTESIAN_POINT('Ctrl Pts',(0.441644217837552,4.06281437445065,56.7805180951369));
#7515=CARTESIAN_POINT('Ctrl Pts',(0.322496314391145,4.07225013072676,56.7863249492585));
#7516=CARTESIAN_POINT('Ctrl Pts',(0.203309402536086,4.08168897622078,56.7921337045143));
#7517=CARTESIAN_POINT('Ctrl Pts',(0.0837548367256362,4.08588722180895,56.79794245977));
#7518=CARTESIAN_POINT('Ctrl Pts',(-0.0356736949816792,4.08484423050456,
56.8037512150258));
#7519=CARTESIAN_POINT('Ctrl Pts',(-0.155233472009372,4.08380009301067,56.8095663537808));
#7520=CARTESIAN_POINT('Ctrl Pts',(-0.274666530469003,4.07750322545559,56.8153814925358));
#7521=CARTESIAN_POINT('Ctrl Pts',(-0.393481717726974,4.06600505875419,56.8211966312908));
#7522=CARTESIAN_POINT('Ctrl Pts',(-0.512375160508561,4.05449931898846,56.8270156000842));
#7523=CARTESIAN_POINT('Ctrl Pts',(-0.630649518773443,4.03778551437724,56.8328345688775));
#7524=CARTESIAN_POINT('Ctrl Pts',(-0.747822897738731,4.0159663735666,56.8386535376709));
#7525=CARTESIAN_POINT('Ctrl Pts',(-0.865161163465148,3.99411652878983,56.8444806949362));
#7526=CARTESIAN_POINT('Ctrl Pts',(-0.981394961997653,3.96714710119714,56.8503078522015));
#7527=CARTESIAN_POINT('Ctrl Pts',(-1.09605652968294,3.93521093255995,56.8561350094667));
#7528=CARTESIAN_POINT('Ctrl Pts',(-1.12110462704494,3.92823439911861,56.8574079660944));
#7529=CARTESIAN_POINT('Ctrl Pts',(-1.14607776894025,3.9210210287919,56.8586809227221));
#7530=CARTESIAN_POINT('Ctrl Pts',(-1.17097120922268,3.91357271903456,56.8599538793497));
#7531=CARTESIAN_POINT('Ctrl Pts',(-1.28491471158784,3.87947994235032,56.8657805202186));
#7532=CARTESIAN_POINT('Ctrl Pts',(-1.3975494038024,3.84035259116033,56.8716071610874));
#7533=CARTESIAN_POINT('Ctrl Pts',(-1.50839836353142,3.79630865142651,56.8774338019562));
#7534=CARTESIAN_POINT('Ctrl Pts',(-1.61910864971283,3.75231981125689,56.8832531536185));
#7535=CARTESIAN_POINT('Ctrl Pts',(-1.72803727115572,3.70342676588168,56.8890725052809));
#7536=CARTESIAN_POINT('Ctrl Pts',(-1.83472150462477,3.6497975286949,56.8948918569432));
#7537=CARTESIAN_POINT('Ctrl Pts',(-1.94129999119695,3.59622144955436,56.9007054403831));
#7538=CARTESIAN_POINT('Ctrl Pts',(-2.04563815332672,3.53791870034244,56.9065190238231));
#7539=CARTESIAN_POINT('Ctrl Pts',(-2.1472928939353,3.47510549878057,56.9123326072631));
#7540=CARTESIAN_POINT('Ctrl Pts',(-2.25211557645087,3.41033480293611,56.9183273637059));
#7541=CARTESIAN_POINT('Ctrl Pts',(-2.3540844365402,3.34076808759735,56.9243221201487));
#7542=CARTESIAN_POINT('Ctrl Pts',(-2.45274032310717,3.26669403333158,56.9303168765915));
#7543=CARTESIAN_POINT('Ctrl Pts',(-2.54830879496111,3.19493811063354,56.9361240284231));
#7544=CARTESIAN_POINT('Ctrl Pts',(-2.64076820856344,3.11895301707606,56.9419311802547));
#7545=CARTESIAN_POINT('Ctrl Pts',(-2.72973088313847,3.03904496604444,56.9477383320863));
#7546=CARTESIAN_POINT('Ctrl Pts',(-2.81868082713901,2.95914834986908,56.9535446529134));
#7547=CARTESIAN_POINT('Ctrl Pts',(-2.90413472396558,2.87533016512985,56.9593509737406));
#7548=CARTESIAN_POINT('Ctrl Pts',(-2.98573920162111,2.78793587083759,56.9651572945677));
#7549=CARTESIAN_POINT('Ctrl Pts',(-3.0673511988152,2.70053352349744,56.970964150425));
#7550=CARTESIAN_POINT('Ctrl Pts',(-3.145112793257,2.60955470951155,56.9767710062822));
#7551=CARTESIAN_POINT('Ctrl Pts',(-3.21870904564205,2.51538010636604,56.9825778621395));
#7552=CARTESIAN_POINT('Ctrl Pts',(-3.29232939273705,2.42117467135514,56.9883866191059));
#7553=CARTESIAN_POINT('Ctrl Pts',(-3.3617814346649,2.32377168750201,56.9941953760723));
#7554=CARTESIAN_POINT('Ctrl Pts',(-3.42679230487315,2.22358258206485,57.0000041330387));
#7555=CARTESIAN_POINT('Ctrl Pts',(-3.49187461789024,2.12328337517719,57.0058192734593));
#7556=CARTESIAN_POINT('Ctrl Pts',(-3.55250579538409,2.02019227762957,57.0116344138799));
#7557=CARTESIAN_POINT('Ctrl Pts',(-3.60845779855021,1.91474732434391,57.0174495543005));
#7558=CARTESIAN_POINT('Ctrl Pts',(-3.66444665326855,1.80923292206657,57.023268524735));
#7559=CARTESIAN_POINT('Ctrl Pts',(-3.71575002121323,1.70136194389109,57.0290874951696));
#7560=CARTESIAN_POINT('Ctrl Pts',(-3.76218775725437,1.59159300047635,57.0349064656041));
#7561=CARTESIAN_POINT('Ctrl Pts',(-3.80869084023158,1.48166959078613,57.040733624463));
#7562=CARTESIAN_POINT('Ctrl Pts',(-3.85031448443054,1.36984326617582,57.0465607833219));
#7563=CARTESIAN_POINT('Ctrl Pts',(-3.88692813860055,1.25658849483641,57.0523879421808));
#7564=CARTESIAN_POINT('Ctrl Pts',(-3.89492637282128,1.23184804736342,57.0536608820839));
#7565=CARTESIAN_POINT('Ctrl Pts',(-3.90268572290362,1.20703947378128,57.0549338219871));
#7566=CARTESIAN_POINT('Ctrl Pts',(-3.9102051533923,1.18216777928697,57.0562067618903));
#7567=CARTESIAN_POINT('Ctrl Pts',(-3.95200512607574,1.04390782036895,57.0632829431598));
#7568=CARTESIAN_POINT('Ctrl Pts',(-3.98649403339853,0.903343379381015,57.0703591244293));
#7569=CARTESIAN_POINT('Ctrl Pts',(-4.01345712133074,0.761174707435549,57.0774353056988));
#7570=CARTESIAN_POINT('Ctrl Pts',(-4.04010251102195,0.620681167697328,57.0844281103777));
#7571=CARTESIAN_POINT('Ctrl Pts',(-4.05939836360981,0.478620981810488,57.0914209150566));
#7572=CARTESIAN_POINT('Ctrl Pts',(-4.07118374982388,0.335690147561718,57.0984137197356));
#7573=CARTESIAN_POINT('Ctrl Pts',(-4.08028542363988,0.22530684675577,57.1038141560124));
#7574=CARTESIAN_POINT('Ctrl Pts',(-4.08490857038048,0.114404670593976,57.1092145922892));
#7575=CARTESIAN_POINT('Ctrl Pts',(-4.08499865687907,0.00331259659225328,
57.114615028566));
#7576=CARTESIAN_POINT('Ctrl Pts',(-4.08499865687956,0.00331259598633898,
57.1146150285955));
#7577=CARTESIAN_POINT('Ctrl Pts',(-4.08509496503765,-0.115451870925616,
57.1203884371961));
#7578=CARTESIAN_POINT('Ctrl Pts',(-4.08000768476869,-0.234306500596084,
57.1261618457968));
#7579=CARTESIAN_POINT('Ctrl Pts',(-4.06973999589507,-0.352762477897,57.1319352543974));
#7580=CARTESIAN_POINT('Ctrl Pts',(-4.05947579674755,-0.471178195026294,
57.1377067007634));
#7581=CARTESIAN_POINT('Ctrl Pts',(-4.04403472462242,-0.589195117883106,
57.1434781471294));
#7582=CARTESIAN_POINT('Ctrl Pts',(-4.02347200102888,-0.706327159987976,
57.1492495934954));
#7583=CARTESIAN_POINT('Ctrl Pts',(-4.00291127450329,-0.823447826136383,
57.155020479334));
#7584=CARTESIAN_POINT('Ctrl Pts',(-3.9772299570893,-0.939683375421726,57.1607913651725));
#7585=CARTESIAN_POINT('Ctrl Pts',(-3.94653469569518,-1.0545562553388,57.1665622510111));
#7586=CARTESIAN_POINT('Ctrl Pts',(-3.91583496393095,-1.16944586501366,57.172333977305));
#7587=CARTESIAN_POINT('Ctrl Pts',(-3.88011994338986,-1.28297201157841,57.1781057035989));
#7588=CARTESIAN_POINT('Ctrl Pts',(-3.83954642655221,-1.39467137288686,57.1838774298928));
#7589=CARTESIAN_POINT('Ctrl Pts',(-3.7989314253598,-1.50648494110398,57.1896550574828));
#7590=CARTESIAN_POINT('Ctrl Pts',(-3.75344814687081,-1.61646760411179,57.1954326850729));
#7591=CARTESIAN_POINT('Ctrl Pts',(-3.70330200785827,-1.72417494431188,57.201210312663));
#7592=CARTESIAN_POINT('Ctrl Pts',(-3.65313037236189,-1.83193704762064,57.2069908778509));
#7593=CARTESIAN_POINT('Ctrl Pts',(-3.59829134461344,-1.93742115709853,57.2127714430389));
#7594=CARTESIAN_POINT('Ctrl Pts',(-3.53903603327882,-2.04020806663294,57.2185520082268));
#7595=CARTESIAN_POINT('Ctrl Pts',(-3.47968342473736,-2.14316375224787,57.2243420651013));
#7596=CARTESIAN_POINT('Ctrl Pts',(-3.41590026556235,-2.24341303986314,57.2301321219759));
#7597=CARTESIAN_POINT('Ctrl Pts',(-3.34798098080885,-2.34056581880155,57.2359221788504));
#7598=CARTESIAN_POINT('Ctrl Pts',(-3.28331766470203,-2.43306121061776,57.2414346673773));
#7599=CARTESIAN_POINT('Ctrl Pts',(-3.21490579880504,-2.52274987289102,57.2469471559041));
#7600=CARTESIAN_POINT('Ctrl Pts',(-3.14303145861862,-2.60932524805431,57.252459644431));
#7601=CARTESIAN_POINT('Ctrl Pts',(-3.0670668285439,-2.70082753288646,57.2582858426353));
#7602=CARTESIAN_POINT('Ctrl Pts',(-2.98698217106811,-2.78915537539435,57.2641120408397));
#7603=CARTESIAN_POINT('Ctrl Pts',(-2.9030726580768,-2.87391616821488,57.269938239044));
#7604=CARTESIAN_POINT('Ctrl Pts',(-2.81925555558232,-2.95858361301446,57.2757580207903));
#7605=CARTESIAN_POINT('Ctrl Pts',(-2.73162225463703,-3.03969152919456,57.2815778025366));
#7606=CARTESIAN_POINT('Ctrl Pts',(-2.6405085480883,-3.11687978713851,57.2873975842829));
#7607=CARTESIAN_POINT('Ctrl Pts',(-2.54949195014274,-3.19398577816353,57.2932111633304));
#7608=CARTESIAN_POINT('Ctrl Pts',(-2.45500263837319,-3.26718016273486,57.299024742378));
#7609=CARTESIAN_POINT('Ctrl Pts',(-2.35741300912399,-3.33613982087277,57.3048383214255));
#7610=CARTESIAN_POINT('Ctrl Pts',(-2.342804626218,-3.34646252728015,57.3057085674694));
#7611=CARTESIAN_POINT('Ctrl Pts',(-2.32812683662819,-3.35669041351151,57.3065788135133));
#7612=CARTESIAN_POINT('Ctrl Pts',(-2.31338095599002,-3.36682247118298,57.3074490595572));
#7613=CARTESIAN_POINT('',(-4.0849985609995,-0.00342879453927592,57.0103849714486));
#7614=CARTESIAN_POINT('Ctrl Pts',(-4.0849985609995,-0.00342879453927238,
57.0103849714486));
#7615=CARTESIAN_POINT('Ctrl Pts',(-4.08487555327701,-0.14997778241887,57.0175132393231));
#7616=CARTESIAN_POINT('Ctrl Pts',(-4.07686266535297,-0.296190803989647,
57.0246415071976));
#7617=CARTESIAN_POINT('Ctrl Pts',(-4.06109046469521,-0.441326678959767,
57.031769775072));
#7618=CARTESIAN_POINT('Ctrl Pts',(-4.04508411276519,-0.588617215191905,
57.0390038679375));
#7619=CARTESIAN_POINT('Ctrl Pts',(-4.02108639579918,-0.734798457853202,
57.0462379608029));
#7620=CARTESIAN_POINT('Ctrl Pts',(-3.98928273098583,-0.879117905777264,
57.0534720536683));
#7621=CARTESIAN_POINT('Ctrl Pts',(-3.9722369976399,-0.956468451394702,57.0573492929333));
#7622=CARTESIAN_POINT('Ctrl Pts',(-3.95294974235968,-1.03328454509797,57.0612265321982));
#7623=CARTESIAN_POINT('Ctrl Pts',(-3.93145514333248,-1.10945277320155,57.0651037714632));
#7624=CARTESIAN_POINT('Ctrl Pts',(-3.89916052089188,-1.22389194768726,57.0709291408043));
#7625=CARTESIAN_POINT('Ctrl Pts',(-3.86181362482941,-1.3371019646882,57.0767545101455));
#7626=CARTESIAN_POINT('Ctrl Pts',(-3.81952486936604,-1.4486044222956,57.0825798794866));
#7627=CARTESIAN_POINT('Ctrl Pts',(-3.77728515920383,-1.55997756250988,57.0883984927294));
#7628=CARTESIAN_POINT('Ctrl Pts',(-3.73011512835958,-1.66964670315502,57.0942171059721));
#7629=CARTESIAN_POINT('Ctrl Pts',(-3.67817543772244,-1.77714671575965,57.1000357192149));
#7630=CARTESIAN_POINT('Ctrl Pts',(-3.62628376199816,-1.88454735149711,57.1058489535228));
#7631=CARTESIAN_POINT('Ctrl Pts',(-3.56963137148317,-1.98978248202845,57.1116621878308));
#7632=CARTESIAN_POINT('Ctrl Pts',(-3.50842745286672,-2.09240574649639,57.1174754221388));
#7633=CARTESIAN_POINT('Ctrl Pts',(-3.44726571223187,-2.19495828931354,57.1232846503227));
#7634=CARTESIAN_POINT('Ctrl Pts',(-3.38155889132315,-2.29490219765928,57.1290938785066));
#7635=CARTESIAN_POINT('Ctrl Pts',(-3.31156236831528,-2.39181514351718,57.1349031066906));
#7636=CARTESIAN_POINT('Ctrl Pts',(-3.24158781145911,-2.48869767637199,57.1407105118355));
#7637=CARTESIAN_POINT('Ctrl Pts',(-3.16732646374444,-2.58255080514865,57.1465179169805));
#7638=CARTESIAN_POINT('Ctrl Pts',(-3.08907710604279,-2.67298103863875,57.1523253221255));
#7639=CARTESIAN_POINT('Ctrl Pts',(-3.01084488953364,-2.76339146261111,57.1581314551086));
#7640=CARTESIAN_POINT('Ctrl Pts',(-2.92862667062261,-2.85038017715329,57.1639375880917));
#7641=CARTESIAN_POINT('Ctrl Pts',(-2.84276106384955,-2.93358731485207,57.1697437210748));
#7642=CARTESIAN_POINT('Ctrl Pts',(-2.75686116856737,-3.01682767945981,57.1755521726073));
#7643=CARTESIAN_POINT('Ctrl Pts',(-2.66731126677953,-3.09628316419446,57.1813606241397));
#7644=CARTESIAN_POINT('Ctrl Pts',(-2.57448627963979,-3.17163134616028,57.1871690756721));
#7645=CARTESIAN_POINT('Ctrl Pts',(-2.49005837374548,-3.24016342370037,57.1924520863623));
#7646=CARTESIAN_POINT('Ctrl Pts',(-2.40292172968864,-3.30529801528073,57.1977350970524));
#7647=CARTESIAN_POINT('Ctrl Pts',(-2.31338095599003,-3.36682247118298,57.2030181077425));
#7648=CARTESIAN_POINT('Ctrl Pts',(-2.31338095599003,-3.36682247118298,55.9532017097085));
#7649=CARTESIAN_POINT('Ctrl Pts',(-2.21490120219679,-3.43448899917066,55.9590093245328));
#7650=CARTESIAN_POINT('Ctrl Pts',(-2.1133988742849,-3.49786634484393,55.9648169393572));
#7651=CARTESIAN_POINT('Ctrl Pts',(-2.00928649021487,-3.55668283661054,55.9706245541816));
#7652=CARTESIAN_POINT('Ctrl Pts',(-1.90519567776754,-3.61548714186179,55.976430965694));
#7653=CARTESIAN_POINT('Ctrl Pts',(-1.79849623950041,-3.66973227196316,55.9822373772064));
#7654=CARTESIAN_POINT('Ctrl Pts',(-1.68962721947816,-3.71919142545776,55.9880437887188));
#7655=CARTESIAN_POINT('Ctrl Pts',(-1.58075514551467,-3.76865196635667,55.9938503631099));
#7656=CARTESIAN_POINT('Ctrl Pts',(-1.46971374017094,-3.8133260951914,55.999656937501));
#7657=CARTESIAN_POINT('Ctrl Pts',(-1.35696345988667,-3.85303454027243,56.0054635118921));
#7658=CARTESIAN_POINT('Ctrl Pts',(-1.24418349287064,-3.89275344044018,56.0112716151327));
#7659=CARTESIAN_POINT('Ctrl Pts',(-1.12969414064907,-3.92750392128263,56.0170797183733));
#7660=CARTESIAN_POINT('Ctrl Pts',(-1.01397188971186,-3.95715630306337,56.0228878216139));
#7661=CARTESIAN_POINT('Ctrl Pts',(-0.898125969859754,-3.9868403734593,56.0287021318011));
#7662=CARTESIAN_POINT('Ctrl Pts',(-0.781044916144667,-4.01141536569325,
56.0345164419883));
#7663=CARTESIAN_POINT('Ctrl Pts',(-0.663216499412574,-4.03080251003531,
56.0403307521755));
#7664=CARTESIAN_POINT('Ctrl Pts',(-0.545317251504739,-4.05020130873262,
56.0461485575673));
#7665=CARTESIAN_POINT('Ctrl Pts',(-0.42667015005983,-4.06440599917684,56.0519663629591));
#7666=CARTESIAN_POINT('Ctrl Pts',(-0.307767521396112,-4.07338976195179,
56.0577841683509));
#7667=CARTESIAN_POINT('Ctrl Pts',(-0.18868894942546,-4.08238681823379,56.0636105825004));
#7668=CARTESIAN_POINT('Ctrl Pts',(-0.0693545020969998,-4.08614750752744,
56.0694369966499));
#7669=CARTESIAN_POINT('Ctrl Pts',(0.0497437624093115,-4.08469711950609,
56.0752634107994));
#7670=CARTESIAN_POINT('Ctrl Pts',(0.108177674612077,-4.0839855067328,56.0781220601196));
#7671=CARTESIAN_POINT('Ctrl Pts',(0.166554807916021,-4.08202025660109,56.0809807094398));
#7672=CARTESIAN_POINT('Ctrl Pts',(0.224817716291339,-4.07880889408189,56.08383935876));
#7673=CARTESIAN_POINT('Ctrl Pts',(0.343572058871225,-4.07226333610362,56.0896659992445));
#7674=CARTESIAN_POINT('Ctrl Pts',(0.462229299207039,-4.0605167693811,56.0954926397291));
#7675=CARTESIAN_POINT('Ctrl Pts',(0.580298148961136,-4.04357256127701,56.1013192802136));
#7676=CARTESIAN_POINT('Ctrl Pts',(0.698219293221433,-4.02664955057282,56.1071386315037));
#7677=CARTESIAN_POINT('Ctrl Pts',(0.815553110801814,-4.00454188929853,56.1129579827937));
#7678=CARTESIAN_POINT('Ctrl Pts',(0.931810439003805,-3.97730490480219,56.1187773340838));
#7679=CARTESIAN_POINT('Ctrl Pts',(1.04795253156214,-3.95009491792818,56.1245909171638));
#7680=CARTESIAN_POINT('Ctrl Pts',(1.16301986270179,-3.91776581515896,56.1304045002437));
#7681=CARTESIAN_POINT('Ctrl Pts',(1.27653109809025,-3.88042437828757,56.1362180833237));
#7682=CARTESIAN_POINT('Ctrl Pts',(1.39357977807922,-3.84191923930526,56.1422128399061));
#7683=CARTESIAN_POINT('Ctrl Pts',(1.50897334874723,-3.79808430442617,56.1482075964884));
#7684=CARTESIAN_POINT('Ctrl Pts',(1.62219794591353,-3.7490930668995,56.1542023530708));
#7685=CARTESIAN_POINT('Ctrl Pts',(1.73187919496825,-3.7016350033767,56.1600095045749));
#7686=CARTESIAN_POINT('Ctrl Pts',(1.83952479976645,-3.64933872967957,56.165816656079));
#7687=CARTESIAN_POINT('Ctrl Pts',(1.94468629728686,-3.59241147492109,56.1716238075831));
#7688=CARTESIAN_POINT('Ctrl Pts',(2.04983274640438,-3.53549236634049,56.1774301280952));
#7689=CARTESIAN_POINT('Ctrl Pts',(2.15249543666421,-3.47394378873973,56.1832364486074));
#7690=CARTESIAN_POINT('Ctrl Pts',(2.25225010197143,-3.40801914287019,56.1890427691195));
#7691=CARTESIAN_POINT('Ctrl Pts',(2.35201395950751,-3.34208842215263,56.1948496246746));
#7692=CARTESIAN_POINT('Ctrl Pts',(2.44886891906241,-3.27178105626694,56.2006564802296));
#7693=CARTESIAN_POINT('Ctrl Pts',(2.54241986169742,-3.19739366466603,56.2064633357847));
#7694=CARTESIAN_POINT('Ctrl Pts',(2.63600143223026,-3.12298191917445,56.212272092462));
#7695=CARTESIAN_POINT('Ctrl Pts',(2.72627651549295,-3.04448774504516,56.2180808491394));
#7696=CARTESIAN_POINT('Ctrl Pts',(2.81288372255131,-2.96224748517167,56.2238896058167));
#7697=CARTESIAN_POINT('Ctrl Pts',(2.89958610573034,-2.87991684819028,56.2297047459688));
#7698=CARTESIAN_POINT('Ctrl Pts',(2.98261227131772,-2.79383218936243,56.235519886121));
#7699=CARTESIAN_POINT('Ctrl Pts',(3.06163820637459,-2.70436619067525,56.2413350262731));
#7700=CARTESIAN_POINT('Ctrl Pts',(3.14071619028187,-2.61484126699872,56.247153996451));
#7701=CARTESIAN_POINT('Ctrl Pts',(3.21578844081482,-2.52193088457491,56.2529729666288));
#7702=CARTESIAN_POINT('Ctrl Pts',(3.2865727106159,-2.42603891515261,56.2587919368066));
#7703=CARTESIAN_POINT('Ctrl Pts',(3.35745658789958,-2.33001200674313,56.2646190954276));
#7704=CARTESIAN_POINT('Ctrl Pts',(3.42404021489688,-2.23099547466168,56.2704462540486));
#7705=CARTESIAN_POINT('Ctrl Pts',(3.48608586470021,-2.12942018961438,56.2762734126696));
#7706=CARTESIAN_POINT('Ctrl Pts',(3.49963973771141,-2.10723106726703,56.2775463555466));
#7707=CARTESIAN_POINT('Ctrl Pts',(3.51297723549247,-2.08491992389572,56.2788192984236));
#7708=CARTESIAN_POINT('Ctrl Pts',(3.52609618252348,-2.0624913846107,56.2800922413006));
#7709=CARTESIAN_POINT('Ctrl Pts',(3.58614553017031,-1.9598292464411,56.2859188818971));
#7710=CARTESIAN_POINT('Ctrl Pts',(3.64180322194183,-1.85437904773052,56.2917455224936));
#7711=CARTESIAN_POINT('Ctrl Pts',(3.69280105526522,-1.74655242298422,56.2975721630902));
#7712=CARTESIAN_POINT('Ctrl Pts',(3.74373508971591,-1.6388606905786,56.3033915144927));
#7713=CARTESIAN_POINT('Ctrl Pts',(3.79002068806166,-1.52879881092131,56.3092108658952));
#7714=CARTESIAN_POINT('Ctrl Pts',(3.83143415942334,-1.41680530843302,56.3150302172977));
#7715=CARTESIAN_POINT('Ctrl Pts',(3.8728065812636,-1.30492281522571,56.3208438004905));
#7716=CARTESIAN_POINT('Ctrl Pts',(3.9093163431132,-1.19111288862575,56.3266573836832));
#7717=CARTESIAN_POINT('Ctrl Pts',(3.94078698993878,-1.07583590752924,56.332470966876));
#7718=CARTESIAN_POINT('Ctrl Pts',(3.97323838172722,-0.956966457578475,56.3384657234162));
#7719=CARTESIAN_POINT('Ctrl Pts',(4.00033124895871,-0.836537416436334,56.3444604799564));
#7720=CARTESIAN_POINT('Ctrl Pts',(4.02192683516748,-0.715073095955729,56.3504552364966));
#7721=CARTESIAN_POINT('Ctrl Pts',(4.04284659104576,-0.597409981474317,56.3562623881136));
#7722=CARTESIAN_POINT('Ctrl Pts',(4.05860793115304,-0.478775850041155,56.3620695397305));
#7723=CARTESIAN_POINT('Ctrl Pts',(4.06913631512704,-0.359659073171202,56.3678766913475));
#7724=CARTESIAN_POINT('Ctrl Pts',(4.07966319250976,-0.24055934168033,56.3736830119723));
#7725=CARTESIAN_POINT('Ctrl Pts',(4.08495856713286,-0.120977508233191,56.3794893325971));
#7726=CARTESIAN_POINT('Ctrl Pts',(4.08499975761303,-0.00140723185226689,
56.385295653222));
#7727=CARTESIAN_POINT('Ctrl Pts',(4.08504095188883,0.118174062727738,56.3911025088895));
#7728=CARTESIAN_POINT('Ctrl Pts',(4.07982699924621,0.237743390297444,56.396909364557));
#7729=CARTESIAN_POINT('Ctrl Pts',(4.06938734499027,0.356807562185923,56.4027162202245));
#7730=CARTESIAN_POINT('Ctrl Pts',(4.05894427286833,0.475910714808278,56.4085249770138));
#7731=CARTESIAN_POINT('Ctrl Pts',(4.04327213216008,0.594507976797068,56.4143337338031));
#7732=CARTESIAN_POINT('Ctrl Pts',(4.02245210756335,0.712112380428253,56.4201424905924));
#7733=CARTESIAN_POINT('Ctrl Pts',(4.00160920301424,0.82984602421194,56.4259576308554));
#7734=CARTESIAN_POINT('Ctrl Pts',(3.97560719379228,0.946584230022544,56.4317727711183));
#7735=CARTESIAN_POINT('Ctrl Pts',(3.94457819240187,1.06185115907436,56.4375879113813));
#7736=CARTESIAN_POINT('Ctrl Pts',(3.91352875438408,1.17719400636953,56.4434068816694));
#7737=CARTESIAN_POINT('Ctrl Pts',(3.87744585313556,1.29106325917657,56.4492258519575));
#7738=CARTESIAN_POINT('Ctrl Pts',(3.8365106554235,1.40300070948734,56.4550448222456));
#7739=CARTESIAN_POINT('Ctrl Pts',(3.79551785379579,1.51509567791955,56.4608719809752));
#7740=CARTESIAN_POINT('Ctrl Pts',(3.74965928412593,1.62525304328815,56.4666991397049));
#7741=CARTESIAN_POINT('Ctrl Pts',(3.69916319162955,1.73303683795039,56.4725262984345));
#7742=CARTESIAN_POINT('Ctrl Pts',(3.68813232908199,1.7565821889864,56.4737992402368));
#7743=CARTESIAN_POINT('Ctrl Pts',(3.67688033094081,1.78001437548934,56.475072182039));
#7744=CARTESIAN_POINT('Ctrl Pts',(3.66540985485052,1.80332903153159,56.4763451238413));
#7745=CARTESIAN_POINT('Ctrl Pts',(3.6129060102169,1.91004727660646,56.4821717641731));
#7746=CARTESIAN_POINT('Ctrl Pts',(3.55565409674372,2.01464048979338,56.487998404505));
#7747=CARTESIAN_POINT('Ctrl Pts',(3.49384950354949,2.11665789549162,56.4938250448369));
#7748=CARTESIAN_POINT('Ctrl Pts',(3.43212222861171,2.21854767624277,56.4996443959747));
#7749=CARTESIAN_POINT('Ctrl Pts',(3.36585381195152,2.31786771313676,56.5054637471126));
#7750=CARTESIAN_POINT('Ctrl Pts',(3.29528662535605,2.41418952378423,56.5112830982504));
#7751=CARTESIAN_POINT('Ctrl Pts',(3.22478938578709,2.51041585911848,56.5170966811789));
#7752=CARTESIAN_POINT('Ctrl Pts',(3.15000209294918,2.6036495534604,56.5229102641074));
#7753=CARTESIAN_POINT('Ctrl Pts',(3.07121140404016,2.69348946752974,56.5287238470358));
#7754=CARTESIAN_POINT('Ctrl Pts',(2.98996529277377,2.7861291405128,56.5347186036752));
#7755=CARTESIAN_POINT('Ctrl Pts',(2.90446240423398,2.87515966400845,56.5407133603147));
#7756=CARTESIAN_POINT('Ctrl Pts',(2.81506351709993,2.96017607494774,56.5467081169541));
#7757=CARTESIAN_POINT('Ctrl Pts',(2.72846235882188,3.0425319061668,56.5525152683092));
#7758=CARTESIAN_POINT('Ctrl Pts',(2.63820573231969,3.12112081890557,56.5583224196644));
#7759=CARTESIAN_POINT('Ctrl Pts',(2.54465986263442,3.19561123785378,56.5641295710195));
#7760=CARTESIAN_POINT('Ctrl Pts',(2.45112737915943,3.27009099738522,56.5699358913839));
#7761=CARTESIAN_POINT('Ctrl Pts',(2.35430690753955,3.34047317556109,56.5757422117484));
#7762=CARTESIAN_POINT('Ctrl Pts',(2.25459769021904,3.4064665351738,56.5815485321128));
#7763=CARTESIAN_POINT('Ctrl Pts',(2.15487928483334,3.47246597598247,56.5873553875215));
#7764=CARTESIAN_POINT('Ctrl Pts',(2.0522719445747,3.53407556904849,56.5931622429303));
#7765=CARTESIAN_POINT('Ctrl Pts',(1.9472032744155,3.59104781478966,56.598969098339));
#7766=CARTESIAN_POINT('Ctrl Pts',(1.84210020551024,3.64803871284469,56.6047778548715));
#7767=CARTESIAN_POINT('Ctrl Pts',(1.73453456238059,3.7003890498009,56.610586611404));
#7768=CARTESIAN_POINT('Ctrl Pts',(1.62495730238763,3.74789791288625,56.6163953679365));
#7769=CARTESIAN_POINT('Ctrl Pts',(1.51525962350574,3.79545898538537,56.6222105079468));
#7770=CARTESIAN_POINT('Ctrl Pts',(1.40354628961632,3.83816780190019,56.6280256479571));
#7771=CARTESIAN_POINT('Ctrl Pts',(1.29028706908165,3.87587206694967,56.6338407879674));
#7772=CARTESIAN_POINT('Ctrl Pts',(1.17695325259555,3.91360116516956,56.639659758005));
#7773=CARTESIAN_POINT('Ctrl Pts',(1.06207191299317,3.94631903595772,56.6454787280426));
#7774=CARTESIAN_POINT('Ctrl Pts',(0.946125173030944,3.97392402506102,56.6512976980801));
#7775=CARTESIAN_POINT('Ctrl Pts',(0.830015272978565,4.00156785986634,56.6571248565642));
#7776=CARTESIAN_POINT('Ctrl Pts',(0.712837379361212,4.02408437672899,56.6629520150482));
#7777=CARTESIAN_POINT('Ctrl Pts',(0.59508103460896,4.04142345742793,56.6687791735323));
#7778=CARTESIAN_POINT('Ctrl Pts',(0.569357130535747,4.04521118410674,56.6700521178155));
#7779=CARTESIAN_POINT('Ctrl Pts',(0.543605629490371,4.04875203824814,56.6713250620987));
#7780=CARTESIAN_POINT('Ctrl Pts',(0.5178316391104,4.05204582816338,56.6725980063819));
#7781=CARTESIAN_POINT('Ctrl Pts',(0.399856502752466,4.06712247359762,56.6784246468506));
#7782=CARTESIAN_POINT('Ctrl Pts',(0.281034631442562,4.07706657969223,56.6842512873192));
#7783=CARTESIAN_POINT('Ctrl Pts',(0.161849794244976,4.08179245480498,56.6900779277879));
#7784=CARTESIAN_POINT('Ctrl Pts',(0.0428140586837499,4.08651241779225,56.6958972790606));
#7785=CARTESIAN_POINT('Ctrl Pts',(-0.0765833356078236,4.08602711839325,
56.7017166303334));
#7786=CARTESIAN_POINT('Ctrl Pts',(-0.195851296802997,4.08030235026041,56.7075359816061));
#7787=CARTESIAN_POINT('Ctrl Pts',(-0.315001038150048,4.0745832565871,56.7133495646674));
#7788=CARTESIAN_POINT('Ctrl Pts',(-0.434021196577892,4.06363504565181,56.7191631477287));
#7789=CARTESIAN_POINT('Ctrl Pts',(-0.552419057446783,4.04747553234971,56.7249767307899));
#7790=CARTESIAN_POINT('Ctrl Pts',(-0.674506649396676,4.030812426685,56.7309714873788));
#7791=CARTESIAN_POINT('Ctrl Pts',(-0.795932080920315,4.00860787223188,56.7369662439677));
#7792=CARTESIAN_POINT('Ctrl Pts',(-0.916158560141836,3.98093939826755,56.7429610005565));
#7793=CARTESIAN_POINT('Ctrl Pts',(-1.03262256775463,3.9541368055003,56.7487681520386));
#7794=CARTESIAN_POINT('Ctrl Pts',(-1.14796111953944,3.92220727662307,56.7545753035208));
#7795=CARTESIAN_POINT('Ctrl Pts',(-1.2616956309075,3.88527336682362,56.7603824550029));
#7796=CARTESIAN_POINT('Ctrl Pts',(-1.37541386706858,3.84834474220119,56.7661887754919));
#7797=CARTESIAN_POINT('Ctrl Pts',(-1.48752813154241,3.8064132868009,56.771995095981));
#7798=CARTESIAN_POINT('Ctrl Pts',(-1.59757527168778,3.75965134703894,56.77780141647));
#7799=CARTESIAN_POINT('Ctrl Pts',(-1.70763255247513,3.71288509825006,56.7836082720008));
#7800=CARTESIAN_POINT('Ctrl Pts',(-1.81562195486502,3.66128763958747,56.7894151275316));
#7801=CARTESIAN_POINT('Ctrl Pts',(-1.92110116144567,3.60507910141957,56.7952219830624));
#7802=CARTESIAN_POINT('Ctrl Pts',(-2.02661490113119,3.54885216099584,56.8010307397144));
#7803=CARTESIAN_POINT('Ctrl Pts',(-2.12961645085554,3.48801133037091,56.8068394963664));
#7804=CARTESIAN_POINT('Ctrl Pts',(-2.22968946866473,3.42282191668302,56.8126482530184));
#7805=CARTESIAN_POINT('Ctrl Pts',(-2.32987246068705,3.35756086375977,56.8184633931437));
#7806=CARTESIAN_POINT('Ctrl Pts',(-2.42712015516095,3.28794191184065,56.824278533269));
#7807=CARTESIAN_POINT('Ctrl Pts',(-2.52104638436984,3.2142728770059,56.8300936733943));
#7808=CARTESIAN_POINT('Ctrl Pts',(-2.6150344761951,3.14055532154725,56.8359126435444));
#7809=CARTESIAN_POINT('Ctrl Pts',(-2.70569643715789,3.0627826355294,56.8417316136945));
#7810=CARTESIAN_POINT('Ctrl Pts',(-2.79268152359938,2.98130087507897,56.8475505838445));
#7811=CARTESIAN_POINT('Ctrl Pts',(-2.87978901526491,2.89970445367284,56.8533777424367));
#7812=CARTESIAN_POINT('Ctrl Pts',(-2.96320902182736,2.81438883135466,56.8592049010289));
#7813=CARTESIAN_POINT('Ctrl Pts',(-3.04262969218861,2.7257346819183,56.8650320596211));
#7814=CARTESIAN_POINT('Ctrl Pts',(-3.05997914179986,2.70636817831818,56.8663050027216));
#7815=CARTESIAN_POINT('Ctrl Pts',(-3.0771379021545,2.68684247351958,56.867577945822));
#7816=CARTESIAN_POINT('Ctrl Pts',(-3.09410299583021,2.66716172197985,56.8688508889225));
#7817=CARTESIAN_POINT('Ctrl Pts',(-3.17269838390856,2.57598531384996,56.8747481423593));
#7818=CARTESIAN_POINT('Ctrl Pts',(-3.24739993934555,2.48116956296244,56.880645395796));
#7819=CARTESIAN_POINT('Ctrl Pts',(-3.31785016116441,2.38308524985181,56.8865426492328));
#7820=CARTESIAN_POINT('Ctrl Pts',(-3.38677126205226,2.28712985517905,56.8923119028786));
#7821=CARTESIAN_POINT('Ctrl Pts',(-3.45162340496512,2.18804667540133,56.8980811565243));
#7822=CARTESIAN_POINT('Ctrl Pts',(-3.51210959684272,2.08621935082706,56.9038504101701));
#7823=CARTESIAN_POINT('Ctrl Pts',(-3.57254048409481,1.98448513051142,56.909614388787));
#7824=CARTESIAN_POINT('Ctrl Pts',(-3.62861314476093,1.88001210781938,56.9153783674039));
#7825=CARTESIAN_POINT('Ctrl Pts',(-3.68007284767165,1.77321426675681,56.9211423460207));
#7826=CARTESIAN_POINT('Ctrl Pts',(-3.73149813955135,1.66648784126047,56.9269024702732));
#7827=CARTESIAN_POINT('Ctrl Pts',(-3.77831642767281,1.5574400615493,56.9326625945256));
#7828=CARTESIAN_POINT('Ctrl Pts',(-3.82031842436584,1.44651033057178,56.9384227187781));
#7829=CARTESIAN_POINT('Ctrl Pts',(-3.86404662310433,1.33102159898496,56.9444195731636));
#7830=CARTESIAN_POINT('Ctrl Pts',(-3.90255395563487,1.21349332845696,56.9504164275492));
#7831=CARTESIAN_POINT('Ctrl Pts',(-3.93565938354699,1.09444516386089,56.9564132819347));
#7832=CARTESIAN_POINT('Ctrl Pts',(-3.96744507222734,0.980142823233796,56.9621710732874));
#7833=CARTESIAN_POINT('Ctrl Pts',(-3.99425118915626,0.864439880713943,56.9679288646401));
#7834=CARTESIAN_POINT('Ctrl Pts',(-4.01596853363508,0.747811297623225,56.9736866559928));
#7835=CARTESIAN_POINT('Ctrl Pts',(-4.03768679329499,0.631177799738453,56.9794446899821));
#7836=CARTESIAN_POINT('Ctrl Pts',(-4.0543157853813,0.51361899341479,56.9852027239713));
#7837=CARTESIAN_POINT('Ctrl Pts',(-4.06579771086683,0.395618470638135,56.9909607579606));
#7838=CARTESIAN_POINT('Ctrl Pts',(-4.07728567533725,0.27755588480637,56.996721820421));
#7839=CARTESIAN_POINT('Ctrl Pts',(-4.08362114071097,0.159051533025043,57.0024828828815));
#7840=CARTESIAN_POINT('Ctrl Pts',(-4.08479831537712,0.0405921506234354,
57.0082439453419));
#7841=CARTESIAN_POINT('Ctrl Pts',(-4.08494414274014,0.0259175064454967,
57.0089576206961));
#7842=CARTESIAN_POINT('Ctrl Pts',(-4.0850108764124,0.0112435507115259,57.0096712960503));
#7843=CARTESIAN_POINT('Ctrl Pts',(-4.08499856100026,-0.00342879363290059,
57.0103849714045));
#7844=CARTESIAN_POINT('Origin',(0.,0.,46.4896150285955));
#7845=CARTESIAN_POINT('',(-2.31338095599002,-3.36682247118298,54.7030792959875));
#7846=CARTESIAN_POINT('',(-2.31338095599002,-3.36682247118299,54.8073227890241));
#7847=CARTESIAN_POINT('',(-2.31338095599002,-3.36682247118298,46.4896150285955));
#7848=CARTESIAN_POINT('',(-4.08499967473006,-0.00163017032924335,55.8646150285584));
#7849=CARTESIAN_POINT('Ctrl Pts',(-2.31338095599002,-3.36682247118299,54.8073227890241));
#7850=CARTESIAN_POINT('Ctrl Pts',(-2.21482319399213,-3.43454259947083,54.8131297128475));
#7851=CARTESIAN_POINT('Ctrl Pts',(-2.11330224758641,-3.49792266475831,54.8189366366709));
#7852=CARTESIAN_POINT('Ctrl Pts',(-2.00924159562139,-3.55670819866134,54.8247435604943));
#7853=CARTESIAN_POINT('Ctrl Pts',(-1.90070329685815,-3.61802322716865,54.830800351615));
#7854=CARTESIAN_POINT('Ctrl Pts',(-1.7894022638471,-3.67433924177659,54.8368571427358));
#7855=CARTESIAN_POINT('Ctrl Pts',(-1.67584634546039,-3.7254213219993,54.8429139338566));
#7856=CARTESIAN_POINT('Ctrl Pts',(-1.56681507205789,-3.7744680324998,54.8487293916329));
#7857=CARTESIAN_POINT('Ctrl Pts',(-1.45570556469748,-3.81868979941789,54.8545448494092));
#7858=CARTESIAN_POINT('Ctrl Pts',(-1.34298565883407,-3.85792878630049,54.8603603071855));
#7859=CARTESIAN_POINT('Ctrl Pts',(-1.23018920423639,-3.89719442060405,54.8661797142725));
#7860=CARTESIAN_POINT('Ctrl Pts',(-1.11578056277697,-3.93147041932827,54.8719991213595));
#7861=CARTESIAN_POINT('Ctrl Pts',(-1.00024049472196,-3.96064943572621,54.8778185284466));
#7862=CARTESIAN_POINT('Ctrl Pts',(-0.884540722147535,-3.98986878463277,
54.8836459793718));
#7863=CARTESIAN_POINT('Ctrl Pts',(-0.767706799903252,-4.01397701072238,
54.889473430297));
#7864=CARTESIAN_POINT('Ctrl Pts',(-0.65022742237105,-4.03291821132002,54.8953008812222));
#7865=CARTESIAN_POINT('Ctrl Pts',(-0.635953228717375,-4.03521963963062,
54.8960089387959));
#7866=CARTESIAN_POINT('Ctrl Pts',(-0.621669508882911,-4.03744484934028,
54.8967169963696));
#7867=CARTESIAN_POINT('Ctrl Pts',(-0.607377140913246,-4.03959379253608,
54.8974250539433));
#7868=CARTESIAN_POINT('Ctrl Pts',(-0.489764544025958,-4.05727755147362,
54.9032516944387));
#7869=CARTESIAN_POINT('Ctrl Pts',(-0.371191835800804,-4.06984876630172,
54.9090783349341));
#7870=CARTESIAN_POINT('Ctrl Pts',(-0.252140770467798,-4.07721106050054,
54.9149049754295));
#7871=CARTESIAN_POINT('Ctrl Pts',(-0.133238639387124,-4.08456414438461,
54.9207243267306));
#7872=CARTESIAN_POINT('Ctrl Pts',(-0.0138597450321857,-4.08672124412869,
54.9265436780317));
#7873=CARTESIAN_POINT('Ctrl Pts',(0.10550569802293,-4.08363729384536,54.9323630293328));
#7874=CARTESIAN_POINT('Ctrl Pts',(0.224752824638586,-4.08055640041005,54.938176612424));
#7875=CARTESIAN_POINT('Ctrl Pts',(0.34398612108893,-4.0722448025657,54.9439901955153));
#7876=CARTESIAN_POINT('Ctrl Pts',(0.462712599148696,-4.05870940701463,54.9498037786065));
#7877=CARTESIAN_POINT('Ctrl Pts',(0.585139048412051,-4.04475219676319,54.9557985351847));
#7878=CARTESIAN_POINT('Ctrl Pts',(0.707026132368672,-4.02524024113901,54.961793291763));
#7879=CARTESIAN_POINT('Ctrl Pts',(0.827835474876989,-4.00023917116654,54.9677880483412));
#7880=CARTESIAN_POINT('Ctrl Pts',(0.944864106033258,-3.97602050615627,54.973595199857));
#7881=CARTESIAN_POINT('Ctrl Pts',(1.06088101671545,-3.94665125407904,54.9794023513727));
#7882=CARTESIAN_POINT('Ctrl Pts',(1.1754050273745,-3.91224334897802,54.9852095028885));
#7883=CARTESIAN_POINT('Ctrl Pts',(1.28991264987605,-3.87784036757959,54.9910158234124));
#7884=CARTESIAN_POINT('Ctrl Pts',(1.40292740676158,-3.83840028444088,54.9968221439364));
#7885=CARTESIAN_POINT('Ctrl Pts',(1.51398244476487,-3.79408515415031,55.0026284644603));
#7886=CARTESIAN_POINT('Ctrl Pts',(1.62504771631026,-3.74976594029218,55.0084353200273));
#7887=CARTESIAN_POINT('Ctrl Pts',(1.7341525311439,-3.70057093725805,55.0142421755943));
#7888=CARTESIAN_POINT('Ctrl Pts',(1.84084980866215,-3.64671043297223,55.0200490311613));
#7889=CARTESIAN_POINT('Ctrl Pts',(1.94758201809453,-3.59283229514829,55.0258577878507));
#7890=CARTESIAN_POINT('Ctrl Pts',(2.05190475874801,-3.53428580193233,55.0316665445401));
#7891=CARTESIAN_POINT('Ctrl Pts',(2.15339591934824,-3.47132698179447,55.0374753012294));
#7892=CARTESIAN_POINT('Ctrl Pts',(2.25499861264177,-3.40829897369252,55.0432904413937));
#7893=CARTESIAN_POINT('Ctrl Pts',(2.35376316806692,-3.34084917529051,55.049105581558));
#7894=CARTESIAN_POINT('Ctrl Pts',(2.44929670046909,-3.26927678134955,55.0549207217223));
#7895=CARTESIAN_POINT('Ctrl Pts',(2.5448931541213,-3.19765724768306,55.0607396919123));
#7896=CARTESIAN_POINT('Ctrl Pts',(2.63725403199957,-3.12190996881854,55.0665586621023));
#7897=CARTESIAN_POINT('Ctrl Pts',(2.72602101807498,-3.04237315413699,55.0723776322923));
#7898=CARTESIAN_POINT('Ctrl Pts',(2.81491291687529,-2.96272441540922,55.0782047909255));
#7899=CARTESIAN_POINT('Ctrl Pts',(2.9002005399884,-2.87927578204997,55.0840319495588));
#7900=CARTESIAN_POINT('Ctrl Pts',(2.98156368832814,-2.79240093332657,55.089859108192));
#7901=CARTESIAN_POINT('Ctrl Pts',(2.99933746753225,-2.77342312321095,55.091132050956));
#7902=CARTESIAN_POINT('Ctrl Pts',(3.01692412742201,-2.75428193099485,55.0924049937199));
#7903=CARTESIAN_POINT('Ctrl Pts',(3.03432059936808,-2.73498144422417,55.0936779364839));
#7904=CARTESIAN_POINT('Ctrl Pts',(3.11394946468215,-2.64663733248,55.0995045769786));
#7905=CARTESIAN_POINT('Ctrl Pts',(3.18984365620379,-2.55467215284154,55.1053312174733));
#7906=CARTESIAN_POINT('Ctrl Pts',(3.26165703567637,-2.45943456542816,55.111157857968));
#7907=CARTESIAN_POINT('Ctrl Pts',(3.33338057578459,-2.36431612133292,55.1169772092684));
#7908=CARTESIAN_POINT('Ctrl Pts',(3.40103321478146,-2.26593373506231,55.1227965605687));
#7909=CARTESIAN_POINT('Ctrl Pts',(3.46430694490073,-2.1646714280723,55.1286159118691));
#7910=CARTESIAN_POINT('Ctrl Pts',(3.52751795734966,-2.06350949347974,55.1344294949596));
#7911=CARTESIAN_POINT('Ctrl Pts',(3.5863584810659,-1.95947366116699,55.14024307805));
#7912=CARTESIAN_POINT('Ctrl Pts',(3.6405623278751,-1.85297893589125,55.1460566611405));
#7913=CARTESIAN_POINT('Ctrl Pts',(3.69645537389905,-1.7431654275973,55.152051417719));
#7914=CARTESIAN_POINT('Ctrl Pts',(3.74741775007967,-1.63073761136662,55.1580461742975));
#7915=CARTESIAN_POINT('Ctrl Pts',(3.79320721189438,-1.51618074372169,55.164040930876));
#7916=CARTESIAN_POINT('Ctrl Pts',(3.83756369894471,-1.40520891713023,55.1698480823909));
#7917=CARTESIAN_POINT('Ctrl Pts',(3.87706605204126,-1.29223971501255,55.1756552339059));
#7918=CARTESIAN_POINT('Ctrl Pts',(3.91154219895384,-1.17773622929898,55.1814623854208));
#7919=CARTESIAN_POINT('Ctrl Pts',(3.94601341239839,-1.06324912880639,55.1872687059438));
#7920=CARTESIAN_POINT('Ctrl Pts',(3.97545973254368,-0.94722857175979,55.1930750264669));
#7921=CARTESIAN_POINT('Ctrl Pts',(3.99975879488763,-0.830153348917576,55.19888134699));
#7922=CARTESIAN_POINT('Ctrl Pts',(4.02406009635076,-0.713067337783471,55.2046882025561));
#7923=CARTESIAN_POINT('Ctrl Pts',(4.04321311408866,-0.594926866941737,55.2104950581222));
#7924=CARTESIAN_POINT('Ctrl Pts',(4.0571466216387,-0.476220842178967,55.2163019136883));
#7925=CARTESIAN_POINT('Ctrl Pts',(4.07108469091791,-0.357475953925963,55.2221106703767));
#7926=CARTESIAN_POINT('Ctrl Pts',(4.07979980394908,-0.238165548319194,55.2279194270652));
#7927=CARTESIAN_POINT('Ctrl Pts',(4.08327265976366,-0.118782936597042,55.2337281837536));
#7928=CARTESIAN_POINT('Ctrl Pts',(4.0867493320383,0.000730869448708649,
55.2395433239169));
#7929=CARTESIAN_POINT('Ctrl Pts',(4.08497223630873,0.120316632144369,55.2453584640803));
#7930=CARTESIAN_POINT('Ctrl Pts',(4.07797419813884,0.239481605376798,55.2511736042436));
#7931=CARTESIAN_POINT('Ctrl Pts',(4.07097155085113,0.358725064234697,55.2569925744327));
#7932=CARTESIAN_POINT('Ctrl Pts',(4.05874115441113,0.477546776967526,55.2628115446217));
#7933=CARTESIAN_POINT('Ctrl Pts',(4.0413674454453,0.595461309318171,55.2686305148108));
#7934=CARTESIAN_POINT('Ctrl Pts',(4.0239692882311,0.713541770762001,55.274457673443));
#7935=CARTESIAN_POINT('Ctrl Pts',(4.00141345024314,0.830712105038716,55.2802848320752));
#7936=CARTESIAN_POINT('Ctrl Pts',(3.97383497965204,0.946499104328078,55.2861119907074));
#7937=CARTESIAN_POINT('Ctrl Pts',(3.96781046289726,0.971792773710525,55.2873849334798));
#7938=CARTESIAN_POINT('Ctrl Pts',(3.96154645001124,0.997020496498459,55.2886578762522));
#7939=CARTESIAN_POINT('Ctrl Pts',(3.95504465760098,1.02217745836129,55.2899308190246));
#7940=CARTESIAN_POINT('Ctrl Pts',(3.9252840054547,1.13732841117781,55.2957574595355));
#7941=CARTESIAN_POINT('Ctrl Pts',(3.89044289746043,1.25136182665304,55.3015841000464));
#7942=CARTESIAN_POINT('Ctrl Pts',(3.85062120473652,1.36379666286198,55.3074107405574));
#7943=CARTESIAN_POINT('Ctrl Pts',(3.81084932940806,1.47609084179809,55.313230091874));
#7944=CARTESIAN_POINT('Ctrl Pts',(3.76610939759966,1.5867900381358,55.3190494431907));
#7945=CARTESIAN_POINT('Ctrl Pts',(3.71655180890724,1.69542550756685,55.3248687945073));
#7946=CARTESIAN_POINT('Ctrl Pts',(3.66704334228296,1.80395329623552,55.3306823776141));
#7947=CARTESIAN_POINT('Ctrl Pts',(3.61272688731292,1.91042105863624,55.3364959607209));
#7948=CARTESIAN_POINT('Ctrl Pts',(3.55380175544378,2.01437784017911,55.3423095438277));
#7949=CARTESIAN_POINT('Ctrl Pts',(3.49304029128945,2.12157431229471,55.3483043004001));
#7950=CARTESIAN_POINT('Ctrl Pts',(3.42737834431585,2.22610032020434,55.3542990569725));
#7951=CARTESIAN_POINT('Ctrl Pts',(3.35708703013771,2.32748612715117,55.3602938135449));
#7952=CARTESIAN_POINT('Ctrl Pts',(3.2889954724853,2.42569907991174,55.3661009650761));
#7953=CARTESIAN_POINT('Ctrl Pts',(3.21656022671052,2.52096508523289,55.3719081166074));
#7954=CARTESIAN_POINT('Ctrl Pts',(3.14007263065266,2.61288516284702,55.3777152681386));
#7955=CARTESIAN_POINT('Ctrl Pts',(3.06359597981802,2.70479208688044,55.383521588678));
#7956=CARTESIAN_POINT('Ctrl Pts',(2.98306839275632,2.79335372204194,55.3893279092173));
#7957=CARTESIAN_POINT('Ctrl Pts',(2.89882172194849,2.87820388860129,55.3951342297567));
#7958=CARTESIAN_POINT('Ctrl Pts',(2.81456728794737,2.96306187396508,55.400941085339));
#7959=CARTESIAN_POINT('Ctrl Pts',(2.72659337616108,3.0442074213325,55.4067479409213));
#7960=CARTESIAN_POINT('Ctrl Pts',(2.63526848534855,3.1213114247266,55.4125547965037));
#7961=CARTESIAN_POINT('Ctrl Pts',(2.54391369543131,3.19844067141034,55.4183635532083));
#7962=CARTESIAN_POINT('Ctrl Pts',(2.44920605602495,3.27152547963709,55.4241723099129));
#7963=CARTESIAN_POINT('Ctrl Pts',(2.3515463842728,3.34027762358363,55.4299810666175));
#7964=CARTESIAN_POINT('Ctrl Pts',(2.25377939040739,3.40910532200673,55.4357962067968));
#7965=CARTESIAN_POINT('Ctrl Pts',(2.15305422253278,3.47359061754456,55.4416113469761));
#7966=CARTESIAN_POINT('Ctrl Pts',(2.04979998118545,3.53348907414925,55.4474264871554));
#7967=CARTESIAN_POINT('Ctrl Pts',(1.94647773349962,3.59342698167298,55.4532454573603));
#7968=CARTESIAN_POINT('Ctrl Pts',(1.84062345546751,3.64877184515063,55.4590644275653));
#7969=CARTESIAN_POINT('Ctrl Pts',(1.73268861931165,3.69932631008781,55.4648833977702));
#7970=CARTESIAN_POINT('Ctrl Pts',(1.62460189747605,3.74995191516421,55.4707105564181));
#7971=CARTESIAN_POINT('Ctrl Pts',(1.5144291493792,3.79577351179383,55.4765377150659));
#7972=CARTESIAN_POINT('Ctrl Pts',(1.40263956837634,3.83664270439991,55.4823648737138));
#7973=CARTESIAN_POINT('Ctrl Pts',(1.37821913804122,3.8455705781958,55.4836378163309));
#7974=CARTESIAN_POINT('Ctrl Pts',(1.35372159872691,3.85426231320738,55.4849107589481));
#7975=CARTESIAN_POINT('Ctrl Pts',(1.32915191293776,3.86271668548625,55.4861837015652));
#7976=CARTESIAN_POINT('Ctrl Pts',(1.21668908557449,3.9014148853014,55.4920103420451));
#7977=CARTESIAN_POINT('Ctrl Pts',(1.10235582985559,3.93525907455255,55.4978369825249));
#7978=CARTESIAN_POINT('Ctrl Pts',(0.986608468599427,3.96406719540523,55.5036636230047));
#7979=CARTESIAN_POINT('Ctrl Pts',(0.871005908623315,3.99283927696742,55.5094829742903));
#7980=CARTESIAN_POINT('Ctrl Pts',(0.753993154183893,4.01658772381757,55.5153023255759));
#7981=CARTESIAN_POINT('Ctrl Pts',(0.636044144039981,4.03517940701928,55.5211216768615));
#7982=CARTESIAN_POINT('Ctrl Pts',(0.518212046349538,4.05375266192477,55.5269352599373));
#7983=CARTESIAN_POINT('Ctrl Pts',(0.399445939794447,4.06717925897552,55.532748843013));
#7984=CARTESIAN_POINT('Ctrl Pts',(0.280231906400479,4.07537667935556,55.5385624260888));
#7985=CARTESIAN_POINT('Ctrl Pts',(0.157302707267462,4.08382956274173,55.5445571826729));
#7986=CARTESIAN_POINT('Ctrl Pts',(0.033897634179829,4.08672190161919,55.5505519392569));
#7987=CARTESIAN_POINT('Ctrl Pts',(-0.0894419552695308,4.08402070717541,
55.556546695841));
#7988=CARTESIAN_POINT('Ctrl Pts',(-0.208921649216648,4.08140404624055,55.5623538473415));
#7989=CARTESIAN_POINT('Ctrl Pts',(-0.32833945943321,4.07353873827955,55.5681609988421));
#7990=CARTESIAN_POINT('Ctrl Pts',(-0.447201890102587,4.06044769323392,55.5739681503426));
#7991=CARTESIAN_POINT('Ctrl Pts',(-0.56604731179769,4.04735852149046,55.5797744708515));
#7992=CARTESIAN_POINT('Ctrl Pts',(-0.684337106748181,4.02904514450999,55.5855807913604));
#7993=CARTESIAN_POINT('Ctrl Pts',(-0.801582788375328,4.00558235883129,55.5913871118693));
#7994=CARTESIAN_POINT('Ctrl Pts',(-0.918839274005289,3.98211741109426,55.5971939674214));
#7995=CARTESIAN_POINT('Ctrl Pts',(-1.0350510551185,3.95350219124539,55.6030008229734));
#7996=CARTESIAN_POINT('Ctrl Pts',(-1.14974035252565,3.91986251312137,55.6088076785255));
#7997=CARTESIAN_POINT('Ctrl Pts',(-1.26446719837932,3.88621182161002,55.6146164352001));
#7998=CARTESIAN_POINT('Ctrl Pts',(-1.37767017808778,3.84753351500041,55.6204251918747));
#7999=CARTESIAN_POINT('Ctrl Pts',(-1.48888778213046,3.80400291432888,55.6262339485492));
#8000=CARTESIAN_POINT('Ctrl Pts',(-1.60022760764993,3.76042447613788,55.632049088699));
#8001=CARTESIAN_POINT('Ctrl Pts',(-1.70957732261405,3.71198324906251,55.6378642288488));
#8002=CARTESIAN_POINT('Ctrl Pts',(-1.81649633988437,3.6589023008529,55.6436793689986));
#8003=CARTESIAN_POINT('Ctrl Pts',(-1.9234857772298,3.60578639193701,55.6494983391743));
#8004=CARTESIAN_POINT('Ctrl Pts',(-2.02804097239212,3.54802487264844,55.65531730935));
#8005=CARTESIAN_POINT('Ctrl Pts',(-2.12974826733999,3.48588544243243,55.6611362795257));
#8006=CARTESIAN_POINT('Ctrl Pts',(-2.23159868459564,3.42365856973098,55.666963438145));
#8007=CARTESIAN_POINT('Ctrl Pts',(-2.33059286620757,3.35704171751783,55.6727905967642));
#8008=CARTESIAN_POINT('Ctrl Pts',(-2.42634821453776,3.28634437358738,55.6786177553834));
#8009=CARTESIAN_POINT('Ctrl Pts',(-2.44726597214082,3.2709005375061,55.6798906982909));
#8010=CARTESIAN_POINT('Ctrl Pts',(-2.46802930543698,3.25526212365175,55.6811636411984));
#8011=CARTESIAN_POINT('Ctrl Pts',(-2.48863445605986,3.23943259601302,55.6824365841059));
#8012=CARTESIAN_POINT('Ctrl Pts',(-2.58202114796586,3.16768998914392,55.6882058176967));
#8013=CARTESIAN_POINT('Ctrl Pts',(-2.67246630657159,3.09178020599366,55.6939750512874));
#8014=CARTESIAN_POINT('Ctrl Pts',(-2.75957065685742,3.01197523061056,55.6997442848782));
#8015=CARTESIAN_POINT('Ctrl Pts',(-2.84656550524162,2.93227058083157,55.7055062657651));
#8016=CARTESIAN_POINT('Ctrl Pts',(-2.93022759101167,2.84868075368061,55.7112682466521));
#8017=CARTESIAN_POINT('Ctrl Pts',(-3.01018835185631,2.76151970594971,55.7170302275391));
#8018=CARTESIAN_POINT('Ctrl Pts',(-3.09007044606037,2.67444440861365,55.7227865396997));
#8019=CARTESIAN_POINT('Ctrl Pts',(-3.16625817678164,2.58380518314649,55.7285428518602));
#8020=CARTESIAN_POINT('Ctrl Pts',(-3.23841823802157,2.48995427983112,55.7342991640208));
#8021=CARTESIAN_POINT('Ctrl Pts',(-3.31052828810567,2.39616842069765,55.7400514867193));
#8022=CARTESIAN_POINT('Ctrl Pts',(-3.37861596748438,2.29917564034009,55.7458038094178));
#8023=CARTESIAN_POINT('Ctrl Pts',(-3.44238730437894,2.19936232727822,55.7515561321163));
#8024=CARTESIAN_POINT('Ctrl Pts',(-3.50613594230349,2.0995845420806,55.757306407315));
#8025=CARTESIAN_POINT('Ctrl Pts',(-3.56557106751066,1.99698857059399,55.7630566825137));
#8026=CARTESIAN_POINT('Ctrl Pts',(-3.62044158917792,1.89199040678087,55.7688069577124));
#8027=CARTESIAN_POINT('Ctrl Pts',(-3.67530614804565,1.78700365315637,55.7745566080266));
#8028=CARTESIAN_POINT('Ctrl Pts',(-3.72560689704342,1.67961559585343,55.7803062583408));
#8029=CARTESIAN_POINT('Ctrl Pts',(-3.7711387042501,1.57026681596055,55.786055908655));
#8030=CARTESIAN_POINT('Ctrl Pts',(-3.81667682252701,1.46090287945799,55.7918063559164));
#8031=CARTESIAN_POINT('Ctrl Pts',(-3.85744452577761,1.34957806530178,55.7975568031778));
#8032=CARTESIAN_POINT('Ctrl Pts',(-3.89328511616352,1.23675220002213,55.8033072504393));
#8033=CARTESIAN_POINT('Ctrl Pts',(-3.92915895699138,1.12382166264189,55.8090630325713));
#8034=CARTESIAN_POINT('Ctrl Pts',(-3.96009643240574,1.00938769160976,55.8148188147034));
#8035=CARTESIAN_POINT('Ctrl Pts',(-3.98599095802731,0.893924539614254,55.8205745968354));
#8036=CARTESIAN_POINT('Ctrl Pts',(-4.01189878447341,0.77840207951838,55.8263333354475));
#8037=CARTESIAN_POINT('Ctrl Pts',(-4.03275842980724,0.661849795739136,55.8320920740596));
#8038=CARTESIAN_POINT('Ctrl Pts',(-4.04851488777089,0.544749670488611,55.8378508126716));
#8039=CARTESIAN_POINT('Ctrl Pts',(-4.06429355947626,0.427484455346497,55.8436176700584));
#8040=CARTESIAN_POINT('Ctrl Pts',(-4.07495464172175,0.309670271146827,55.8493845274452));
#8041=CARTESIAN_POINT('Ctrl Pts',(-4.08049517445832,0.191791895611725,55.855151384832));
#8042=CARTESIAN_POINT('Ctrl Pts',(-4.08352591976477,0.127310851934067,55.8583059327408));
#8043=CARTESIAN_POINT('Ctrl Pts',(-4.08502539061802,0.0628105767807092,
55.8614604806496));
#8044=CARTESIAN_POINT('Ctrl Pts',(-4.08499967473006,-0.00163017032923469,
55.8646150285584));
#8045=CARTESIAN_POINT('Ctrl Pts',(-4.08499967472976,-0.00163017108645733,
55.8646150285955));
#8046=CARTESIAN_POINT('Ctrl Pts',(-4.0849614297524,-0.0974671794700561,
55.8693065079458));
#8047=CARTESIAN_POINT('Ctrl Pts',(-4.0815508193244,-0.193231850126992,55.8739979872961));
#8048=CARTESIAN_POINT('Ctrl Pts',(-4.07478160324302,-0.288755754699795,
55.8786894666465));
#8049=CARTESIAN_POINT('Ctrl Pts',(-4.06637398885077,-0.407399944105821,
55.884516455892));
#8050=CARTESIAN_POINT('Ctrl Pts',(-4.05276690521363,-0.525865457260426,
55.8903434451375));
#8051=CARTESIAN_POINT('Ctrl Pts',(-4.03397142744041,-0.64366103081852,55.896170434383));
#8052=CARTESIAN_POINT('Ctrl Pts',(-4.01519973360685,-0.761307544967347,
55.9019900501123));
#8053=CARTESIAN_POINT('Ctrl Pts',(-3.99125276903905,-0.878285406458357,
55.9078096658415));
#8054=CARTESIAN_POINT('Ctrl Pts',(-3.96219353843484,-0.994106314226605,
55.9136292815708));
#8055=CARTESIAN_POINT('Ctrl Pts',(-3.93230866040702,-1.11321799164401,55.9196142475393));
#8056=CARTESIAN_POINT('Ctrl Pts',(-3.89701666828244,-1.23110555139611,55.9255992135079));
#8057=CARTESIAN_POINT('Ctrl Pts',(-3.85644311636423,-1.34724589078867,55.9315841794764));
#8058=CARTESIAN_POINT('Ctrl Pts',(-3.81706128616502,-1.45997496943716,55.9373933557101));
#8059=CARTESIAN_POINT('Ctrl Pts',(-3.77270395398662,-1.57105761236674,55.9432025319438));
#8060=CARTESIAN_POINT('Ctrl Pts',(-3.7235369860474,-1.68002896211257,55.9490117081776));
#8061=CARTESIAN_POINT('Ctrl Pts',(-3.67438965859307,-1.78895678161364,55.9548185638485));
#8062=CARTESIAN_POINT('Ctrl Pts',(-3.620436684292,-1.89577461433207,55.9606254195194));
#8063=CARTESIAN_POINT('Ctrl Pts',(-3.56189215523888,-2.00003731826376,55.9664322751903));
#8064=CARTESIAN_POINT('Ctrl Pts',(-3.50335724029384,-2.10428290030686,55.9722381772667));
#8065=CARTESIAN_POINT('Ctrl Pts',(-3.44023247092876,-2.20597383334425,55.9780440793431));
#8066=CARTESIAN_POINT('Ctrl Pts',(-3.37277770636757,-2.30468990179372,55.9838499814196));
#8067=CARTESIAN_POINT('Ctrl Pts',(-3.30531815114227,-2.40341298109748,55.9896562958335));
#8068=CARTESIAN_POINT('Ctrl Pts',(-3.2335282204974,-2.4991604400003,55.9954626102474));
#8069=CARTESIAN_POINT('Ctrl Pts',(-3.15771050668699,-2.59154188774919,56.0012689246613));
#8070=CARTESIAN_POINT('Ctrl Pts',(-3.08183801886284,-2.68399007587354,56.0070794338093));
#8071=CARTESIAN_POINT('Ctrl Pts',(-3.00193219750778,-2.77306708261564,56.0128899429572));
#8072=CARTESIAN_POINT('Ctrl Pts',(-2.91833523262634,-2.85841642697697,56.0187004521052));
#8073=CARTESIAN_POINT('Ctrl Pts',(-2.83470157435502,-2.94380323390375,56.024513511672));
#8074=CARTESIAN_POINT('Ctrl Pts',(-2.74737384114757,-3.02545883912275,56.0303265712389));
#8075=CARTESIAN_POINT('Ctrl Pts',(-2.65672926697682,-3.10306535573919,56.0361396308057));
#8076=CARTESIAN_POINT('Ctrl Pts',(-2.56598553605099,-3.18075676668529,56.0419590493204));
#8077=CARTESIAN_POINT('Ctrl Pts',(-2.47191804151851,-3.25438999591718,56.0477784678351));
#8078=CARTESIAN_POINT('Ctrl Pts',(-2.37493505628005,-3.32368898642037,56.0535978863499));
#8079=CARTESIAN_POINT('Ctrl Pts',(-2.35454449341646,-3.3382590207286,56.0548214125051));
#8080=CARTESIAN_POINT('Ctrl Pts',(-2.33402514682412,-3.35263761934235,56.0560449386604));
#8081=CARTESIAN_POINT('Ctrl Pts',(-2.31338095599003,-3.36682247118297,56.0572684648156));
#8082=CARTESIAN_POINT('',(-4.08499907904467,0.00274302828863158,55.7603849713635));
#8083=CARTESIAN_POINT('Ctrl Pts',(-4.08499907904524,0.00274302744451809,
55.7603849714045));
#8084=CARTESIAN_POINT('Ctrl Pts',(-4.08507962007017,-0.117201092451769,
55.7662069774139));
#8085=CARTESIAN_POINT('Ctrl Pts',(-4.07987312568528,-0.237187977077858,
55.7720289834232));
#8086=CARTESIAN_POINT('Ctrl Pts',(-4.06939496226397,-0.356720676581326,
55.7778509894326));
#8087=CARTESIAN_POINT('Ctrl Pts',(-4.05891733800245,-0.476247225462436,
55.7836726958673));
#8088=CARTESIAN_POINT('Ctrl Pts',(-4.0431686192454,-0.595319232855506,55.7894944023021));
#8089=CARTESIAN_POINT('Ctrl Pts',(-4.02221613371006,-0.713444022837443,
55.7953161087369));
#8090=CARTESIAN_POINT('Ctrl Pts',(-4.00125990646559,-0.831589907624846,
55.8011388548159));
#8091=CARTESIAN_POINT('Ctrl Pts',(-3.97509813425175,-0.94878784029879,55.806961600895));
#8092=CARTESIAN_POINT('Ctrl Pts',(-3.94384932198535,-1.06455508334501,55.812784346974));
#8093=CARTESIAN_POINT('Ctrl Pts',(-3.9125877409405,-1.18036963079005,55.8186094723229));
#8094=CARTESIAN_POINT('Ctrl Pts',(-3.87623508960262,-1.29475193540395,55.8244345976717));
#8095=CARTESIAN_POINT('Ctrl Pts',(-3.83495963376548,-1.40723473784202,55.8302597230206));
#8096=CARTESIAN_POINT('Ctrl Pts',(-3.79363389169115,-1.51985457903035,55.8360919451689));
#8097=CARTESIAN_POINT('Ctrl Pts',(-3.74737351197248,-1.63056991855327,55.8419241673173));
#8098=CARTESIAN_POINT('Ctrl Pts',(-3.69639488000267,-1.73893354993515,55.8477563894657));
#8099=CARTESIAN_POINT('Ctrl Pts',(-3.64537959984465,-1.84737508318697,55.8535928043584));
#8100=CARTESIAN_POINT('Ctrl Pts',(-3.58963949908449,-1.9534611839262,55.8594292192512));
#8101=CARTESIAN_POINT('Ctrl Pts',(-3.52943605806971,-2.05677079714716,55.865265634144));
#8102=CARTESIAN_POINT('Ctrl Pts',(-3.46914148721096,-2.16023678995,55.8711108836079));
#8103=CARTESIAN_POINT('Ctrl Pts',(-3.40437030766645,-2.2609175670037,55.8769561330717));
#8104=CARTESIAN_POINT('Ctrl Pts',(-3.33542639573551,-2.35842230286071,55.8828013825356));
#8105=CARTESIAN_POINT('Ctrl Pts',(-3.31661322220324,-2.38502905412446,55.8843964137635));
#8106=CARTESIAN_POINT('Ctrl Pts',(-3.29748956415988,-2.41139951163461,55.8859914449914));
#8107=CARTESIAN_POINT('Ctrl Pts',(-3.27806208721923,-2.43752619521019,55.8875864762193));
#8108=CARTESIAN_POINT('Ctrl Pts',(-3.20710690365541,-2.53294896342057,55.893412025976));
#8109=CARTESIAN_POINT('Ctrl Pts',(-3.13186879950885,-2.62542279303147,55.8992375757327));
#8110=CARTESIAN_POINT('Ctrl Pts',(-3.05262143677735,-2.71453999118218,55.9050631254894));
#8111=CARTESIAN_POINT('Ctrl Pts',(-2.97346095662305,-2.80355948599514,55.9108822884244));
#8112=CARTESIAN_POINT('Ctrl Pts',(-2.89030022290519,-2.88922936187276,55.9167014513595));
#8113=CARTESIAN_POINT('Ctrl Pts',(-2.80345518295529,-2.97117216552005,55.9225206142945));
#8114=CARTESIAN_POINT('Ctrl Pts',(-2.71670129106433,-3.05302896624189,55.9283336697373));
#8115=CARTESIAN_POINT('Ctrl Pts',(-2.6262710829065,-3.13116620091211,55.9341467251801));
#8116=CARTESIAN_POINT('Ctrl Pts',(-2.53251903752131,-3.20524138320223,55.9399597806229));
#8117=CARTESIAN_POINT('Ctrl Pts',(-2.46133111986253,-3.26148824113224,55.9443737569847));
#8118=CARTESIAN_POINT('Ctrl Pts',(-2.38822877536372,-3.31539370669703,55.9487877333466));
#8119=CARTESIAN_POINT('Ctrl Pts',(-2.31338095599003,-3.36682247118298,55.9532017097085));
#8120=CARTESIAN_POINT('Ctrl Pts',(-2.31338095599002,-3.36682247118298,54.7030792959875));
#8121=CARTESIAN_POINT('Ctrl Pts',(-2.27413470222594,-3.39378900619601,54.7054092576502));
#8122=CARTESIAN_POINT('Ctrl Pts',(-2.23443999392367,-3.42005333803004,54.7077392193128));
#8123=CARTESIAN_POINT('Ctrl Pts',(-2.19432454529482,-3.44560078794928,54.7100691809754));
#8124=CARTESIAN_POINT('Ctrl Pts',(-2.09400602881825,-3.50948845126245,54.7158958214701));
#8125=CARTESIAN_POINT('Ctrl Pts',(-1.99073541405492,-3.5690930039375,54.7217224619647));
#8126=CARTESIAN_POINT('Ctrl Pts',(-1.88491390154344,-3.62413087288087,54.7275491024594));
#8127=CARTESIAN_POINT('Ctrl Pts',(-1.77922477296197,-3.67909988881679,54.7333684537597));
#8128=CARTESIAN_POINT('Ctrl Pts',(-1.67099145276118,-3.72951339782278,54.73918780506));
#8129=CARTESIAN_POINT('Ctrl Pts',(-1.56064369498213,-3.77513129007622,54.7450071563604));
#8130=CARTESIAN_POINT('Ctrl Pts',(-1.4504053152065,-3.82070396533499,54.7508207394508));
#8131=CARTESIAN_POINT('Ctrl Pts',(-1.3380570422053,-3.86149032568069,54.7566343225413));
#8132=CARTESIAN_POINT('Ctrl Pts',(-1.22405225467107,-3.8972966371364,54.7624479056317));
#8133=CARTESIAN_POINT('Ctrl Pts',(-1.10649464184963,-3.93421881022855,54.7684426622102));
#8134=CARTESIAN_POINT('Ctrl Pts',(-0.987175968270247,-3.96584525144488,
54.7744374187888));
#8135=CARTESIAN_POINT('Ctrl Pts',(-0.866614925145773,-3.99201748136385,
54.7804321753673));
#8136=CARTESIAN_POINT('Ctrl Pts',(-0.749826822901344,-4.01737065503029,
54.7862393268822));
#8137=CARTESIAN_POINT('Ctrl Pts',(-0.631873378760497,-4.03760581114111,
54.7920464783971));
#8138=CARTESIAN_POINT('Ctrl Pts',(-0.513239797011675,-4.05262999924289,
54.7978536299121));
#8139=CARTESIAN_POINT('Ctrl Pts',(-0.394623191492106,-4.06765203741327,
54.8036599504352));
#8140=CARTESIAN_POINT('Ctrl Pts',(-0.275327046402772,-4.07746453936188,
54.8094662709583));
#8141=CARTESIAN_POINT('Ctrl Pts',(-0.155843810341062,-4.08202617664051,
54.8152725914814));
#8142=CARTESIAN_POINT('Ctrl Pts',(-0.0363495640925718,-4.08658823426664,
54.8210794470476));
#8143=CARTESIAN_POINT('Ctrl Pts',(0.0833313998760015,-4.08589844963655,
54.8268863026137));
#8144=CARTESIAN_POINT('Ctrl Pts',(0.202705132280273,-4.07996760150706,54.8326931581799));
#8145=CARTESIAN_POINT('Ctrl Pts',(0.322117946777565,-4.07403481166096,54.8385019148684));
#8146=CARTESIAN_POINT('Ctrl Pts',(0.441222922575412,-4.06285756596303,54.8443106715569));
#8147=CARTESIAN_POINT('Ctrl Pts',(0.559530370828998,-4.04649858076337,54.8501194282454));
#8148=CARTESIAN_POINT('Ctrl Pts',(0.677967831866507,-4.03012161802096,54.8559345684088));
#8149=CARTESIAN_POINT('Ctrl Pts',(0.795605611801294,-4.00855160548719,54.8617497085722));
#8150=CARTESIAN_POINT('Ctrl Pts',(0.911963217393696,-3.98190257165101,54.8675648487356));
#8151=CARTESIAN_POINT('Ctrl Pts',(1.02839745959529,-3.95523598596181,54.8733838189247));
#8152=CARTESIAN_POINT('Ctrl Pts',(1.14354945602695,-3.92348382490905,54.8792027891139));
#8153=CARTESIAN_POINT('Ctrl Pts',(1.25695447707683,-3.88680980272466,54.885021759303));
#8154=CARTESIAN_POINT('Ctrl Pts',(1.37051908144492,-3.85008417292979,54.8908489179353));
#8155=CARTESIAN_POINT('Ctrl Pts',(1.48233142331655,-3.8084230007567,54.8966760765677));
#8156=CARTESIAN_POINT('Ctrl Pts',(1.59194721769772,-3.76203788604853,54.9025032352));
#8157=CARTESIAN_POINT('Ctrl Pts',(1.61589278739337,-3.75190505798889,54.903776177972));
#8158=CARTESIAN_POINT('Ctrl Pts',(1.63973363355421,-3.74154697378309,54.9050491207441));
#8159=CARTESIAN_POINT('Ctrl Pts',(1.66346529288866,-3.73096612412319,54.9063220635161));
#8160=CARTESIAN_POINT('Ctrl Pts',(1.77209220868144,-3.68253440475525,54.9121487040117));
#8161=CARTESIAN_POINT('Ctrl Pts',(1.87877511718031,-3.62927767174078,54.9179753445073));
#8162=CARTESIAN_POINT('Ctrl Pts',(1.98305617814506,-3.57137413250428,54.923801985003));
#8163=CARTESIAN_POINT('Ctrl Pts',(2.0872067823021,-3.51354303126193,54.9296213363042));
#8164=CARTESIAN_POINT('Ctrl Pts',(2.18896116201644,-3.45107688279009,54.9354406876055));
#8165=CARTESIAN_POINT('Ctrl Pts',(2.28788197809559,-3.38420168641076,54.9412600389068));
#8166=CARTESIAN_POINT('Ctrl Pts',(2.38670474269078,-3.31739277751777,54.9470736219982));
#8167=CARTESIAN_POINT('Ctrl Pts',(2.48269919537037,-3.24618374230914,54.9528872050896));
#8168=CARTESIAN_POINT('Ctrl Pts',(2.57545364624933,-3.17084586759133,54.958700788181));
#8169=CARTESIAN_POINT('Ctrl Pts',(2.67109868061442,-3.09316017652104,54.9646955447591));
#8170=CARTESIAN_POINT('Ctrl Pts',(2.7632980775166,-3.01108430395582,54.9706903013373));
#8171=CARTESIAN_POINT('Ctrl Pts',(2.85163352382441,-2.92496346059242,54.9766850579154));
#8172=CARTESIAN_POINT('Ctrl Pts',(2.93720452478794,-2.84153775688623,54.9824922094312));
#8173=CARTESIAN_POINT('Ctrl Pts',(3.01914949873876,-2.75431678592284,54.988299360947));
#8174=CARTESIAN_POINT('Ctrl Pts',(3.09712326188684,-2.66365397540285,54.9941065124628));
#8175=CARTESIAN_POINT('Ctrl Pts',(3.1750858671444,-2.57300413855084,54.9999128329868));
#8176=CARTESIAN_POINT('Ctrl Pts',(3.24907812593549,-2.47891375078002,55.0057191535108));
#8177=CARTESIAN_POINT('Ctrl Pts',(3.31879391547839,-2.38177075861294,55.0115254740347));
#8178=CARTESIAN_POINT('Ctrl Pts',(3.38851612921808,-2.28461881487686,55.0173323296017));
#8179=CARTESIAN_POINT('Ctrl Pts',(3.45396085241963,-2.1844140387996,55.0231391851687));
#8180=CARTESIAN_POINT('Ctrl Pts',(3.51486459638405,-2.0815743727011,55.0289460407357));
#8181=CARTESIAN_POINT('Ctrl Pts',(3.57578827979171,-1.97870103764317,55.034754797425));
#8182=CARTESIAN_POINT('Ctrl Pts',(3.6321678195309,-1.87319144763098,55.0405635541142));
#8183=CARTESIAN_POINT('Ctrl Pts',(3.68378539754664,-1.76548864194085,55.0463723108035));
#8184=CARTESIAN_POINT('Ctrl Pts',(3.73545970018174,-1.65766747733323,55.0521874509677));
#8185=CARTESIAN_POINT('Ctrl Pts',(3.78236141935878,-1.5476486541637,55.0580025911319));
#8186=CARTESIAN_POINT('Ctrl Pts',(3.82432060838779,-1.43589584728854,55.063817731296));
#8187=CARTESIAN_POINT('Ctrl Pts',(3.86630743299707,-1.32406943666324,55.0696367014859));
#8188=CARTESIAN_POINT('Ctrl Pts',(3.90334511813548,-1.21050715464037,55.0754556716758));
#8189=CARTESIAN_POINT('Ctrl Pts',(3.93531385506652,-1.09568693618272,55.0812746418656));
#8190=CARTESIAN_POINT('Ctrl Pts',(3.96732757833984,-0.980705142944693,55.0871018004987));
#8191=CARTESIAN_POINT('Ctrl Pts',(3.99425802551269,-0.864462276144644,55.0929289591317));
#8192=CARTESIAN_POINT('Ctrl Pts',(4.01603660652882,-0.747445633488134,55.0987561177647));
#8193=CARTESIAN_POINT('Ctrl Pts',(4.02079413740465,-0.721883348690442,55.1000290605287));
#8194=CARTESIAN_POINT('Ctrl Pts',(4.02530601614962,-0.696284153471523,55.1013020032927));
#8195=CARTESIAN_POINT('Ctrl Pts',(4.02957185811376,-0.67065314455208,55.1025749460567));
#8196=CARTESIAN_POINT('Ctrl Pts',(4.04909789515259,-0.553332335738597,55.1084015865575));
#8197=CARTESIAN_POINT('Ctrl Pts',(4.06352707368852,-0.434971356480761,55.1142282270584));
#8198=CARTESIAN_POINT('Ctrl Pts',(4.07275547397121,-0.316050390345526,55.1200548675592));
#8199=CARTESIAN_POINT('Ctrl Pts',(4.08197232941901,-0.197278195706544,55.1258742188658));
#8200=CARTESIAN_POINT('Ctrl Pts',(4.08600131651674,-0.0779478107034862,
55.1316935701723));
#8201=CARTESIAN_POINT('Ctrl Pts',(4.08478968715762,0.0414513171170837,55.1375129214789));
#8202=CARTESIAN_POINT('Ctrl Pts',(4.08357925877985,0.160732095109789,55.1433265045756));
#8203=CARTESIAN_POINT('Ctrl Pts',(4.07713855234978,0.280081074856549,55.1491400876723));
#8204=CARTESIAN_POINT('Ctrl Pts',(4.06546674246128,0.399005220443617,55.154953670769));
#8205=CARTESIAN_POINT('Ctrl Pts',(4.05343119434556,0.521635497153633,55.1609484273451));
#8206=CARTESIAN_POINT('Ctrl Pts',(4.03583312540292,0.643813586859018,55.1669431839213));
#8207=CARTESIAN_POINT('Ctrl Pts',(4.01272971553403,0.765000150372641,55.1729379404975));
#8208=CARTESIAN_POINT('Ctrl Pts',(3.99034932359311,0.882394197606358,55.1787450920187));
#8209=CARTESIAN_POINT('Ctrl Pts',(3.96280311173274,0.998857422566529,55.18455224354));
#8210=CARTESIAN_POINT('Ctrl Pts',(3.93019545416052,1.11390694947826,55.1903593950612));
#8211=CARTESIAN_POINT('Ctrl Pts',(3.89759246267913,1.22894001303194,55.1961657155906));
#8212=CARTESIAN_POINT('Ctrl Pts',(3.85992957711822,1.34255938861216,55.20197203612));
#8213=CARTESIAN_POINT('Ctrl Pts',(3.81736151073809,1.45429573895251,55.2077783566494));
#8214=CARTESIAN_POINT('Ctrl Pts',(3.77478952177962,1.56604238561646,55.2135852122218));
#8215=CARTESIAN_POINT('Ctrl Pts',(3.72731159849809,1.67590528093854,55.2193920677943));
#8216=CARTESIAN_POINT('Ctrl Pts',(3.6751309916417,1.7834341014668,55.2251989233667));
#8217=CARTESIAN_POINT('Ctrl Pts',(3.62293330123368,1.89099812614978,55.2310076800615));
#8218=CARTESIAN_POINT('Ctrl Pts',(3.56603004317143,1.99622618957287,55.2368164367562));
#8219=CARTESIAN_POINT('Ctrl Pts',(3.50467059470403,2.09869221721931,55.242625193451));
#8220=CARTESIAN_POINT('Ctrl Pts',(3.4432437158866,2.20127084887839,55.2484403336206));
#8221=CARTESIAN_POINT('Ctrl Pts',(3.37735108160713,2.30108103616106,55.2542554737903));
#8222=CARTESIAN_POINT('Ctrl Pts',(3.30728568843415,2.39772525012327,55.2600706139599));
#8223=CARTESIAN_POINT('Ctrl Pts',(3.23717414809192,2.49443311686321,55.2658895841552));
#8224=CARTESIAN_POINT('Ctrl Pts',(3.16288462843217,2.58797053885086,55.2717085543506));
#8225=CARTESIAN_POINT('Ctrl Pts',(3.08474967797375,2.67797394017209,55.2775275245459));
#8226=CARTESIAN_POINT('Ctrl Pts',(3.00650477617087,2.76810399409786,55.2833546831844));
#8227=CARTESIAN_POINT('Ctrl Pts',(2.9244039231842,2.85468980720146,55.2891818418228));
#8228=CARTESIAN_POINT('Ctrl Pts',(2.83881573082375,2.9374053595695,55.2950090004613));
#8229=CARTESIAN_POINT('Ctrl Pts',(2.82011899156167,2.95547457067085,55.2962819431733));
#8230=CARTESIAN_POINT('Ctrl Pts',(2.80125595581707,2.97335924771464,55.2975548858854));
#8231=CARTESIAN_POINT('Ctrl Pts',(2.78223066250909,2.99105625834658,55.2988278285974));
#8232=CARTESIAN_POINT('Ctrl Pts',(2.69514619014679,3.07206078260409,55.3046544690928));
#8233=CARTESIAN_POINT('Ctrl Pts',(2.6043825263909,3.14938787953511,55.3104811095882));
#8234=CARTESIAN_POINT('Ctrl Pts',(2.51028286019059,3.22268598560787,55.3163077500836));
#8235=CARTESIAN_POINT('Ctrl Pts',(2.41630091375526,3.29589239490668,55.3221271013848));
#8236=CARTESIAN_POINT('Ctrl Pts',(2.31899158486167,3.3650795903048,55.3279464526859));
#8237=CARTESIAN_POINT('Ctrl Pts',(2.21873401742616,3.42993357951958,55.333765803987));
#8238=CARTESIAN_POINT('Ctrl Pts',(2.11857582647777,3.49472328469287,55.3395793870783));
#8239=CARTESIAN_POINT('Ctrl Pts',(2.01547555129439,3.55518810833686,55.3453929701695));
#8240=CARTESIAN_POINT('Ctrl Pts',(1.90984397111666,3.61105538672413,55.3512065532608));
#8241=CARTESIAN_POINT('Ctrl Pts',(1.80092050684368,3.66866370320681,55.357201309839));
#8242=CARTESIAN_POINT('Ctrl Pts',(1.68930573118877,3.7213829549389,55.3631960664172));
#8243=CARTESIAN_POINT('Ctrl Pts',(1.57548104201319,3.76896331718114,55.3691908229954));
#8244=CARTESIAN_POINT('Ctrl Pts',(1.46521848044732,3.81505465869113,55.3749979745112));
#8245=CARTESIAN_POINT('Ctrl Pts',(1.3528826643103,3.8563237869193,55.3808051260269));
#8246=CARTESIAN_POINT('Ctrl Pts',(1.2389339300701,3.89259138838397,55.3866122775427));
#8247=CARTESIAN_POINT('Ctrl Pts',(1.12500150166655,3.92885380002719,55.3924185980667));
#8248=CARTESIAN_POINT('Ctrl Pts',(1.00945700268923,3.96011598466009,55.3982249185907));
#8249=CARTESIAN_POINT('Ctrl Pts',(0.892777246042168,3.98624808422022,55.4040312391146));
#8250=CARTESIAN_POINT('Ctrl Pts',(0.776086737544239,4.01238259181106,55.4098380946817));
#8251=CARTESIAN_POINT('Ctrl Pts',(0.658261161350215,4.03338598529941,55.4156449502487));
#8252=CARTESIAN_POINT('Ctrl Pts',(0.539788246117744,4.04917937974513,55.4214518058157));
#8253=CARTESIAN_POINT('Ctrl Pts',(0.421276543713065,4.06497794483351,55.427260562505));
#8254=CARTESIAN_POINT('Ctrl Pts',(0.302117484790072,4.07556306466938,55.4330693191944));
#8255=CARTESIAN_POINT('Ctrl Pts',(0.182804017234988,4.08090770433279,55.4388780758838));
#8256=CARTESIAN_POINT('Ctrl Pts',(0.0633594313408508,4.08625821743439,55.4446932160481));
#8257=CARTESIAN_POINT('Ctrl Pts',(-0.0562394942678495,4.08635673707916,
55.4505083562124));
#8258=CARTESIAN_POINT('Ctrl Pts',(-0.175499559289298,4.08122835733181,55.4563234963767));
#8259=CARTESIAN_POINT('Ctrl Pts',(-0.294838172566923,4.07609659987972,55.4621424665667));
#8260=CARTESIAN_POINT('Ctrl Pts',(-0.413837075458972,4.06573112215777,55.4679614367567));
#8261=CARTESIAN_POINT('Ctrl Pts',(-0.53200956923297,4.05020873761397,55.4737804069468));
#8262=CARTESIAN_POINT('Ctrl Pts',(-0.650348355103284,4.03466451000176,55.47960756558));
#8263=CARTESIAN_POINT('Ctrl Pts',(-0.767858010762216,4.01394896287395,55.4854347242132));
#8264=CARTESIAN_POINT('Ctrl Pts',(-0.884063268697977,3.98818970673902,55.4912618828465));
#8265=CARTESIAN_POINT('Ctrl Pts',(-0.909448306504777,3.9825625974113,55.4925348256103));
#8266=CARTESIAN_POINT('Ctrl Pts',(-0.934771161712084,3.97669498720446,55.4938077683742));
#8267=CARTESIAN_POINT('Ctrl Pts',(-0.96002699366087,3.97058851701388,55.495080711138));
#8268=CARTESIAN_POINT('Ctrl Pts',(-1.07563050494179,3.94263737301693,55.5009073516327));
#8269=CARTESIAN_POINT('Ctrl Pts',(-1.19019629028253,3.90958887226335,55.5067339921275));
#8270=CARTESIAN_POINT('Ctrl Pts',(-1.30324180069416,3.87153532967522,55.5125606326222));
#8271=CARTESIAN_POINT('Ctrl Pts',(-1.416145889871,3.83352939250691,55.5183799839226));
#8272=CARTESIAN_POINT('Ctrl Pts',(-1.52753310387075,3.79053099661766,55.524199335223));
#8273=CARTESIAN_POINT('Ctrl Pts',(-1.63693239739873,3.74268317205003,55.5300186865233));
#8274=CARTESIAN_POINT('Ctrl Pts',(-1.74622325305185,3.69488277481255,55.5358322696138));
#8275=CARTESIAN_POINT('Ctrl Pts',(-1.85352973679054,3.64224267428103,55.5416458527043));
#8276=CARTESIAN_POINT('Ctrl Pts',(-1.95839782379331,3.58495508531999,55.5474594357948));
#8277=CARTESIAN_POINT('Ctrl Pts',(-2.06653400154259,3.52588219594273,55.5534541923733));
#8278=CARTESIAN_POINT('Ctrl Pts',(-2.17207689503155,3.46186754697634,55.5594489489518));
#8279=CARTESIAN_POINT('Ctrl Pts',(-2.27455257351142,3.39317485407584,55.5654437055303));
#8280=CARTESIAN_POINT('Ctrl Pts',(-2.37382129005347,3.32663188933334,55.5712508570452));
#8281=CARTESIAN_POINT('Ctrl Pts',(-2.47021154122054,3.25569955532869,55.5770580085602));
#8282=CARTESIAN_POINT('Ctrl Pts',(-2.56331982692313,3.18066289708651,55.5828651600751));
#8283=CARTESIAN_POINT('Ctrl Pts',(-2.65641478901527,3.10563697644085,55.5886714805982));
#8284=CARTESIAN_POINT('Ctrl Pts',(-2.74622840222356,3.02650815545822,55.5944778011213));
#8285=CARTESIAN_POINT('Ctrl Pts',(-2.83238932759356,2.94360250321508,55.6002841216444));
#8286=CARTESIAN_POINT('Ctrl Pts',(-2.91855819255312,2.86068921135052,55.6060909772106));
#8287=CARTESIAN_POINT('Ctrl Pts',(-3.00107340657881,2.77399867903235,55.6118978327767));
#8288=CARTESIAN_POINT('Ctrl Pts',(-3.07960012520711,2.68389419851535,55.6177046883428));
#8289=CARTESIAN_POINT('Ctrl Pts',(-3.15815255291268,2.59376021844594,55.6235134450313));
#8290=CARTESIAN_POINT('Ctrl Pts',(-3.23271362042647,2.5002103745522,55.6293222017198));
#8291=CARTESIAN_POINT('Ctrl Pts',(-3.30298885158018,2.40364091459956,55.6351309584082));
#8292=CARTESIAN_POINT('Ctrl Pts',(-3.37334131099423,2.30696533060761,55.6409460985716));
#8293=CARTESIAN_POINT('Ctrl Pts',(-3.43939829295682,2.20726383692335,55.646761238735));
#8294=CARTESIAN_POINT('Ctrl Pts',(-3.50090866213717,2.10496164795773,55.6525763788983));
#8295=CARTESIAN_POINT('Ctrl Pts',(-3.56245954389156,2.00259207970209,55.6583953490874));
#8296=CARTESIAN_POINT('Ctrl Pts',(-3.61945765488474,1.89761876234378,55.6642143192765));
#8297=CARTESIAN_POINT('Ctrl Pts',(-3.67169858470686,1.79049001758224,55.6700332894656));
#8298=CARTESIAN_POINT('Ctrl Pts',(-3.72401302786043,1.68321052146639,55.6758604480978));
#8299=CARTESIAN_POINT('Ctrl Pts',(-3.77155676736374,1.57376991704553,55.68168760673));
#8300=CARTESIAN_POINT('Ctrl Pts',(-3.81417406779311,1.4626350127679,55.6875147653623));
#8301=CARTESIAN_POINT('Ctrl Pts',(-3.82348381684447,1.43835759352155,55.6887877081344));
#8302=CARTESIAN_POINT('Ctrl Pts',(-3.8325586653512,1.41399937152597,55.6900606509065));
#8303=CARTESIAN_POINT('Ctrl Pts',(-3.84139731169079,1.38956528948256,55.6913335936786));
#8304=CARTESIAN_POINT('Ctrl Pts',(-3.887911547906,1.26097855569982,55.698032578853));
#8305=CARTESIAN_POINT('Ctrl Pts',(-3.92800186419981,1.12995375257658,55.7047315640274));
#8306=CARTESIAN_POINT('Ctrl Pts',(-3.96144195472371,0.997097106281418,55.7114305492018));
#8307=CARTESIAN_POINT('Ctrl Pts',(-3.99475499066144,0.864745244690844,55.7181040817899));
#8308=CARTESIAN_POINT('Ctrl Pts',(-4.02146813859723,0.73057557588834,55.724777614378));
#8309=CARTESIAN_POINT('Ctrl Pts',(-4.04140466040663,0.595208678400749,55.7314511469661));
#8310=CARTESIAN_POINT('Ctrl Pts',(-4.06120264161761,0.460782457083427,55.7380783046044));
#8311=CARTESIAN_POINT('Ctrl Pts',(-4.07431776582529,0.325175745336553,55.7447054622427));
#8312=CARTESIAN_POINT('Ctrl Pts',(-4.0806247467514,0.189015015805715,55.751332619881));
#8313=CARTESIAN_POINT('Ctrl Pts',(-4.08349641568564,0.127018865565581,55.7543500703752));
#8314=CARTESIAN_POINT('Ctrl Pts',(-4.08495733593587,0.0649081039118598,
55.7573675208694));
#8315=CARTESIAN_POINT('Ctrl Pts',(-4.08499907904467,0.00274302828863158,
55.7603849713635));
#8316=CARTESIAN_POINT('Origin',(0.,0.,46.4896150285955));
#8317=CARTESIAN_POINT('',(-2.31338095599002,-3.36682247118299,53.4530632234442));
#8318=CARTESIAN_POINT('',(-2.31338095599001,-3.36682247118299,53.5574546183695));
#8319=CARTESIAN_POINT('',(-2.31338095599002,-3.36682247118298,46.4896150285955));
#8320=CARTESIAN_POINT('',(-4.08499981754213,-0.00122093438978996,54.6146150286217));
#8321=CARTESIAN_POINT('Ctrl Pts',(-2.31338095599001,-3.36682247118299,53.5574546183695));
#8322=CARTESIAN_POINT('Ctrl Pts',(-2.21507323877183,-3.43437079093728,53.5632685315697));
#8323=CARTESIAN_POINT('Ctrl Pts',(-2.11370279085638,-3.49767973840142,53.5690824447699));
#8324=CARTESIAN_POINT('Ctrl Pts',(-2.00967227144596,-3.55646486857121,53.5748963579702));
#8325=CARTESIAN_POINT('Ctrl Pts',(-1.90155797433677,-3.61755764273785,53.5809384996672));
#8326=CARTESIAN_POINT('Ctrl Pts',(-1.79057083243497,-3.67376387503014,53.5869806413643));
#8327=CARTESIAN_POINT('Ctrl Pts',(-1.67719615426145,-3.72481382892227,53.5930227830613));
#8328=CARTESIAN_POINT('Ctrl Pts',(-1.56822916280103,-3.7738791050442,53.5988300233844));
#8329=CARTESIAN_POINT('Ctrl Pts',(-1.45705721270963,-3.81818134763452,53.6046372637075));
#8330=CARTESIAN_POINT('Ctrl Pts',(-1.34413539373244,-3.85752835936636,53.6104445040305));
#8331=CARTESIAN_POINT('Ctrl Pts',(-1.23123125071837,-3.89686921200216,53.6162508353303));
#8332=CARTESIAN_POINT('Ctrl Pts',(-1.11657816855113,-3.93125624223149,53.6220571666301));
#8333=CARTESIAN_POINT('Ctrl Pts',(-1.00064911336343,-3.96054621888509,53.6278634979298));
#8334=CARTESIAN_POINT('Ctrl Pts',(-0.884710932964752,-3.98983850106266,
53.6336702862677));
#8335=CARTESIAN_POINT('Ctrl Pts',(-0.767496975267442,-4.0140328321037,53.6394770746056));
#8336=CARTESIAN_POINT('Ctrl Pts',(-0.649492567833327,-4.03303662323184,
53.6452838629435));
#8337=CARTESIAN_POINT('Ctrl Pts',(-0.53145111195188,-4.05204638075539,53.65109247437));
#8338=CARTESIAN_POINT('Ctrl Pts',(-0.41261911520761,-4.06586229259228,53.6569010857965));
#8339=CARTESIAN_POINT('Ctrl Pts',(-0.293488597444497,-4.07444345195391,
53.6627096972231));
#8340=CARTESIAN_POINT('Ctrl Pts',(-0.174227900411427,-4.08303398833396,
53.6685246559803));
#8341=CARTESIAN_POINT('Ctrl Pts',(-0.0546684382242412,-4.08637832452129,
53.6743396147375));
#8342=CARTESIAN_POINT('Ctrl Pts',(0.0646960231269892,-4.08448765753938,
53.6801545734947));
#8343=CARTESIAN_POINT('Ctrl Pts',(0.184137663127862,-4.08259576809039,53.6859732920868));
#8344=CARTESIAN_POINT('Ctrl Pts',(0.303383644970468,-4.0754621583867,53.6917920106789));
#8345=CARTESIAN_POINT('Ctrl Pts',(0.421945228617589,-4.06314991405029,53.697610729271));
#8346=CARTESIAN_POINT('Ctrl Pts',(0.540675418571428,-4.05082016048381,53.7034377226569));
#8347=CARTESIAN_POINT('Ctrl Pts',(0.658718865578198,-4.03329713211679,53.7092647160428));
#8348=CARTESIAN_POINT('Ctrl Pts',(0.77559677164338,-4.01069503301066,53.7150917094286));
#8349=CARTESIAN_POINT('Ctrl Pts',(0.80779689710556,-4.00446810397481,53.7166970591855));
#8350=CARTESIAN_POINT('Ctrl Pts',(0.839908645801648,-3.9978559574552,53.7183024089425));
#8351=CARTESIAN_POINT('Ctrl Pts',(0.871922226930701,-3.99086164007025,53.7199077586994));
#8352=CARTESIAN_POINT('Ctrl Pts',(0.988115989079898,-3.96547566255819,53.7257343991827));
#8353=CARTESIAN_POINT('Ctrl Pts',(1.10338508462331,-3.93497061164439,53.731561039666));
#8354=CARTESIAN_POINT('Ctrl Pts',(1.21724503980884,-3.89942810076821,53.7373876801494));
#8355=CARTESIAN_POINT('Ctrl Pts',(1.33096255487992,-3.86393005398222,53.7432070314384));
#8356=CARTESIAN_POINT('Ctrl Pts',(1.44327405004653,-3.82340720250275,53.7490263827274));
#8357=CARTESIAN_POINT('Ctrl Pts',(1.55370543010105,-3.77799211704769,53.7548457340164));
#8358=CARTESIAN_POINT('Ctrl Pts',(1.66402734926497,-3.73262204756271,53.7606593170956));
#8359=CARTESIAN_POINT('Ctrl Pts',(1.77247248578099,-3.68236954563469,53.7664729001747));
#8360=CARTESIAN_POINT('Ctrl Pts',(1.87858267227964,-3.62741673142344,53.7722864832539));
#8361=CARTESIAN_POINT('Ctrl Pts',(1.98799965838778,-3.57075137715763,53.7782812398366));
#8362=CARTESIAN_POINT('Ctrl Pts',(2.0949333571339,-3.50908808380912,53.7842759964194));
#8363=CARTESIAN_POINT('Ctrl Pts',(2.19890411777047,-3.44268001429876,53.7902707530021));
#8364=CARTESIAN_POINT('Ctrl Pts',(2.29962112781829,-3.37835017614829,53.7960779045059));
#8365=CARTESIAN_POINT('Ctrl Pts',(2.3975575147714,-3.30956834288976,53.8018850560097));
#8366=CARTESIAN_POINT('Ctrl Pts',(2.49230356927486,-3.23661056022806,53.8076922075135));
#8367=CARTESIAN_POINT('Ctrl Pts',(2.58703606580779,-3.16366321767886,53.8134985280255));
#8368=CARTESIAN_POINT('Ctrl Pts',(2.67857881480949,-3.08654136292323,53.8193048485376));
#8369=CARTESIAN_POINT('Ctrl Pts',(2.76655335231605,-3.00556276740128,53.8251111690496));
#8370=CARTESIAN_POINT('Ctrl Pts',(2.85453599653532,-2.92457670983146,53.8309180246048));
#8371=CARTESIAN_POINT('Ctrl Pts',(2.93894947545509,-2.83973348108884,53.83672488016));
#8372=CARTESIAN_POINT('Ctrl Pts',(3.01945098691094,-2.75138887430377,53.8425317357151));
#8373=CARTESIAN_POINT('Ctrl Pts',(3.09997885397798,-2.66301534413496,53.8483404923927));
#8374=CARTESIAN_POINT('Ctrl Pts',(3.17659193188125,-2.57113845736897,53.8541492490703));
#8375=CARTESIAN_POINT('Ctrl Pts',(3.24898704755551,-2.47614784793165,53.8599580057479));
#8376=CARTESIAN_POINT('Ctrl Pts',(3.32146172111921,-2.38105284951265,53.8657731459006));
#8377=CARTESIAN_POINT('Ctrl Pts',(3.38970893300221,-2.28283762297132,53.8715882860533));
#8378=CARTESIAN_POINT('Ctrl Pts',(3.45346819932686,-2.18192172092357,53.8774034262061));
#8379=CARTESIAN_POINT('Ctrl Pts',(3.51726945941804,-2.08093935263376,53.8832223963846));
#8380=CARTESIAN_POINT('Ctrl Pts',(3.57657668506128,-1.97725311948707,53.8890413665632));
#8381=CARTESIAN_POINT('Ctrl Pts',(3.63117559448954,-1.87130670975753,53.8948603367418));
#8382=CARTESIAN_POINT('Ctrl Pts',(3.68585133539594,-1.76521121244823,53.9006874953638));
#8383=CARTESIAN_POINT('Ctrl Pts',(3.73580536663856,-1.65684955979108,53.9065146539857));
#8384=CARTESIAN_POINT('Ctrl Pts',(3.78087166040175,-1.54668499946528,53.9123418126077));
#8385=CARTESIAN_POINT('Ctrl Pts',(3.79071639286584,-1.52261954981614,53.9136147554852));
#8386=CARTESIAN_POINT('Ctrl Pts',(3.80032807045,-1.49846811881181,53.9148876983626));
#8387=CARTESIAN_POINT('Ctrl Pts',(3.80970528246749,-1.47423561913939,53.9161606412401));
#8388=CARTESIAN_POINT('Ctrl Pts',(3.85262758802718,-1.3633162164988,53.9219872817217));
#8389=CARTESIAN_POINT('Ctrl Pts',(3.89077006661586,-1.25034421188072,53.9278139222034));
#8390=CARTESIAN_POINT('Ctrl Pts',(3.92393353880419,-1.13576871899502,53.9336405626851));
#8391=CARTESIAN_POINT('Ctrl Pts',(3.95705552310549,-1.02133656137529,53.9394599139721));
#8392=CARTESIAN_POINT('Ctrl Pts',(3.98521077794245,-0.905305293834171,53.9452792652592));
#8393=CARTESIAN_POINT('Ctrl Pts',(4.0082483518158,-0.788143483235101,53.9510986165463));
#8394=CARTESIAN_POINT('Ctrl Pts',(4.03126309057218,-0.671097804814871,53.9569121996232));
#8395=CARTESIAN_POINT('Ctrl Pts',(4.04917016199053,-0.552924210630184,53.9627257827001));
#8396=CARTESIAN_POINT('Ctrl Pts',(4.06186872942208,-0.434105315497335,53.968539365777));
#8397=CARTESIAN_POINT('Ctrl Pts',(4.07496303283255,-0.311583568682053,53.9745341223605));
#8398=CARTESIAN_POINT('Ctrl Pts',(4.08251875788642,-0.188376066085167,53.980528878944));
#8399=CARTESIAN_POINT('Ctrl Pts',(4.0844824727802,-0.0650225311052865,53.9865236355275));
#8400=CARTESIAN_POINT('Ctrl Pts',(4.0863847334865,0.0544706719653243,53.9923307870283));
#8401=CARTESIAN_POINT('Ctrl Pts',(4.08303975986409,0.174100465976518,53.9981379385291));
#8402=CARTESIAN_POINT('Ctrl Pts',(4.07445178836443,0.293372841779753,54.0039450900299));
#8403=CARTESIAN_POINT('Ctrl Pts',(4.06586504578666,0.412628149939694,54.0097514105388));
#8404=CARTESIAN_POINT('Ctrl Pts',(4.05203682673918,0.531525734957949,54.0155577310476));
#8405=CARTESIAN_POINT('Ctrl Pts',(4.03302340655613,0.649574631717078,54.0213640515564));
#8406=CARTESIAN_POINT('Ctrl Pts',(4.01400823431782,0.767634406487022,54.027170907108));
#8407=CARTESIAN_POINT('Ctrl Pts',(3.98980697579756,0.884844934869403,54.0329777626597));
#8408=CARTESIAN_POINT('Ctrl Pts',(3.96052729195874,1.00072402272053,54.0387846182114));
#8409=CARTESIAN_POINT('Ctrl Pts',(3.93123802216488,1.11664104854028,54.0445933748852));
#8410=CARTESIAN_POINT('Ctrl Pts',(3.89686712022224,1.231225371725,54.050402131559));
#8411=CARTESIAN_POINT('Ctrl Pts',(3.85757233399246,1.34400918449836,54.0562108882329));
#8412=CARTESIAN_POINT('Ctrl Pts',(3.81823436515222,1.45691693990942,54.0620260283815));
#8413=CARTESIAN_POINT('Ctrl Pts',(3.7739618456986,1.56801985017223,54.0678411685301));
#8414=CARTESIAN_POINT('Ctrl Pts',(3.7249610270647,1.676869209822,54.0736563086787));
#8415=CARTESIAN_POINT('Ctrl Pts',(3.67592793502284,1.78579026092283,54.0794752788529));
#8416=CARTESIAN_POINT('Ctrl Pts',(3.62216052476994,1.89245444210414,54.0852942490271));
#8417=CARTESIAN_POINT('Ctrl Pts',(3.56391066560922,1.99643827040979,54.0911132192014));
#8418=CARTESIAN_POINT('Ctrl Pts',(3.50557883736368,2.10056842454979,54.0969403778187));
#8419=CARTESIAN_POINT('Ctrl Pts',(3.44275218512514,2.20201035260932,54.1027675364361));
#8420=CARTESIAN_POINT('Ctrl Pts',(3.37572551094116,2.30037002996932,54.1085946950534));
#8421=CARTESIAN_POINT('Ctrl Pts',(3.36108353271044,2.32185670333062,54.1098676379625));
#8422=CARTESIAN_POINT('Ctrl Pts',(3.3462412776424,2.34319641899314,54.1111405808716));
#8423=CARTESIAN_POINT('Ctrl Pts',(3.33120206516043,2.36438529031773,54.1124135237807));
#8424=CARTESIAN_POINT('Ctrl Pts',(3.2623630904796,2.46137309326144,54.1182401642909));
#8425=CARTESIAN_POINT('Ctrl Pts',(3.18917535426923,2.55550639195625,54.1240668048011));
#8426=CARTESIAN_POINT('Ctrl Pts',(3.11190358208296,2.64637130724682,54.1298934453113));
#8427=CARTESIAN_POINT('Ctrl Pts',(3.0347284777701,2.73712254948601,54.1357127966274));
#8428=CARTESIAN_POINT('Ctrl Pts',(2.95347976177254,2.8246132331025,54.1415321479435));
#8429=CARTESIAN_POINT('Ctrl Pts',(2.86846498941049,2.90845897418655,54.1473514992596));
#8430=CARTESIAN_POINT('Ctrl Pts',(2.78353448469444,2.99222160638221,54.153165082366));
#8431=CARTESIAN_POINT('Ctrl Pts',(2.69484563885741,3.0723461989703,54.1589786654723));
#8432=CARTESIAN_POINT('Ctrl Pts',(2.60274536947073,3.14848241883271,54.1647922485787));
#8433=CARTESIAN_POINT('Ctrl Pts',(2.50777490372805,3.22699133426121,54.1707870051513));
#8434=CARTESIAN_POINT('Ctrl Pts',(2.40917719148304,3.30125888272042,54.1767817617239));
#8435=CARTESIAN_POINT('Ctrl Pts',(2.30737293390592,3.37094276781413,54.1827765182965));
#8436=CARTESIAN_POINT('Ctrl Pts',(2.20875462587246,3.43844590578392,54.1885836698277));
#8437=CARTESIAN_POINT('Ctrl Pts',(2.10712783743867,3.5016477449496,54.1943908213588));
#8438=CARTESIAN_POINT('Ctrl Pts',(2.00290695190488,3.56027930674141,54.2001979728899));
#8439=CARTESIAN_POINT('Ctrl Pts',(1.89870098017042,3.61890247847453,54.2060042934293));
#8440=CARTESIAN_POINT('Ctrl Pts',(1.79190200493657,3.67295647360696,54.2118106139687));
#8441=CARTESIAN_POINT('Ctrl Pts',(1.68295057692418,3.72221739768523,54.2176169345081));
#8442=CARTESIAN_POINT('Ctrl Pts',(1.57398910921333,3.77148286107823,54.2234237900906));
#8443=CARTESIAN_POINT('Ctrl Pts',(1.46287516597445,3.81595420724559,54.2292306456731));
#8444=CARTESIAN_POINT('Ctrl Pts',(1.35007032822716,3.85545524015525,54.2350375012555));
#8445=CARTESIAN_POINT('Ctrl Pts',(1.23722855899427,3.89496920541655,54.2408462579604));
#8446=CARTESIAN_POINT('Ctrl Pts',(1.12269517896059,3.92950948642712,54.2466550146653));
#8447=CARTESIAN_POINT('Ctrl Pts',(1.00694739929703,3.95894959996322,54.2524637713702));
#8448=CARTESIAN_POINT('Ctrl Pts',(0.891072419772218,3.98842206641674,54.25827891155));
#8449=CARTESIAN_POINT('Ctrl Pts',(0.773980772256783,4.01278307757026,54.2640940517297));
#8450=CARTESIAN_POINT('Ctrl Pts',(0.656160491151446,4.0319571438511,54.2699091919095));
#8451=CARTESIAN_POINT('Ctrl Pts',(0.53826261007532,4.05114383874705,54.275728162115));
#8452=CARTESIAN_POINT('Ctrl Pts',(0.419635543697051,4.06513673733663,54.2815471323205));
#8453=CARTESIAN_POINT('Ctrl Pts',(0.300771453023509,4.07391231288133,54.2873661025261));
#8454=CARTESIAN_POINT('Ctrl Pts',(0.181740097042269,4.08270023739817,54.2931932611747));
#8455=CARTESIAN_POINT('Ctrl Pts',(0.0624714571839893,4.08625617385383,54.2990204198233));
#8456=CARTESIAN_POINT('Ctrl Pts',(-0.0565431931913263,4.08460865534309,
54.3048475784719));
#8457=CARTESIAN_POINT('Ctrl Pts',(-0.0825419396795343,4.08424875497822,
54.3061205210884));
#8458=CARTESIAN_POINT('Ctrl Pts',(-0.108528590220755,4.08364073970447,54.3073934637049));
#8459=CARTESIAN_POINT('Ctrl Pts',(-0.134498071919463,4.08278523420593,54.3086664063214));
#8460=CARTESIAN_POINT('Ctrl Pts',(-0.253368185723169,4.07886932871536,54.314493046816));
#8461=CARTESIAN_POINT('Ctrl Pts',(-0.372256320073657,4.06975153930717,54.3203196873106));
#8462=CARTESIAN_POINT('Ctrl Pts',(-0.490671232428501,4.05542436024482,54.3261463278052));
#8463=CARTESIAN_POINT('Ctrl Pts',(-0.608938006365209,4.04111510464835,54.3319656791055));
#8464=CARTESIAN_POINT('Ctrl Pts',(-0.726732334459119,4.0216094705717,54.3377850304058));
#8465=CARTESIAN_POINT('Ctrl Pts',(-0.843563949405264,3.99695194657927,54.3436043817061));
#8466=CARTESIAN_POINT('Ctrl Pts',(-0.960279759471247,3.97231886341659,54.3494179647965));
#8467=CARTESIAN_POINT('Ctrl Pts',(-1.07603435803646,3.94254413340492,54.3552315478869));
#8468=CARTESIAN_POINT('Ctrl Pts',(-1.19034416555116,3.90772386019513,54.3610451309773));
#8469=CARTESIAN_POINT('Ctrl Pts',(-1.3082163039442,3.87181845407204,54.3670398875558));
#8470=CARTESIAN_POINT('Ctrl Pts',(-1.42455168744414,3.83054792954459,54.3730346441343));
#8471=CARTESIAN_POINT('Ctrl Pts',(-1.53883273829007,3.78407436549107,54.3790294007129));
#8472=CARTESIAN_POINT('Ctrl Pts',(-1.64953737972976,3.73905518508553,54.3848365522278));
#8473=CARTESIAN_POINT('Ctrl Pts',(-1.75831394566974,3.68915393029484,54.3906437037427));
#8474=CARTESIAN_POINT('Ctrl Pts',(-1.864709496909,3.63456785493646,54.3964508552576));
#8475=CARTESIAN_POINT('Ctrl Pts',(-1.97108982315693,3.57998959073666,54.4022571757807));
#8476=CARTESIAN_POINT('Ctrl Pts',(-2.07508944957714,3.52072802535044,54.4080634963038));
#8477=CARTESIAN_POINT('Ctrl Pts',(-2.17627860618468,3.45702710840729,54.4138698168269));
#8478=CARTESIAN_POINT('Ctrl Pts',(-2.27747708720895,3.39332032152792,54.419676672393));
#8479=CARTESIAN_POINT('Ctrl Pts',(-2.37586423837257,3.32517358701314,54.4254835279591));
#8480=CARTESIAN_POINT('Ctrl Pts',(-2.47103847327306,3.25287470764005,54.4312903835252));
#8481=CARTESIAN_POINT('Ctrl Pts',(-2.56624386752803,3.18055215813803,54.4370991402137));
#8482=CARTESIAN_POINT('Ctrl Pts',(-2.65823392895141,3.10407500677429,54.4429078969023));
#8483=CARTESIAN_POINT('Ctrl Pts',(-2.74663991379978,3.02377151648763,54.4487166535908));
#8484=CARTESIAN_POINT('Ctrl Pts',(-2.83514305151773,2.94337977748647,54.4545317937542));
#8485=CARTESIAN_POINT('Ctrl Pts',(-2.92005394894313,2.85915358080764,54.4603469339175));
#8486=CARTESIAN_POINT('Ctrl Pts',(-3.00104042498547,2.77145834671983,54.4661620740809));
#8487=CARTESIAN_POINT('Ctrl Pts',(-3.08208024115021,2.68370535392035,54.47198104427));
#8488=CARTESIAN_POINT('Ctrl Pts',(-3.15919022558717,2.59247908405389,54.4778000144592));
#8489=CARTESIAN_POINT('Ctrl Pts',(-3.23207926232517,2.49817706379023,54.4836189846483));
#8490=CARTESIAN_POINT('Ctrl Pts',(-3.30507086836956,2.4037423419127,54.4894461432806));
#8491=CARTESIAN_POINT('Ctrl Pts',(-3.37382943801791,2.30622356340577,54.4952733019129));
#8492=CARTESIAN_POINT('Ctrl Pts',(-3.43810776735536,2.20604623252795,54.5011004605452));
#8493=CARTESIAN_POINT('Ctrl Pts',(-3.45214936805756,2.18416249513002,54.5023734033175));
#8494=CARTESIAN_POINT('Ctrl Pts',(-3.46597734689685,2.1621519781996,54.5036463460897));
#8495=CARTESIAN_POINT('Ctrl Pts',(-3.47958942653237,2.14001925756852,54.504919288862));
#8496=CARTESIAN_POINT('Ctrl Pts',(-3.54356996194138,2.03598935516193,54.5109024716155));
#8497=CARTESIAN_POINT('Ctrl Pts',(-3.60297137049294,1.92894186180992,54.516885654369));
#8498=CARTESIAN_POINT('Ctrl Pts',(-3.65750670425542,1.81930473212342,54.5228688371224));
#8499=CARTESIAN_POINT('Ctrl Pts',(-3.71196228215891,1.70982794258433,54.5288432696979));
#8500=CARTESIAN_POINT('Ctrl Pts',(-3.76156578514888,1.59776939164976,54.5348177022733));
#8501=CARTESIAN_POINT('Ctrl Pts',(-3.80607433331058,1.48358456763152,54.5407921348488));
#8502=CARTESIAN_POINT('Ctrl Pts',(-3.85190504303721,1.36600779326105,54.546944042661));
#8503=CARTESIAN_POINT('Ctrl Pts',(-3.89233313914355,1.24617677374807,54.5530959504732));
#8504=CARTESIAN_POINT('Ctrl Pts',(-3.92714445344491,1.12461613085394,54.5592478582854));
#8505=CARTESIAN_POINT('Ctrl Pts',(-3.96086078617512,1.00687914892803,54.5652062593078));
#8506=CARTESIAN_POINT('Ctrl Pts',(-3.98930823046686,0.887520109317343,54.5711646603301));
#8507=CARTESIAN_POINT('Ctrl Pts',(-4.01234118947697,0.767035318108995,54.5771230613525));
#8508=CARTESIAN_POINT('Ctrl Pts',(-4.03649618624754,0.640681177450641,54.5833717225597));
#8509=CARTESIAN_POINT('Ctrl Pts',(-4.05469572660276,0.513089233302163,54.5896203837668));
#8510=CARTESIAN_POINT('Ctrl Pts',(-4.06683129097684,0.384848347705532,54.595869044974));
#8511=CARTESIAN_POINT('Ctrl Pts',(-4.07896685535091,0.256607462108901,54.6021177061812));
#8512=CARTESIAN_POINT('Ctrl Pts',(-4.08503835513097,0.127718109681303,54.6083663673883));
#8513=CARTESIAN_POINT('Ctrl Pts',(-4.08499981754229,-0.00122093384916138,
54.6146150285955));
#8514=CARTESIAN_POINT('Ctrl Pts',(-4.08499981754213,-0.00122093438980094,
54.6146150286217));
#8515=CARTESIAN_POINT('Ctrl Pts',(-4.0849613114778,-0.130054446722099,54.6208585755618));
#8516=CARTESIAN_POINT('Ctrl Pts',(-4.0788238307835,-0.258718368127277,54.6271021225019));
#8517=CARTESIAN_POINT('Ctrl Pts',(-4.06666054896851,-0.386648392552093,
54.633345669442));
#8518=CARTESIAN_POINT('Ctrl Pts',(-4.05445122125751,-0.515062714939471,
54.6396128522493));
#8519=CARTESIAN_POINT('Ctrl Pts',(-4.03617046827928,-0.642737277144754,
54.6458800350566));
#8520=CARTESIAN_POINT('Ctrl Pts',(-4.01194308905835,-0.769114848482948,
54.6521472178638));
#8521=CARTESIAN_POINT('Ctrl Pts',(-3.98766880109497,-0.895737110461865,
54.6584265351105));
#8522=CARTESIAN_POINT('Ctrl Pts',(-3.95742496150907,-1.02105707251704,54.6647058523571));
#8523=CARTESIAN_POINT('Ctrl Pts',(-3.92138638497742,-1.14453214009642,54.6709851696037));
#8524=CARTESIAN_POINT('Ctrl Pts',(-3.88523988384411,-1.26837697803763,54.6772832915002));
#8525=CARTESIAN_POINT('Ctrl Pts',(-3.8432640256831,-1.39036558117875,54.6835814133967));
#8526=CARTESIAN_POINT('Ctrl Pts',(-3.79568276842705,-1.5099726227538,54.6898795352932));
#8527=CARTESIAN_POINT('Ctrl Pts',(-3.76724477624178,-1.58145842009854,54.6936437473296));
#8528=CARTESIAN_POINT('Ctrl Pts',(-3.73680536935565,-1.65209393914338,54.6974079593661));
#8529=CARTESIAN_POINT('Ctrl Pts',(-3.70442010209234,-1.72177138645471,54.7011721714026));
#8530=CARTESIAN_POINT('Ctrl Pts',(-3.65429334650934,-1.82961994433828,54.7069985163014));
#8531=CARTESIAN_POINT('Ctrl Pts',(-3.59937314424357,-1.93544927103489,54.7128248612001));
#8532=CARTESIAN_POINT('Ctrl Pts',(-3.53984483140051,-2.03880444614168,54.7186512060989));
#8533=CARTESIAN_POINT('Ctrl Pts',(-3.4803877596237,-2.14203592997411,54.7244705782648));
#8534=CARTESIAN_POINT('Ctrl Pts',(-3.41633374565396,-2.24279880006085,54.7302899504308));
#8535=CARTESIAN_POINT('Ctrl Pts',(-3.34791561976592,-2.34065930945265,54.7361093225967));
#8536=CARTESIAN_POINT('Ctrl Pts',(-3.27814446330158,-2.44045509929389,54.7420437781323));
#8537=CARTESIAN_POINT('Ctrl Pts',(-3.20383491891496,-2.53723212144727,54.7479782336679));
#8538=CARTESIAN_POINT('Ctrl Pts',(-3.12528286286086,-2.63055736054324,54.7539126892035));
#8539=CARTESIAN_POINT('Ctrl Pts',(-3.04838984166705,-2.72191155224996,54.759721807872));
#8540=CARTESIAN_POINT('Ctrl Pts',(-2.96743201131959,-2.80995798811599,54.7655309265405));
#8541=CARTESIAN_POINT('Ctrl Pts',(-2.8827296257502,-2.89432114749246,54.7713400452091));
#8542=CARTESIAN_POINT('Ctrl Pts',(-2.79528594698747,-2.98141462140509,54.7773371691782));
#8543=CARTESIAN_POINT('Ctrl Pts',(-2.70385149272671,-3.06458200391232,54.7833342931474));
#8544=CARTESIAN_POINT('Ctrl Pts',(-2.60882163596673,-3.14344948610787,54.7893314171166));
#8545=CARTESIAN_POINT('Ctrl Pts',(-2.51379177920677,-3.22231696830342,54.7953285410857));
#8546=CARTESIAN_POINT('Ctrl Pts',(-2.41516688168822,-3.29688423591414,54.8013256650549));
#8547=CARTESIAN_POINT('Ctrl Pts',(-2.31338095599002,-3.36682247118299,54.8073227890241));
#8548=CARTESIAN_POINT('',(-4.08499997893751,-0.000414825933522758,54.5103849713796));
#8549=CARTESIAN_POINT('Ctrl Pts',(-4.08499997893746,-0.000414826442725132,
54.5103849714045));
#8550=CARTESIAN_POINT('Ctrl Pts',(-4.08499760796101,-0.0237629974469017,
54.5115287470813));
#8551=CARTESIAN_POINT('Ctrl Pts',(-4.08479506611947,-0.0471099734563326,
54.5126725227581));
#8552=CARTESIAN_POINT('Ctrl Pts',(-4.08439240353752,-0.0704534876710844,
54.5138162984348));
#8553=CARTESIAN_POINT('Ctrl Pts',(-4.08234110579074,-0.189373149582664,
54.5196430739379));
#8554=CARTESIAN_POINT('Ctrl Pts',(-4.07508860521704,-0.308392412691008,
54.5254698494409));
#8555=CARTESIAN_POINT('Ctrl Pts',(-4.06261969266714,-0.427020178391096,
54.531296624944));
#8556=CARTESIAN_POINT('Ctrl Pts',(-4.05016644986693,-0.54549886393775,54.5371160779068));
#8557=CARTESIAN_POINT('Ctrl Pts',(-4.03250987681782,-0.663586628572482,
54.5429355308697));
#8558=CARTESIAN_POINT('Ctrl Pts',(-4.00968677161816,-0.780792541915143,
54.5487549838325));
#8559=CARTESIAN_POINT('Ctrl Pts',(-3.98688641878641,-0.897881612609194,
54.554568635379));
#8560=CARTESIAN_POINT('Ctrl Pts',(-3.95892985829082,-1.01409018293799,54.5603822869256));
#8561=CARTESIAN_POINT('Ctrl Pts',(-3.92590560378646,-1.12893320890038,54.5661959384721));
#8562=CARTESIAN_POINT('Ctrl Pts',(-3.89290572395898,-1.24369147105227,54.5720052990549));
#8563=CARTESIAN_POINT('Ctrl Pts',(-3.85484570588691,-1.35708580391272,54.5778146596377));
#8564=CARTESIAN_POINT('Ctrl Pts',(-3.81186484778546,-1.46864270066532,54.5836240202205));
#8565=CARTESIAN_POINT('Ctrl Pts',(-3.76890092317954,-1.58015564649891,54.5894310920454));
#8566=CARTESIAN_POINT('Ctrl Pts',(-3.72102016028149,-1.68983221586267,54.5952381638702));
#8567=CARTESIAN_POINT('Ctrl Pts',(-3.66841113396372,-1.79721583350776,54.601045235695));
#8568=CARTESIAN_POINT('Ctrl Pts',(-3.61581045826974,-1.90458240616543,54.6068513857641));
#8569=CARTESIAN_POINT('Ctrl Pts',(-3.55848319159784,-2.00965638510735,54.6126575358332));
#8570=CARTESIAN_POINT('Ctrl Pts',(-3.49666503069175,-2.11200347138385,54.6184636859023));
#8571=CARTESIAN_POINT('Ctrl Pts',(-3.4348421398624,-2.21435838859317,54.6242702802202));
#8572=CARTESIAN_POINT('Ctrl Pts',(-3.36852788294009,-2.31398564958607,54.6300768745381));
#8573=CARTESIAN_POINT('Ctrl Pts',(-3.29800233105639,-2.41047829783772,54.635883468856));
#8574=CARTESIAN_POINT('Ctrl Pts',(-3.2274156120223,-2.50705463462734,54.6416950992611));
#8575=CARTESIAN_POINT('Ctrl Pts',(-3.15261054266328,-2.60049059795527,54.6475067296662));
#8576=CARTESIAN_POINT('Ctrl Pts',(-3.07390881038207,-2.69041067970217,54.6533183600713));
#8577=CARTESIAN_POINT('Ctrl Pts',(-2.99517263341694,-2.78037011596775,54.6591325340007));
#8578=CARTESIAN_POINT('Ctrl Pts',(-2.91253667615821,-2.86681030866367,54.6649467079301));
#8579=CARTESIAN_POINT('Ctrl Pts',(-2.82635983936874,-2.94939232019132,54.6707608818596));
#8580=CARTESIAN_POINT('Ctrl Pts',(-2.74005896454961,-3.03209319556193,54.6765834243797));
#8581=CARTESIAN_POINT('Ctrl Pts',(-2.65020733296229,-3.11092452379591,54.6824059668999));
#8582=CARTESIAN_POINT('Ctrl Pts',(-2.5571976537131,-3.18558709814128,54.6882285094201));
#8583=CARTESIAN_POINT('Ctrl Pts',(-2.4781218381537,-3.24906440508164,54.6931787716092));
#8584=CARTESIAN_POINT('Ctrl Pts',(-2.39676397863391,-3.30952907413331,54.6981290337984));
#8585=CARTESIAN_POINT('Ctrl Pts',(-2.31338095599002,-3.36682247118298,54.7030792959875));
#8586=CARTESIAN_POINT('Ctrl Pts',(-2.31338095599002,-3.36682247118299,53.4530632234442));
#8587=CARTESIAN_POINT('Ctrl Pts',(-2.21483110028557,-3.43453716696917,53.458871188923));
#8588=CARTESIAN_POINT('Ctrl Pts',(-2.11333532917852,-3.49790096330531,53.4646791544019));
#8589=CARTESIAN_POINT('Ctrl Pts',(-2.00931967003337,-3.55666409204145,53.4704871198808));
#8590=CARTESIAN_POINT('Ctrl Pts',(-1.90519361781242,-3.6154895867961,53.4763012494236));
#8591=CARTESIAN_POINT('Ctrl Pts',(-1.79854269304458,-3.66970446364335,53.4821153789664));
#8592=CARTESIAN_POINT('Ctrl Pts',(-1.68981715296657,-3.71910513289688,53.4879295085092));
#8593=CARTESIAN_POINT('Ctrl Pts',(-1.58102771926253,-3.76853483293643,53.493747054782));
#8594=CARTESIAN_POINT('Ctrl Pts',(-1.47016161960171,-3.81314453778066,53.4995646010548));
#8595=CARTESIAN_POINT('Ctrl Pts',(-1.35768711150758,-3.85277960792545,53.5053821473277));
#8596=CARTESIAN_POINT('Ctrl Pts',(-1.24504420052336,-3.89247402183155,53.511208403944));
#8597=CARTESIAN_POINT('Ctrl Pts',(-1.13078846152099,-3.92717880812908,53.5170346605604));
#8598=CARTESIAN_POINT('Ctrl Pts',(-1.01540158357285,-3.95678968661183,53.5228609171768));
#8599=CARTESIAN_POINT('Ctrl Pts',(-0.951426222865082,-3.97320720882488,
53.5260912400284));
#8600=CARTESIAN_POINT('Ctrl Pts',(-0.887103309351932,-3.98805974644403,
53.52932156288));
#8601=CARTESIAN_POINT('Ctrl Pts',(-0.822515744067601,-4.00133638310514,
53.5325518857316));
#8602=CARTESIAN_POINT('Ctrl Pts',(-0.706017010642136,-4.02528389294484,
53.5383785261864));
#8603=CARTESIAN_POINT('Ctrl Pts',(-0.588286158508163,-4.04417751280474,
53.5442051666412));
#8604=CARTESIAN_POINT('Ctrl Pts',(-0.469799099151263,-4.05789524340349,
53.5500318070961));
#8605=CARTESIAN_POINT('Ctrl Pts',(-0.35146026844917,-4.07159581296571,53.5558511583576));
#8606=CARTESIAN_POINT('Ctrl Pts',(-0.232367513824851,-4.08013332601978,
53.5616705096192));
#8607=CARTESIAN_POINT('Ctrl Pts',(-0.113007938716276,-4.08343656811112,
53.5674898608808));
#8608=CARTESIAN_POINT('Ctrl Pts',(0.00623332579019821,-4.08673653599039,
53.5733034439335));
#8609=CARTESIAN_POINT('Ctrl Pts',(0.125740479250513,-4.08481254346311,53.5791170269863));
#8610=CARTESIAN_POINT('Ctrl Pts',(0.245020869434864,-4.07764512599385,53.584930610039));
#8611=CARTESIAN_POINT('Ctrl Pts',(0.368018493961781,-4.07025434431255,53.5909253666321));
#8612=CARTESIAN_POINT('Ctrl Pts',(0.490774551486939,-4.05728792303876,53.5969201232251));
#8613=CARTESIAN_POINT('Ctrl Pts',(0.612747926644611,-4.03878261093522,53.6029148798182));
#8614=CARTESIAN_POINT('Ctrl Pts',(0.730904161196627,-4.02085642012073,53.6087220312984));
#8615=CARTESIAN_POINT('Ctrl Pts',(0.848325537981576,-3.99773291183685,53.6145291827786));
#8616=CARTESIAN_POINT('Ctrl Pts',(0.964525580467868,-3.96949813006923,53.6203363342587));
#8617=CARTESIAN_POINT('Ctrl Pts',(1.08070899498276,-3.941267388637,53.6261426547483));
#8618=CARTESIAN_POINT('Ctrl Pts',(1.19567102660526,-3.90792692462295,53.6319489752378));
#8619=CARTESIAN_POINT('Ctrl Pts',(1.30893682451529,-3.86961359691479,53.6377552957274));
#8620=CARTESIAN_POINT('Ctrl Pts',(1.42221305970884,-3.83129673868752,53.6435621512612));
#8621=CARTESIAN_POINT('Ctrl Pts',(1.53379236409329,-3.78800623634791,53.6493690067949));
#8622=CARTESIAN_POINT('Ctrl Pts',(1.64321705206185,-3.73992817040824,53.6551758623287));
#8623=CARTESIAN_POINT('Ctrl Pts',(1.75267756490243,-3.69183436404847,53.6609846189861));
#8624=CARTESIAN_POINT('Ctrl Pts',(1.85998168524429,-3.63895004074933,53.6667933756435));
#8625=CARTESIAN_POINT('Ctrl Pts',(1.96469421522189,-3.58150829130321,53.6726021323009));
#8626=CARTESIAN_POINT('Ctrl Pts',(2.06952181802128,-3.52400341680225,53.6784172724352));
#8627=CARTESIAN_POINT('Ctrl Pts',(2.17175178805305,-3.46193131564877,53.6842324125695));
#8628=CARTESIAN_POINT('Ctrl Pts',(2.27097580354513,-3.39556974596496,53.6900475527038));
#8629=CARTESIAN_POINT('Ctrl Pts',(2.37026517097005,-3.32916446854745,53.695866522865));
#8630=CARTESIAN_POINT('Ctrl Pts',(2.46654431298234,-3.25846433685901,53.7016854930262));
#8631=CARTESIAN_POINT('Ctrl Pts',(2.55943734126607,-3.18378791632434,53.7075044631874));
#8632=CARTESIAN_POINT('Ctrl Pts',(2.6524610884637,-3.10900641125569,53.7133316217937));
#8633=CARTESIAN_POINT('Ctrl Pts',(2.74208890681506,-3.03023771809086,53.7191587803999));
#8634=CARTESIAN_POINT('Ctrl Pts',(2.82798107374755,-2.94783785960586,53.7249859390062));
#8635=CARTESIAN_POINT('Ctrl Pts',(2.8467442219051,-2.92983760640314,53.7262588820949));
#8636=CARTESIAN_POINT('Ctrl Pts',(2.86532925483141,-2.91166419900583,53.7275318251835));
#8637=CARTESIAN_POINT('Ctrl Pts',(2.88373288971329,-2.89332155502734,53.7288047682722));
#8638=CARTESIAN_POINT('Ctrl Pts',(2.96797181797925,-2.80936180032512,53.7346314086191));
#8639=CARTESIAN_POINT('Ctrl Pts',(3.04867504377748,-2.72158645576335,53.740458048966));
#8640=CARTESIAN_POINT('Ctrl Pts',(3.12547828030272,-2.63032517369164,53.7462846893129));
#8641=CARTESIAN_POINT('Ctrl Pts',(3.20218543505863,-2.53917806057751,53.752104040463));
#8642=CARTESIAN_POINT('Ctrl Pts',(3.2750020446252,-2.444553993408,53.757923391613));
#8643=CARTESIAN_POINT('Ctrl Pts',(3.34360000726998,-2.34681997421707,53.763742742763));
#8644=CARTESIAN_POINT('Ctrl Pts',(3.41212997477236,-2.24918283018534,53.7695563257007));
#8645=CARTESIAN_POINT('Ctrl Pts',(3.47644938138893,-2.14844219876397,53.7753699086384));
#8646=CARTESIAN_POINT('Ctrl Pts',(3.53627022838904,-2.04499825716534,53.7811834915762));
#8647=CARTESIAN_POINT('Ctrl Pts',(3.59795532401731,-1.938330602833,53.787178248211));
#8648=CARTESIAN_POINT('Ctrl Pts',(3.65485659782205,-1.82878872493102,53.7931730048459));
#8649=CARTESIAN_POINT('Ctrl Pts',(3.706706203894,-1.7168442323093,53.7991677614808));
#8650=CARTESIAN_POINT('Ctrl Pts',(3.75693318200392,-1.60840303079596,53.804974912838));
#8651=CARTESIAN_POINT('Ctrl Pts',(3.80241977601923,-1.49770774825449,53.8107820641953));
#8652=CARTESIAN_POINT('Ctrl Pts',(3.84296939715654,-1.3852116129019,53.8165892155525));
#8653=CARTESIAN_POINT('Ctrl Pts',(3.88351321571274,-1.27273157555301,53.8223955359164));
#8654=CARTESIAN_POINT('Ctrl Pts',(3.91912132817581,-1.158451581456,53.8282018562802));
#8655=CARTESIAN_POINT('Ctrl Pts',(3.94964594291672,-1.04284319319898,53.8340081766441));
#8656=CARTESIAN_POINT('Ctrl Pts',(3.98017337044418,-0.927224151843767,53.8398150320496));
#8657=CARTESIAN_POINT('Ctrl Pts',(4.0056162647757,-0.810276867263508,53.8456218874551));
#8658=CARTESIAN_POINT('Ctrl Pts',(4.02587735828219,-0.69248573708837,53.8514287428606));
#8659=CARTESIAN_POINT('Ctrl Pts',(4.04614508511947,-0.574656042976366,53.8572374993872));
#8660=CARTESIAN_POINT('Ctrl Pts',(4.06122756804862,-0.455982355514988,53.8630462559138));
#8661=CARTESIAN_POINT('Ctrl Pts',(4.07107915507459,-0.336956248075587,53.8688550124405));
#8662=CARTESIAN_POINT('Ctrl Pts',(4.08094156840191,-0.217799338106082,53.874670152441));
#8663=CARTESIAN_POINT('Ctrl Pts',(4.08556157816917,-0.0982896417554054,
53.8804852924415));
#8664=CARTESIAN_POINT('Ctrl Pts',(4.08494561455591,0.021079044579889,53.886300432442));
#8665=CARTESIAN_POINT('Ctrl Pts',(4.08432924525062,0.140526350698755,53.8921194024675));
#8666=CARTESIAN_POINT('Ctrl Pts',(4.0784700544374,0.259832055481758,53.897938372493));
#8667=CARTESIAN_POINT('Ctrl Pts',(4.06742640050331,0.378506904149321,53.9037573425185));
#8668=CARTESIAN_POINT('Ctrl Pts',(4.05636720596094,0.497348751832471,53.9095845009872));
#8669=CARTESIAN_POINT('Ctrl Pts',(4.04010904303405,0.615557569138881,53.915411659456));
#8670=CARTESIAN_POINT('Ctrl Pts',(4.01876146302421,0.732653603902604,53.9212388179247));
#8671=CARTESIAN_POINT('Ctrl Pts',(4.01409807857125,0.758233263412903,53.9225117622208));
#8672=CARTESIAN_POINT('Ctrl Pts',(4.00919201371126,0.783759877033307,53.9237847065168));
#8673=CARTESIAN_POINT('Ctrl Pts',(4.0040447251659,0.809228545511804,53.9250576508129));
#8674=CARTESIAN_POINT('Ctrl Pts',(3.98048407096562,0.925806134989238,53.9308842914046));
#8675=CARTESIAN_POINT('Ctrl Pts',(3.9517904716661,1.04153945104153,53.9367109319963));
#8676=CARTESIAN_POINT('Ctrl Pts',(3.91803793295716,1.15594279958342,53.942537572588));
#8677=CARTESIAN_POINT('Ctrl Pts',(3.88432761905494,1.27020302824562,53.9483569239866));
#8678=CARTESIAN_POINT('Ctrl Pts',(3.84557106839036,1.38313621100127,53.9541762753851));
#8679=CARTESIAN_POINT('Ctrl Pts',(3.80189340042581,1.49426623190069,53.9599956267837));
#8680=CARTESIAN_POINT('Ctrl Pts',(3.75825902627393,1.60528609943041,53.9658092099735));
#8681=CARTESIAN_POINT('Ctrl Pts',(3.70971338740881,1.71450598344587,53.9716227931632));
#8682=CARTESIAN_POINT('Ctrl Pts',(3.65643139642823,1.82146491682215,53.977436376353));
#8683=CARTESIAN_POINT('Ctrl Pts',(3.60148893606277,1.93175709715565,53.9834311328947));
#8684=CARTESIAN_POINT('Ctrl Pts',(3.54151020734356,2.03964467537803,53.9894258894364));
#8685=CARTESIAN_POINT('Ctrl Pts',(3.47674081996221,2.14464408954225,53.9954206459781));
#8686=CARTESIAN_POINT('Ctrl Pts',(3.41399837996478,2.24635756421471,54.0012277975943));
#8687=CARTESIAN_POINT('Ctrl Pts',(3.34676088525576,2.34536057575913,54.0070349492106));
#8688=CARTESIAN_POINT('Ctrl Pts',(3.27529792236496,2.44123913612571,54.0128421008269));
#8689=CARTESIAN_POINT('Ctrl Pts',(3.20384518567459,2.53710397647096,54.0186484214519));
#8690=CARTESIAN_POINT('Ctrl Pts',(3.12816842699467,2.62984492794562,54.0244547420769));
#8691=CARTESIAN_POINT('Ctrl Pts',(3.04857944346241,2.71907858968777,54.0302610627019));
#8692=CARTESIAN_POINT('Ctrl Pts',(2.96898312592808,2.8083204741742,54.0360679183704));
#8693=CARTESIAN_POINT('Ctrl Pts',(2.8854741382294,2.89405412199044,54.0418747740389));
#8694=CARTESIAN_POINT('Ctrl Pts',(2.79840285378173,2.97593119341599,54.0476816297074));
#8695=CARTESIAN_POINT('Ctrl Pts',(2.71130306282304,3.05783507080462,54.0534903864987));
#8696=CARTESIAN_POINT('Ctrl Pts',(2.62063895255242,3.13587958147787,54.0592991432899));
#8697=CARTESIAN_POINT('Ctrl Pts',(2.52679535449982,3.20975547923484,54.0651079000811));
#8698=CARTESIAN_POINT('Ctrl Pts',(2.43284862796809,3.28371256216736,54.0709230403472));
#8699=CARTESIAN_POINT('Ctrl Pts',(2.33571576002902,3.35349163592164,54.0767381806133));
#8700=CARTESIAN_POINT('Ctrl Pts',(2.23581216669383,3.41882566903664,54.0825533208794));
#8701=CARTESIAN_POINT('Ctrl Pts',(2.13584277385464,3.48420273310608,54.0883722911714));
#8702=CARTESIAN_POINT('Ctrl Pts',(2.03309937117241,3.54512871841213,54.0941912614633));
#8703=CARTESIAN_POINT('Ctrl Pts',(1.92802223191034,3.60138241141641,54.1000102317553));
#8704=CARTESIAN_POINT('Ctrl Pts',(1.822797228322,3.65771526449751,54.1058373904899));
#8705=CARTESIAN_POINT('Ctrl Pts',(1.71523230008273,3.70936252723781,54.1116645492244));
#8706=CARTESIAN_POINT('Ctrl Pts',(1.60578803419549,3.75615092737693,54.117491707959));
#8707=CARTESIAN_POINT('Ctrl Pts',(1.58187995360847,3.76637184513809,54.1187646497571));
#8708=CARTESIAN_POINT('Ctrl Pts',(1.55788224752409,3.77636108546979,54.1200375915553));
#8709=CARTESIAN_POINT('Ctrl Pts',(1.5337998058897,3.78611716081961,54.1213105333535));
#8710=CARTESIAN_POINT('Ctrl Pts',(1.42356717029867,3.83077367510339,54.127137173837));
#8711=CARTESIAN_POINT('Ctrl Pts',(1.31120722579543,3.87068314002797,54.1329638143204));
#8712=CARTESIAN_POINT('Ctrl Pts',(1.1971659072405,3.90563935746006,54.1387904548039));
#8713=CARTESIAN_POINT('Ctrl Pts',(1.08326725568749,3.94055184426187,54.144609806093));
#8714=CARTESIAN_POINT('Ctrl Pts',(0.967691800422726,3.97052329033378,54.1504291573822));
#8715=CARTESIAN_POINT('Ctrl Pts',(0.850905683399544,3.9953954144688,54.1562485086714));
#8716=CARTESIAN_POINT('Ctrl Pts',(0.734235326157389,4.0202428850601,54.1620620917507));
#8717=CARTESIAN_POINT('Ctrl Pts',(0.61635709116518,4.04000100490577,54.16787567483));
#8718=CARTESIAN_POINT('Ctrl Pts',(0.497751952524549,4.05456138118021,54.1736892579093));
#8719=CARTESIAN_POINT('Ctrl Pts',(0.375450623738313,4.06957551451712,54.179684014492));
#8720=CARTESIAN_POINT('Ctrl Pts',(0.252376765074173,4.07906250494079,54.1856787710747));
#8721=CARTESIAN_POINT('Ctrl Pts',(0.129069195615655,4.08296046303943,54.1916735276574));
#8722=CARTESIAN_POINT('Ctrl Pts',(0.00962051950209979,4.08673643507807,
54.1974806791613));
#8723=CARTESIAN_POINT('Ctrl Pts',(-0.110047020198127,4.08526796015158,54.2032878306652));
#8724=CARTESIAN_POINT('Ctrl Pts',(-0.229439408649957,4.07855152692207,54.2090949821692));
#8725=CARTESIAN_POINT('Ctrl Pts',(-0.348814712290411,4.07183605480069,54.2149013026814));
#8726=CARTESIAN_POINT('Ctrl Pts',(-0.467914535926838,4.05987414081413,54.2207076231936));
#8727=CARTESIAN_POINT('Ctrl Pts',(-0.586247092284356,4.04271435384546,54.2265139437057));
#8728=CARTESIAN_POINT('Ctrl Pts',(-0.704590552797133,4.02555298562995,54.2323207992611));
#8729=CARTESIAN_POINT('Ctrl Pts',(-0.822166201852386,4.00319285064147,54.2381276548164));
#8730=CARTESIAN_POINT('Ctrl Pts',(-0.938490216218402,3.97573403462333,54.2439345103717));
#8731=CARTESIAN_POINT('Ctrl Pts',(-1.05485231422392,3.94826622878778,54.2497432670494));
#8732=CARTESIAN_POINT('Ctrl Pts',(-1.16996156588243,3.91569651569341,54.2555520237272));
#8733=CARTESIAN_POINT('Ctrl Pts',(-1.28334774707571,3.87817528743553,54.2613607804049));
#8734=CARTESIAN_POINT('Ctrl Pts',(-1.39685853288007,3.84061282559871,54.2671759205578));
#8735=CARTESIAN_POINT('Ctrl Pts',(-1.5086420812892,3.79808811560402,54.2729910607107));
#8736=CARTESIAN_POINT('Ctrl Pts',(-1.61824650749295,3.75080034672427,54.2788062008636));
#8737=CARTESIAN_POINT('Ctrl Pts',(-1.72792312246141,3.70348143270066,54.2846251710423));
#8738=CARTESIAN_POINT('Ctrl Pts',(-1.83541739071912,3.65139338944626,54.290444141221));
#8739=CARTESIAN_POINT('Ctrl Pts',(-1.94030193146339,3.59478141404445,54.2962631113997));
#8740=CARTESIAN_POINT('Ctrl Pts',(-2.04533406552763,3.53808977438192,54.3020902700218));
#8741=CARTESIAN_POINT('Ctrl Pts',(-2.14774879391313,3.47686170553716,54.3079174286439));
#8742=CARTESIAN_POINT('Ctrl Pts',(-2.24714751724139,3.41138579403676,54.3137445872661));
#8743=CARTESIAN_POINT('Ctrl Pts',(-2.26886116963209,3.39708258032658,54.3150175301421));
#8744=CARTESIAN_POINT('Ctrl Pts',(-2.29043102323381,3.38257680976385,54.3162904730181));
#8745=CARTESIAN_POINT('Ctrl Pts',(-2.31185313982904,3.36787174041154,54.3175634158941));
#8746=CARTESIAN_POINT('Ctrl Pts',(-2.40962137593576,3.30075938547629,54.3233729902702));
#8747=CARTESIAN_POINT('Ctrl Pts',(-2.50462505378427,3.22927620521925,54.3291825646463));
#8748=CARTESIAN_POINT('Ctrl Pts',(-2.59644759805791,3.15367799093999,54.3349921390224));
#8749=CARTESIAN_POINT('Ctrl Pts',(-2.68815504986841,3.07817453318005,54.340794431546));
#8750=CARTESIAN_POINT('Ctrl Pts',(-2.77668898388059,2.99856655800571,54.3465967240695));
#8751=CARTESIAN_POINT('Ctrl Pts',(-2.86166152162032,2.91515322679232,54.3523990165931));
#8752=CARTESIAN_POINT('Ctrl Pts',(-2.94654999687871,2.83182241555285,54.3581955689668));
#8753=CARTESIAN_POINT('Ctrl Pts',(-3.0278837930395,2.74469402282852,54.3639921213404));
#8754=CARTESIAN_POINT('Ctrl Pts',(-3.10530837555256,2.65410717430987,54.3697886737141));
#8755=CARTESIAN_POINT('Ctrl Pts',(-3.18355610618591,2.56255724156576,54.3756468527835));
#8756=CARTESIAN_POINT('Ctrl Pts',(-3.25781068237893,2.46747515130599,54.3815050318528));
#8757=CARTESIAN_POINT('Ctrl Pts',(-3.32774444873561,2.36924922368022,54.3873632109222));
#8758=CARTESIAN_POINT('Ctrl Pts',(-3.39686760748384,2.27216184025747,54.3931534873922));
#8759=CARTESIAN_POINT('Ctrl Pts',(-3.46176935901469,2.17200346539132,54.3989437638621));
#8760=CARTESIAN_POINT('Ctrl Pts',(-3.5221744930545,2.0691814421351,54.4047340403321));
#8761=CARTESIAN_POINT('Ctrl Pts',(-3.5825715191737,1.96637322023558,54.4105235395982));
#8762=CARTESIAN_POINT('Ctrl Pts',(-3.63847292019524,1.86090241487841,54.4163130388643));
#8763=CARTESIAN_POINT('Ctrl Pts',(-3.68964809220262,1.75320334123158,54.4221025381304));
#8764=CARTESIAN_POINT('Ctrl Pts',(-3.74082863267413,1.64549296955503,54.4278926447363));
#8765=CARTESIAN_POINT('Ctrl Pts',(-3.7872817823887,1.53555423576914,54.4336827513422));
#8766=CARTESIAN_POINT('Ctrl Pts',(-3.82882426433602,1.42384330346836,54.4394728579481));
#8767=CARTESIAN_POINT('Ctrl Pts',(-3.87122223430697,1.3098318980083,54.4453822007341));
#8768=CARTESIAN_POINT('Ctrl Pts',(-3.90850489483918,1.19397491631519,54.45129154352));
#8769=CARTESIAN_POINT('Ctrl Pts',(-3.94053066445184,1.07677438793591,54.457200886306));
#8770=CARTESIAN_POINT('Ctrl Pts',(-3.97195588228142,0.961771620520624,54.4629994162562));
#8771=CARTESIAN_POINT('Ctrl Pts',(-3.99831961112235,0.845475672892513,54.4687979462064));
#8772=CARTESIAN_POINT('Ctrl Pts',(-4.01953987707944,0.728370905904543,54.4745964761567));
#8773=CARTESIAN_POINT('Ctrl Pts',(-4.04136843803518,0.607909242060507,54.4805612253605));
#8774=CARTESIAN_POINT('Ctrl Pts',(-4.05775414418478,0.486592157322449,54.4865259745643));
#8775=CARTESIAN_POINT('Ctrl Pts',(-4.0686651095036,0.36495099220038,54.4924907237681));
#8776=CARTESIAN_POINT('Ctrl Pts',(-4.07957607482243,0.24330982707832,54.4984554729719));
#8777=CARTESIAN_POINT('Ctrl Pts',(-4.0850123434796,0.121345049922239,54.5044202221757));
#8778=CARTESIAN_POINT('Ctrl Pts',(-4.08499997893751,-0.000414825933535863,
54.5103849713796));
#8779=CARTESIAN_POINT('Origin',(0.,0.,46.4896150285955));
#8780=CARTESIAN_POINT('',(-2.31338095599002,-3.36682247118298,52.2032272635689));
#8781=CARTESIAN_POINT('',(-2.31338095599003,-3.36682247118298,52.3072351639912));
#8782=CARTESIAN_POINT('',(-2.31338095599002,-3.36682247118298,46.4896150285955));
#8783=CARTESIAN_POINT('',(-4.08499863636843,0.00333779389427079,53.3646150286363));
#8784=CARTESIAN_POINT('Ctrl Pts',(-2.31338095599003,-3.36682247118298,52.3072351639912));
#8785=CARTESIAN_POINT('Ctrl Pts',(-2.21493144244683,-3.43446822076041,52.3130540845183));
#8786=CARTESIAN_POINT('Ctrl Pts',(-2.11360661907073,-3.49772756075896,52.3188730050453));
#8787=CARTESIAN_POINT('Ctrl Pts',(-2.00984156052795,-3.55636920209004,52.3246919255724));
#8788=CARTESIAN_POINT('Ctrl Pts',(-1.90593025909387,-3.61509349092598,52.3305190470852));
#8789=CARTESIAN_POINT('Ctrl Pts',(-1.79957222056283,-3.66918690786224,52.336346168598));
#8790=CARTESIAN_POINT('Ctrl Pts',(-1.69122393906574,-3.71846562279806,52.3421732901108));
#8791=CARTESIAN_POINT('Ctrl Pts',(-1.66665354039674,-3.72964067472449,52.3434947203788));
#8792=CARTESIAN_POINT('Ctrl Pts',(-1.64198085808676,-3.74056832863762,52.3448161506469));
#8793=CARTESIAN_POINT('Ctrl Pts',(-1.61721132365331,-3.75124679735252,52.3461375809149));
#8794=CARTESIAN_POINT('Ctrl Pts',(-1.50799383531472,-3.79833187823997,52.3519642263563));
#8795=CARTESIAN_POINT('Ctrl Pts',(-1.39654450508684,-3.84071813988266,52.3577908717977));
#8796=CARTESIAN_POINT('Ctrl Pts',(-1.28330459644759,-3.87818956637456,52.363617517239));
#8797=CARTESIAN_POINT('Ctrl Pts',(-1.17020635109364,-3.91561411605911,52.3694368735387));
#8798=CARTESIAN_POINT('Ctrl Pts',(-1.05532236665007,-3.94813593315012,52.3752562298384));
#8799=CARTESIAN_POINT('Ctrl Pts',(-0.939115169065273,-3.97558645978571,
52.3810755861381));
#8800=CARTESIAN_POINT('Ctrl Pts',(-0.823023156410561,-4.00300977737525,
52.3868891742741));
#8801=CARTESIAN_POINT('Ctrl Pts',(-0.705610934579691,-4.02537171157905,
52.39270276241));
#8802=CARTESIAN_POINT('Ctrl Pts',(-0.587356961998321,-4.04255325248686,
52.3985163505459));
#8803=CARTESIAN_POINT('Ctrl Pts',(-0.465417887214954,-4.06027021502028,
52.4045111052505));
#8804=CARTESIAN_POINT('Ctrl Pts',(-0.342584159196125,-4.0724784877694,52.4105058599551));
#8805=CARTESIAN_POINT('Ctrl Pts',(-0.219393094396066,-4.07910427301526,
52.4165006146596));
#8806=CARTESIAN_POINT('Ctrl Pts',(-0.100057133964627,-4.08552271291761,
52.4223077713019));
#8807=CARTESIAN_POINT('Ctrl Pts',(0.0196136949359783,-4.08670282490637,
52.4281149279442));
#8808=CARTESIAN_POINT('Ctrl Pts',(0.139125575425362,-4.08263016623629,52.4339220845864));
#8809=CARTESIAN_POINT('Ctrl Pts',(0.258620354455936,-4.07855809034011,52.4397284102581));
#8810=CARTESIAN_POINT('Ctrl Pts',(0.377955822841558,-4.06923475253925,52.4455347359299));
#8811=CARTESIAN_POINT('Ctrl Pts',(0.496639238214287,-4.05469782685047,52.4513410616016));
#8812=CARTESIAN_POINT('Ctrl Pts',(0.615333590380842,-4.04015956156965,52.457147922332));
#8813=CARTESIAN_POINT('Ctrl Pts',(0.733375365265743,-4.02040680275784,52.4629547830624));
#8814=CARTESIAN_POINT('Ctrl Pts',(0.850278642547521,-3.99552890491704,52.4687616437927));
#8815=CARTESIAN_POINT('Ctrl Pts',(0.967220193279139,-3.97064286219786,52.4745704056554));
#8816=CARTESIAN_POINT('Ctrl Pts',(1.08302210643856,-3.94062842817693,52.480379167518));
#8817=CARTESIAN_POINT('Ctrl Pts',(1.19721094421841,-3.90562555233392,52.4861879293807));
#8818=CARTESIAN_POINT('Ctrl Pts',(1.31152526834388,-3.87058421053346,52.492003074707));
#8819=CARTESIAN_POINT('Ctrl Pts',(1.42422258870311,-3.8305436043431,52.4978182200333));
#8820=CARTESIAN_POINT('Ctrl Pts',(1.53484672242706,-3.78569287431705,52.5036333653596));
#8821=CARTESIAN_POINT('Ctrl Pts',(1.64554371644493,-3.74081260428683,52.509452340711));
#8822=CARTESIAN_POINT('Ctrl Pts',(1.75416443444624,-3.69111607020024,52.5152713160623));
#8823=CARTESIAN_POINT('Ctrl Pts',(1.86027617340527,-3.63683895143305,52.5210902914136));
#8824=CARTESIAN_POINT('Ctrl Pts',(1.96653723173567,-3.58248545445046,52.5269174551685));
#8825=CARTESIAN_POINT('Ctrl Pts',(2.07028191132472,-3.52353870894868,52.5327446189234));
#8826=CARTESIAN_POINT('Ctrl Pts',(2.17110532330159,-3.4602784100606,52.5385717826783));
#8827=CARTESIAN_POINT('Ctrl Pts',(2.19312932682573,-3.44645974415422,52.5398446762707));
#8828=CARTESIAN_POINT('Ctrl Pts',(2.21501406010772,-3.43243540469784,52.5411175698632));
#8829=CARTESIAN_POINT('Ctrl Pts',(2.23675551426093,-3.41820856142853,52.5423904634556));
#8830=CARTESIAN_POINT('Ctrl Pts',(2.33627651339756,-3.35308551828965,52.5482171041771));
#8831=CARTESIAN_POINT('Ctrl Pts',(2.43310945763141,-3.28350890485543,52.5540437448986));
#8832=CARTESIAN_POINT('Ctrl Pts',(2.52683075548952,-3.20972761042308,52.5598703856202));
#8833=CARTESIAN_POINT('Ctrl Pts',(2.6204348071879,-3.13603861703254,52.5656897371634));
#8834=CARTESIAN_POINT('Ctrl Pts',(2.71093463758183,-3.05815565528383,52.5715090887067));
#8835=CARTESIAN_POINT('Ctrl Pts',(2.79793451014694,-2.97637152871223,52.5773284402499));
#8836=CARTESIAN_POINT('Ctrl Pts',(2.88484814764639,-2.89466846731139,52.5831420235989));
#8837=CARTESIAN_POINT('Ctrl Pts',(2.96826843360688,-2.80907221176675,52.5889556069479));
#8838=CARTESIAN_POINT('Ctrl Pts',(3.04783216983345,-2.71991618704112,52.594769190297));
#8839=CARTESIAN_POINT('Ctrl Pts',(3.12987541154458,-2.62798172501764,52.6007639467844));
#8840=CARTESIAN_POINT('Ctrl Pts',(3.20781744996931,-2.53226226087349,52.6067587032719));
#8841=CARTESIAN_POINT('Ctrl Pts',(3.28130032850117,-2.43316525418601,52.6127534597594));
#8842=CARTESIAN_POINT('Ctrl Pts',(3.35248357540003,-2.33716946802593,52.6185606115704));
#8843=CARTESIAN_POINT('Ctrl Pts',(3.41948233654224,-2.23800473731128,52.6243677633814));
#8844=CARTESIAN_POINT('Ctrl Pts',(3.482012159524,-2.13607498017439,52.6301749151925));
#8845=CARTESIAN_POINT('Ctrl Pts',(3.54453303475801,-2.03415980874575,52.6359812360251));
#8846=CARTESIAN_POINT('Ctrl Pts',(3.6025860304528,-1.92948074531676,52.6417875568578));
#8847=CARTESIAN_POINT('Ctrl Pts',(3.65593075681061,-1.82246956117411,52.6475938776905));
#8848=CARTESIAN_POINT('Ctrl Pts',(3.70928039891937,-1.71544851588181,52.6534007335794));
#8849=CARTESIAN_POINT('Ctrl Pts',(3.75792072710644,-1.60609528758058,52.6592075894682));
#8850=CARTESIAN_POINT('Ctrl Pts',(3.80165822082893,-1.49486446609844,52.6650144453571));
#8851=CARTESIAN_POINT('Ctrl Pts',(3.84541003398569,-1.38359722820785,52.6708232023813));
#8852=CARTESIAN_POINT('Ctrl Pts',(3.88425567115322,-1.27045155390415,52.6766319594054));
#8853=CARTESIAN_POINT('Ctrl Pts',(3.91805069814696,-1.1558995314257,52.6824407164295));
#8854=CARTESIAN_POINT('Ctrl Pts',(3.95188286394642,-1.04122162281288,52.6882558569461));
#8855=CARTESIAN_POINT('Ctrl Pts',(3.98065322554323,-0.925134672530824,52.6940709974626));
#8856=CARTESIAN_POINT('Ctrl Pts',(4.00426789676726,-0.808123512168205,52.6998861379792));
#8857=CARTESIAN_POINT('Ctrl Pts',(4.02789812136444,-0.691035284535784,52.7057051085322));
#8858=CARTESIAN_POINT('Ctrl Pts',(4.04636582989237,-0.57302203647665,52.7115240790851));
#8859=CARTESIAN_POINT('Ctrl Pts',(4.05962890585733,-0.454574687733093,52.7173430496381));
#8860=CARTESIAN_POINT('Ctrl Pts',(4.07291064562427,-0.335960659867111,52.723170208647));
#8861=CARTESIAN_POINT('Ctrl Pts',(4.08097310808659,-0.216911717493788,52.728997367656));
#8862=CARTESIAN_POINT('Ctrl Pts',(4.08382623292447,-0.0979198615089626,
52.734824526665));
#8863=CARTESIAN_POINT('Ctrl Pts',(4.08444949652334,-0.0719261540439095,
52.736097466442));
#8864=CARTESIAN_POINT('Ctrl Pts',(4.08482436641676,-0.0459351536481145,
52.7373704062191));
#8865=CARTESIAN_POINT('Ctrl Pts',(4.08495127505391,-0.0199519531724785,
52.7386433459962));
#8866=CARTESIAN_POINT('Ctrl Pts',(4.08553217514419,0.0989811930683613,52.7444699851281));
#8867=CARTESIAN_POINT('Ctrl Pts',(4.08091559422358,0.218129010432613,52.75029662426));
#8868=CARTESIAN_POINT('Ctrl Pts',(4.0710754597632,0.337000891562378,52.7561232633919));
#8869=CARTESIAN_POINT('Ctrl Pts',(4.06124763546442,0.455724062115895,52.7619426133074));
#8870=CARTESIAN_POINT('Ctrl Pts',(4.04620928887724,0.574171580131339,52.7677619632229));
#8871=CARTESIAN_POINT('Ctrl Pts',(4.02598634147149,0.691851847063394,52.7735813131384));
#8872=CARTESIAN_POINT('Ctrl Pts',(4.00578343936559,0.809415467485428,52.7793948948238));
#8873=CARTESIAN_POINT('Ctrl Pts',(3.98040622898983,0.926212950150694,52.7852084765092));
#8874=CARTESIAN_POINT('Ctrl Pts',(3.94993246284014,1.04175742810004,52.7910220581946));
#8875=CARTESIAN_POINT('Ctrl Pts',(3.91850900724911,1.16090275309187,52.7970168152922));
#8876=CARTESIAN_POINT('Ctrl Pts',(3.88166616893103,1.27871525635869,52.8030115723898));
#8877=CARTESIAN_POINT('Ctrl Pts',(3.83954634323955,1.39467160224758,52.8090063294874));
#8878=CARTESIAN_POINT('Ctrl Pts',(3.7987446652614,1.50699907290559,52.814813479556));
#8879=CARTESIAN_POINT('Ctrl Pts',(3.75299151228405,1.61758441980801,52.8206206296246));
#8880=CARTESIAN_POINT('Ctrl Pts',(3.70246687307412,1.72596757031781,52.8264277796931));
#8881=CARTESIAN_POINT('Ctrl Pts',(3.65194946395254,1.834335211172,52.8322340987571));
#8882=CARTESIAN_POINT('Ctrl Pts',(3.59666209881831,1.94050091284881,52.8380404178211));
#8883=CARTESIAN_POINT('Ctrl Pts',(3.53683230480951,2.04402598996584,52.8438467368851));
#8884=CARTESIAN_POINT('Ctrl Pts',(3.47699699769631,2.14756060655342,52.8496535909809));
#8885=CARTESIAN_POINT('Ctrl Pts',(3.41261863355883,2.24845376169357,52.8554604450767));
#8886=CARTESIAN_POINT('Ctrl Pts',(3.34396962684773,2.3462932755135,52.8612672991724));
#8887=CARTESIAN_POINT('Ctrl Pts',(3.2752981450587,2.44416482112533,52.8670760543809));
#8888=CARTESIAN_POINT('Ctrl Pts',(3.20235347410291,2.53898040347634,52.8728848095894));
#8889=CARTESIAN_POINT('Ctrl Pts',(3.12544970132398,2.63035913222773,52.8786935647979));
#8890=CARTESIAN_POINT('Ctrl Pts',(3.04846141598508,2.72183828063364,52.8845087034744));
#8891=CARTESIAN_POINT('Ctrl Pts',(2.96750560724484,2.80987272450696,52.8903238421509));
#8892=CARTESIAN_POINT('Ctrl Pts',(2.88293487550622,2.89411670524703,52.8961389808274));
#8893=CARTESIAN_POINT('Ctrl Pts',(2.79830844301607,2.97841617153089,52.9019579495239));
#8894=CARTESIAN_POINT('Ctrl Pts',(2.71006264636445,3.05891992849812,52.9077769182204));
#8895=CARTESIAN_POINT('Ctrl Pts',(2.61858372191455,3.13532203949198,52.9135958869169));
#8896=CARTESIAN_POINT('Ctrl Pts',(2.52697606842891,3.21183166344728,52.9194230440593));
#8897=CARTESIAN_POINT('Ctrl Pts',(2.4321265298229,3.28422787539933,52.9252502012018));
#8898=CARTESIAN_POINT('Ctrl Pts',(2.33445096018978,3.3522475616322,52.9310773583442));
#8899=CARTESIAN_POINT('Ctrl Pts',(2.3131134930913,3.36710662846431,52.9323503150751));
#8900=CARTESIAN_POINT('Ctrl Pts',(2.29164125791616,3.38175701461162,52.933623271806));
#8901=CARTESIAN_POINT('Ctrl Pts',(2.27003874127722,3.39619627128653,52.9348962285368));
#8902=CARTESIAN_POINT('Ctrl Pts',(2.17115862198715,3.46228835890476,52.9407228697334));
#8903=CARTESIAN_POINT('Ctrl Pts',(2.06923234116559,3.52416371376206,52.94654951093));
#8904=CARTESIAN_POINT('Ctrl Pts',(1.96465472573961,3.58152995361326,52.9523761521266));
#8905=CARTESIAN_POINT('Ctrl Pts',(1.86020793795112,3.63882442772759,52.958195504137));
#8906=CARTESIAN_POINT('Ctrl Pts',(1.75311676738121,3.69162081248238,52.9640148561475));
#8907=CARTESIAN_POINT('Ctrl Pts',(1.64380554930374,3.73966954637415,52.969834208158));
#8908=CARTESIAN_POINT('Ctrl Pts',(1.53460268164954,3.78767065385807,52.9756477919658));
#8909=CARTESIAN_POINT('Ctrl Pts',(1.42318451557263,3.83093330946312,52.9814613757737));
#8910=CARTESIAN_POINT('Ctrl Pts',(1.31000003150605,3.86925379336302,52.9872749595816));
#8911=CARTESIAN_POINT('Ctrl Pts',(1.19328830553101,3.90876848349958,52.9932697158939));
#8912=CARTESIAN_POINT('Ctrl Pts',(1.07469875546949,3.94302771155996,52.9992644722062));
#8913=CARTESIAN_POINT('Ctrl Pts',(0.954746438207526,3.97186155835397,53.0052592285186));
#8914=CARTESIAN_POINT('Ctrl Pts',(0.838547992052256,3.99979305872529,53.0110663807643));
#8915=CARTESIAN_POINT('Ctrl Pts',(0.721071227025833,4.02263358284084,53.0168735330101));
#8916=CARTESIAN_POINT('Ctrl Pts',(0.602799171696235,4.04027946540859,53.0226806852558));
#8917=CARTESIAN_POINT('Ctrl Pts',(0.484544040784918,4.05792282289722,53.0284870065135));
#8918=CARTESIAN_POINT('Ctrl Pts',(0.365494249146629,4.07037295703365,53.0342933277711));
#8919=CARTESIAN_POINT('Ctrl Pts',(0.246141210279892,4.07757765157231,53.0400996490288));
#8920=CARTESIAN_POINT('Ctrl Pts',(0.126777173166066,4.08478301001539,53.0459065053323));
#8921=CARTESIAN_POINT('Ctrl Pts',(0.00711024035019893,4.08674194324849,
53.0517133616359));
#8922=CARTESIAN_POINT('Ctrl Pts',(-0.112365521214941,4.08345429625974,53.0575202179394));
#8923=CARTESIAN_POINT('Ctrl Pts',(-0.231880398314553,4.08016557291819,53.0633289753674));
#8924=CARTESIAN_POINT('Ctrl Pts',(-0.351203572249954,4.0716268643931,53.0691377327954));
#8925=CARTESIAN_POINT('Ctrl Pts',(-0.469844086081757,4.05789003483017,53.0749464902233));
#8926=CARTESIAN_POINT('Ctrl Pts',(-0.588614978687084,4.04413810931955,53.0807616311256));
#8927=CARTESIAN_POINT('Ctrl Pts',(-0.706701308455423,4.02517670759286,53.0865767720278));
#8928=CARTESIAN_POINT('Ctrl Pts',(-0.823620176257923,4.0011091968679,53.0923919129301));
#8929=CARTESIAN_POINT('Ctrl Pts',(-0.940616050333473,3.97702583455852,53.0982108838586));
#8930=CARTESIAN_POINT('Ctrl Pts',(-1.05644253656456,3.94782976495233,53.104029854787));
#8931=CARTESIAN_POINT('Ctrl Pts',(-1.17063139603742,3.9136743776931,53.1098488257155));
#8932=CARTESIAN_POINT('Ctrl Pts',(-1.28498094172898,3.87947092707592,53.1156759850823));
#8933=CARTESIAN_POINT('Ctrl Pts',(-1.39768787761184,3.840294363912,53.1215031444491));
#8934=CARTESIAN_POINT('Ctrl Pts',(-1.5083033446677,3.79634640417129,53.1273303038159));
#8935=CARTESIAN_POINT('Ctrl Pts',(-1.53246715658383,3.78674602674182,53.1286032395698));
#8936=CARTESIAN_POINT('Ctrl Pts',(-1.55653125664943,3.77691813330193,53.1298761753236));
#8937=CARTESIAN_POINT('Ctrl Pts',(-1.58049112762186,3.76686511512008,53.1311491110775));
#8938=CARTESIAN_POINT('Ctrl Pts',(-1.69016324034444,3.72084918521332,53.1369757515317));
#8939=CARTESIAN_POINT('Ctrl Pts',(-1.79799860007571,3.66996640222913,53.1428023919859));
#8940=CARTESIAN_POINT('Ctrl Pts',(-1.90353553495269,3.61438479788364,53.1486290324401));
#8941=CARTESIAN_POINT('Ctrl Pts',(-2.00894044192748,3.55887272675542,53.154448383701));
#8942=CARTESIAN_POINT('Ctrl Pts',(-2.11205228553337,3.49867371481663,53.160267734962));
#8943=CARTESIAN_POINT('Ctrl Pts',(-2.21242883229364,3.43400402766738,53.1660870862229));
#8944=CARTESIAN_POINT('Ctrl Pts',(-2.31270588465065,3.36939844186591,53.171900669275));
#8945=CARTESIAN_POINT('Ctrl Pts',(-2.4102526931584,3.30033121648047,53.1777142523271));
#8946=CARTESIAN_POINT('Ctrl Pts',(-2.5046516651484,3.22706446112707,53.1835278353793));
#8947=CARTESIAN_POINT('Ctrl Pts',(-2.60199247109591,3.15151443272195,53.1895225919725));
#8948=CARTESIAN_POINT('Ctrl Pts',(-2.69598563869675,3.07149904554205,53.1955173485658));
#8949=CARTESIAN_POINT('Ctrl Pts',(-2.78620531770213,2.98735416842536,53.2015121051591));
#8950=CARTESIAN_POINT('Ctrl Pts',(-2.87360158380063,2.90584259409493,53.2073192566387));
#8951=CARTESIAN_POINT('Ctrl Pts',(-2.95745670070888,2.82045643756548,53.2131264081182));
#8952=CARTESIAN_POINT('Ctrl Pts',(-3.0374177477781,2.73154140101932,53.2189335595978));
#8953=CARTESIAN_POINT('Ctrl Pts',(-3.11736735259683,2.64263908801991,53.2247398800868));
#8954=CARTESIAN_POINT('Ctrl Pts',(-3.1934237231818,2.55020920245243,53.2305462005757));
#8955=CARTESIAN_POINT('Ctrl Pts',(-3.26527222642084,2.45463282129216,53.2363525210646));
#8956=CARTESIAN_POINT('Ctrl Pts',(-3.3371273503981,2.35904763290318,53.2421593765978));
#8957=CARTESIAN_POINT('Ctrl Pts',(-3.40477359103225,2.26031569842973,53.2479662321309));
#8958=CARTESIAN_POINT('Ctrl Pts',(-3.46793827504224,2.15884902679577,53.2537730876641));
#8959=CARTESIAN_POINT('Ctrl Pts',(-3.53112363872488,2.05734913568818,53.2595818443209));
#8960=CARTESIAN_POINT('Ctrl Pts',(-3.58982431233119,1.95311307279088,53.2653906009777));
#8961=CARTESIAN_POINT('Ctrl Pts',(-3.64381272664073,1.84657894853457,53.2711993576344));
#8962=CARTESIAN_POINT('Ctrl Pts',(-3.69786047099602,1.73992774963277,53.2770144977681));
#8963=CARTESIAN_POINT('Ctrl Pts',(-3.74718543523956,1.63097381251409,53.2828296379019));
#8964=CARTESIAN_POINT('Ctrl Pts',(-3.79160745312437,1.52017693753448,53.2886447780356));
#8965=CARTESIAN_POINT('Ctrl Pts',(-3.83605872869159,1.40930708838725,53.2944637481962));
#8966=CARTESIAN_POINT('Ctrl Pts',(-3.87560049196883,1.29659226788354,53.3002827183568));
#8967=CARTESIAN_POINT('Ctrl Pts',(-3.91010238680603,1.18250764255196,53.3061016885174));
#8968=CARTESIAN_POINT('Ctrl Pts',(-3.94465283265201,1.0682624775262,53.3119288471231));
#8969=CARTESIAN_POINT('Ctrl Pts',(-3.97414915509558,0.952644054234602,53.3177560057288));
#8970=CARTESIAN_POINT('Ctrl Pts',(-3.99851199692488,0.836138033130776,53.3235831643345));
#8971=CARTESIAN_POINT('Ctrl Pts',(-4.00383406096464,0.810687286880546,53.324856107429));
#8972=CARTESIAN_POINT('Ctrl Pts',(-4.00891134974107,0.785194202913159,53.3261290505236));
#8973=CARTESIAN_POINT('Ctrl Pts',(-4.013743365907,0.759663868192736,53.3274019936181));
#8974=CARTESIAN_POINT('Ctrl Pts',(-4.0458370446992,0.590094410261053,53.3358567308113));
#8975=CARTESIAN_POINT('Ctrl Pts',(-4.06719182948094,0.418433988893306,53.3443114680044));
#8976=CARTESIAN_POINT('Ctrl Pts',(-4.07759833749446,0.245798287346335,53.3527662051976));
#8977=CARTESIAN_POINT('Ctrl Pts',(-4.08245970979669,0.165151982477693,53.3567158129969));
#8978=CARTESIAN_POINT('Ctrl Pts',(-4.08493248888153,0.0842931598013199,
53.3606654207962));
#8979=CARTESIAN_POINT('Ctrl Pts',(-4.08499863636774,0.00333779473110509,
53.3646150285955));
#8980=CARTESIAN_POINT('Ctrl Pts',(-4.08499863636843,0.00333779389426807,
53.3646150286363));
#8981=CARTESIAN_POINT('Ctrl Pts',(-4.0850946608337,-0.114182886570259,53.3703485658236));
#8982=CARTESIAN_POINT('Ctrl Pts',(-4.08011509051747,-0.231867440180717,
53.3760821030108));
#8983=CARTESIAN_POINT('Ctrl Pts',(-4.07004418083968,-0.349235402004226,
53.381815640198));
#8984=CARTESIAN_POINT('Ctrl Pts',(-4.0596633716385,-0.470214981506232,53.3877256083631));
#8985=CARTESIAN_POINT('Ctrl Pts',(-4.04387275277963,-0.590857721096756,
53.3936355765281));
#8986=CARTESIAN_POINT('Ctrl Pts',(-4.0227131092999,-0.710636503612598,53.3995455446931));
#8987=CARTESIAN_POINT('Ctrl Pts',(-4.00221473529391,-0.826672025871896,
53.4052708178021));
#8988=CARTESIAN_POINT('Ctrl Pts',(-3.97667799340902,-0.941896338091274,
53.4109960909111));
#8989=CARTESIAN_POINT('Ctrl Pts',(-3.94619255154103,-1.05583585190221,53.4167213640201));
#8990=CARTESIAN_POINT('Ctrl Pts',(-3.91571465964673,-1.16974714764318,53.4224452192175));
#8991=CARTESIAN_POINT('Ctrl Pts',(-3.8802906122784,-1.28237387106175,53.4281690744149));
#8992=CARTESIAN_POINT('Ctrl Pts',(-3.84006075202239,-1.39325461448268,53.4338929296123));
#8993=CARTESIAN_POINT('Ctrl Pts',(-3.79983072022201,-1.50413583071077,53.4396168092168));
#8994=CARTESIAN_POINT('Ctrl Pts',(-3.75479497912581,-1.61327065677188,53.4453406888213));
#8995=CARTESIAN_POINT('Ctrl Pts',(-3.7051428357764,-1.72021555814811,53.4510645684258));
#8996=CARTESIAN_POINT('Ctrl Pts',(-3.65547797106196,-1.82718785985465,53.4567899145443));
#8997=CARTESIAN_POINT('Ctrl Pts',(-3.60119453146051,-1.93196874060564,53.4625152606628));
#8998=CARTESIAN_POINT('Ctrl Pts',(-3.54252842342547,-2.03413799168657,53.4682406067813));
#8999=CARTESIAN_POINT('Ctrl Pts',(-3.4838014026026,-2.13641332469661,53.473971897504));
#9000=CARTESIAN_POINT('Ctrl Pts',(-3.42068284295228,-2.23607125209266,53.4797031882267));
#9001=CARTESIAN_POINT('Ctrl Pts',(-3.35345271933515,-2.33271941287068,53.4854344789494));
#9002=CARTESIAN_POINT('Ctrl Pts',(-3.28618056105595,-2.42942800151284,53.4911693530787));
#9003=CARTESIAN_POINT('Ctrl Pts',(-3.2147919776946,-2.52312274512152,53.496904227208));
#9004=CARTESIAN_POINT('Ctrl Pts',(-3.13960694212807,-2.61344470937137,53.5026391013373));
#9005=CARTESIAN_POINT('Ctrl Pts',(-3.06431706707054,-2.70389262034303,53.5083819722878));
#9006=CARTESIAN_POINT('Ctrl Pts',(-2.98522046104977,-2.79095806015633,53.5141248432383));
#9007=CARTESIAN_POINT('Ctrl Pts',(-2.90267351731113,-2.87431930235676,53.5198677141888));
#9008=CARTESIAN_POINT('Ctrl Pts',(-2.8845282000555,-2.89264361720165,53.5211301015121));
#9009=CARTESIAN_POINT('Ctrl Pts',(-2.86621628596619,-2.91078910223333,53.5223924888354));
#9010=CARTESIAN_POINT('Ctrl Pts',(-2.84774176294681,-2.92875261016847,53.5236548761588));
#9011=CARTESIAN_POINT('Ctrl Pts',(-2.76248879875287,-3.01164743225319,53.5294803181018));
#9012=CARTESIAN_POINT('Ctrl Pts',(-2.67347771023089,-3.09094862859931,53.5353057600448));
#9013=CARTESIAN_POINT('Ctrl Pts',(-2.58104361116293,-3.16629734505068,53.5411312019878));
#9014=CARTESIAN_POINT('Ctrl Pts',(-2.49470736968296,-3.23667532292191,53.5465723407817));
#9015=CARTESIAN_POINT('Ctrl Pts',(-2.40538541417085,-3.3036051904254,53.5520134795756));
#9016=CARTESIAN_POINT('Ctrl Pts',(-2.31338095599001,-3.36682247118299,53.5574546183695));
#9017=CARTESIAN_POINT('',(-4.08499939840936,-0.00221697883968487,53.2603849714447));
#9018=CARTESIAN_POINT('Ctrl Pts',(-4.08499939840936,-0.00221697883967045,
53.2603849714447));
#9019=CARTESIAN_POINT('Ctrl Pts',(-4.08492707751238,-0.135475274033514,
53.2668482540158));
#9020=CARTESIAN_POINT('Ctrl Pts',(-4.07833004186189,-0.268506050828305,
53.2733115365868));
#9021=CARTESIAN_POINT('Ctrl Pts',(-4.06529953148975,-0.400705277316363,
53.2797748191579));
#9022=CARTESIAN_POINT('Ctrl Pts',(-4.05222537576177,-0.533347301677931,
53.2862597503259));
#9023=CARTESIAN_POINT('Ctrl Pts',(-4.03267468654002,-0.665151973365606,
53.2927446814939));
#9024=CARTESIAN_POINT('Ctrl Pts',(-4.00678976762601,-0.795525460338974,
53.299229612662));
#9025=CARTESIAN_POINT('Ctrl Pts',(-3.98078013150707,-0.926527105234957,
53.3057457891467));
#9026=CARTESIAN_POINT('Ctrl Pts',(-3.94837518576072,-1.05608352155153,53.3122619656315));
#9027=CARTESIAN_POINT('Ctrl Pts',(-3.90976823011133,-1.18361200856199,53.3187781421162));
#9028=CARTESIAN_POINT('Ctrl Pts',(-3.87516577533156,-1.29791262177236,53.3246184291411));
#9029=CARTESIAN_POINT('Ctrl Pts',(-3.83558190815159,-1.41058434768274,53.330458716166));
#9030=CARTESIAN_POINT('Ctrl Pts',(-3.79118783028315,-1.52122313797581,53.3362990031909));
#9031=CARTESIAN_POINT('Ctrl Pts',(-3.74690246501772,-1.6315909950394,53.3421249884703));
#9032=CARTESIAN_POINT('Ctrl Pts',(-3.69772314220471,-1.7401990447553,53.3479509737497));
#9033=CARTESIAN_POINT('Ctrl Pts',(-3.64381057578868,-1.84658319275643,53.353776959029));
#9034=CARTESIAN_POINT('Ctrl Pts',(-3.58996186347553,-1.95284133925584,53.3595960440051));
#9035=CARTESIAN_POINT('Ctrl Pts',(-3.53139123772933,-2.05688046120153,53.3654151289811));
#9036=CARTESIAN_POINT('Ctrl Pts',(-3.46830796704526,-2.15825504649714,53.3712342139571));
#9037=CARTESIAN_POINT('Ctrl Pts',(-3.40528456459923,-2.25953342375317,53.3770477764172));
#9038=CARTESIAN_POINT('Ctrl Pts',(-3.3377572495909,-2.35815194973833,53.3828613388773));
#9039=CARTESIAN_POINT('Ctrl Pts',(-3.26598154053163,-2.45368897313955,53.3886749013375));
#9040=CARTESIAN_POINT('Ctrl Pts',(-3.1942586231698,-2.54915572817701,53.3944841878687));
#9041=CARTESIAN_POINT('Ctrl Pts',(-3.11829377405021,-2.64154516592262,53.4002934743999));
#9042=CARTESIAN_POINT('Ctrl Pts',(-3.03838585205935,-2.73046450517225,53.4061027609311));
#9043=CARTESIAN_POINT('Ctrl Pts',(-2.9585130687976,-2.81934474300995,53.4119094928852));
#9044=CARTESIAN_POINT('Ctrl Pts',(-2.87470093510515,-2.90475761602359,53.4177162248393));
#9045=CARTESIAN_POINT('Ctrl Pts',(-2.78728827016216,-2.98634376772274,53.4235229567934));
#9046=CARTESIAN_POINT('Ctrl Pts',(-2.69987790237354,-3.06792777538491,53.42932953615));
#9047=CARTESIAN_POINT('Ctrl Pts',(-2.60886748387272,-3.14568497751308,53.4351361155066));
#9048=CARTESIAN_POINT('Ctrl Pts',(-2.51463206891315,-3.21929348739651,53.4409426948631));
#9049=CARTESIAN_POINT('Ctrl Pts',(-2.44906374430374,-3.27050975966657,53.4449828710568));
#9050=CARTESIAN_POINT('Ctrl Pts',(-2.38193487256495,-3.31971831691873,53.4490230472505));
#9051=CARTESIAN_POINT('Ctrl Pts',(-2.31338095599002,-3.36682247118299,53.4530632234442));
#9052=CARTESIAN_POINT('Ctrl Pts',(-2.31338095599002,-3.36682247118298,52.2032272635689));
#9053=CARTESIAN_POINT('Ctrl Pts',(-2.21500698803516,-3.43441631255116,52.209038374945));
#9054=CARTESIAN_POINT('Ctrl Pts',(-2.11358325818932,-3.49775331847722,52.2148494863211));
#9055=CARTESIAN_POINT('Ctrl Pts',(-2.0095158195868,-3.55655327119254,52.2206605976972));
#9056=CARTESIAN_POINT('Ctrl Pts',(-1.90550258339924,-3.61532259857991,52.2264686824179));
#9057=CARTESIAN_POINT('Ctrl Pts',(-1.79884873132084,-3.66955937251817,52.2322767671387));
#9058=CARTESIAN_POINT('Ctrl Pts',(-1.68998803059726,-3.71902748799172,52.2380848518594));
#9059=CARTESIAN_POINT('Ctrl Pts',(-1.58115537394738,-3.76848285977111,52.2438914403345));
#9060=CARTESIAN_POINT('Ctrl Pts',(-1.47011737018069,-3.8131718473842,52.2496980288095));
#9061=CARTESIAN_POINT('Ctrl Pts',(-1.35733050818773,-3.85290525338255,52.2555046172846));
#9062=CARTESIAN_POINT('Ctrl Pts',(-1.24454616975475,-3.89263777036216,52.2613110758396));
#9063=CARTESIAN_POINT('Ctrl Pts',(-1.13001343562466,-3.92741479094115,52.2671175343946));
#9064=CARTESIAN_POINT('Ctrl Pts',(-1.01420620174307,-3.95709625613857,52.2729239929496));
#9065=CARTESIAN_POINT('Ctrl Pts',(-0.898374316818721,-3.9867840394134,52.2787316874831));
#9066=CARTESIAN_POINT('Ctrl Pts',(-0.781267787618402,-4.01137400909616,
52.2845393820167));
#9067=CARTESIAN_POINT('Ctrl Pts',(-0.663372383682657,-4.03077685819585,
52.2903470765502));
#9068=CARTESIAN_POINT('Ctrl Pts',(-0.54535394965723,-4.05019995519482,52.2961608317202));
#9069=CARTESIAN_POINT('Ctrl Pts',(-0.426545399849018,-4.06442505521714,
52.3019745868902));
#9070=CARTESIAN_POINT('Ctrl Pts',(-0.307439577105467,-4.07341452671211,
52.3077883420602));
#9071=CARTESIAN_POINT('Ctrl Pts',(-0.188267544862691,-4.08240899534653,
52.313605329027));
#9072=CARTESIAN_POINT('Ctrl Pts',(-0.0687983178358109,-4.08616202451501,
52.3194223159937));
#9073=CARTESIAN_POINT('Ctrl Pts',(0.0504750103484449,-4.0846881488469,52.3252393029605));
#9074=CARTESIAN_POINT('Ctrl Pts',(0.169931934319669,-4.08321200446233,52.331065243935));
#9075=CARTESIAN_POINT('Ctrl Pts',(0.289191950067047,-4.07649290644593,52.3368911849095));
#9076=CARTESIAN_POINT('Ctrl Pts',(0.407766381997247,-4.06459734509002,52.3427171258841));
#9077=CARTESIAN_POINT('Ctrl Pts',(0.491331501897505,-4.05621396939254,52.3468229474186));
#9078=CARTESIAN_POINT('Ctrl Pts',(0.574556245414403,-4.04526069041347,52.3509287689531));
#9079=CARTESIAN_POINT('Ctrl Pts',(0.657273191228009,-4.0317759054904,52.3550345904877));
#9080=CARTESIAN_POINT('Ctrl Pts',(0.774658327852714,-4.01263939960301,52.3608612372171));
#9081=CARTESIAN_POINT('Ctrl Pts',(0.891393842455179,-3.98834168701438,52.3666878839465));
#9082=CARTESIAN_POINT('Ctrl Pts',(1.00699158944047,-3.95893836006525,52.3725145306759));
#9083=CARTESIAN_POINT('Ctrl Pts',(1.12244472614728,-3.92957181604148,52.3783338883963));
#9084=CARTESIAN_POINT('Ctrl Pts',(1.23676253446512,-3.89511246137051,52.3841532461168));
#9085=CARTESIAN_POINT('Ctrl Pts',(1.34946450787744,-3.85566732771113,52.3899726038373));
#9086=CARTESIAN_POINT('Ctrl Pts',(1.46205477330165,-3.81626129129547,52.3957861935245));
#9087=CARTESIAN_POINT('Ctrl Pts',(1.57303200732343,-3.77187944130429,52.4015997832116));
#9088=CARTESIAN_POINT('Ctrl Pts',(1.68192895912139,-3.7226791396075,52.4074133728987));
#9089=CARTESIAN_POINT('Ctrl Pts',(1.79421938401356,-3.67194564623474,52.4134081270708));
#9090=CARTESIAN_POINT('Ctrl Pts',(1.9042973225786,-3.61608858344617,52.4194028812429));
#9091=CARTESIAN_POINT('Ctrl Pts',(2.01167027494216,-3.55533510444713,52.4253976354149));
#9092=CARTESIAN_POINT('Ctrl Pts',(2.11568317291385,-3.49648280250842,52.4312047939249));
#9093=CARTESIAN_POINT('Ctrl Pts',(2.21715747509268,-3.43303618012524,52.437011952435));
#9094=CARTESIAN_POINT('Ctrl Pts',(2.31566929715199,-3.36524898131292,52.442819110945));
#9095=CARTESIAN_POINT('Ctrl Pts',(2.41416702468894,-3.29747148111512,52.4486254385991));
#9096=CARTESIAN_POINT('Ctrl Pts',(2.50970277920253,-3.22535487070371,52.4544317662533));
#9097=CARTESIAN_POINT('Ctrl Pts',(2.60188164598711,-3.14919623083024,52.4602380939075));
#9098=CARTESIAN_POINT('Ctrl Pts',(2.69406900893618,-3.07303057138326,52.4660449567332));
#9099=CARTESIAN_POINT('Ctrl Pts',(2.78289855458322,-2.99282240150259,52.471851819559));
#9100=CARTESIAN_POINT('Ctrl Pts',(2.86800894597763,-2.90890867608322,52.4776586823848));
#9101=CARTESIAN_POINT('Ctrl Pts',(2.95314720364018,-2.82496747620001,52.4834674464543));
#9102=CARTESIAN_POINT('Ctrl Pts',(3.03456359502749,-2.73731859401619,52.4892762105238));
#9103=CARTESIAN_POINT('Ctrl Pts',(3.11193454611108,-2.64633489579842,52.4950849745933));
#9104=CARTESIAN_POINT('Ctrl Pts',(3.18939052502715,-2.55525120983922,52.5009001222811));
#9105=CARTESIAN_POINT('Ctrl Pts',(3.26279192542986,-2.46082570358057,52.5067152699689));
#9106=CARTESIAN_POINT('Ctrl Pts',(3.33185620162636,-2.3634634018076,52.5125304176567));
#9107=CARTESIAN_POINT('Ctrl Pts',(3.40096596666728,-2.26603697283543,52.5183493954628));
#9108=CARTESIAN_POINT('Ctrl Pts',(3.46573269772204,-2.16567023788159,52.5241683732689));
#9109=CARTESIAN_POINT('Ctrl Pts',(3.52591869455345,-2.06279479333221,52.529987351075));
#9110=CARTESIAN_POINT('Ctrl Pts',(3.58618938569597,-1.95977458147208,52.5358145174024));
#9111=CARTESIAN_POINT('Ctrl Pts',(3.6418662878908,-1.85423897356204,52.5416416837298));
#9112=CARTESIAN_POINT('Ctrl Pts',(3.69275883995195,-1.74664167760784,52.5474688500572));
#9113=CARTESIAN_POINT('Ctrl Pts',(3.70387570519099,-1.72313834380428,52.5487417243809));
#9114=CARTESIAN_POINT('Ctrl Pts',(3.71476447124475,-1.69953670046962,52.5500145987046));
#9115=CARTESIAN_POINT('Ctrl Pts',(3.72542346702583,-1.67584157703921,52.5512874730283));
#9116=CARTESIAN_POINT('Ctrl Pts',(3.77421541008635,-1.56737628284319,52.5571141018029));
#9117=CARTESIAN_POINT('Ctrl Pts',(3.81834414749158,-1.45660573581094,52.5629407305775));
#9118=CARTESIAN_POINT('Ctrl Pts',(3.85758676850764,-1.34396775386718,52.568767359352));
#9119=CARTESIAN_POINT('Ctrl Pts',(3.89678029524987,-1.231470687076,52.5745866987534));
#9120=CARTESIAN_POINT('Ctrl Pts',(3.93109973111366,-1.11711121406019,52.5804060381548));
#9121=CARTESIAN_POINT('Ctrl Pts',(3.96036928397369,-1.00134915716634,52.5862253775562));
#9122=CARTESIAN_POINT('Ctrl Pts',(3.98960982362738,-0.885701848470356,52.5920389485848));
#9123=CARTESIAN_POINT('Ctrl Pts',(4.01381033934235,-0.768655114975705,52.5978525196133));
#9124=CARTESIAN_POINT('Ctrl Pts',(4.03284433088837,-0.650685486868673,52.6036660906418));
#9125=CARTESIAN_POINT('Ctrl Pts',(4.05247154974745,-0.529039130980441,52.6096608516805));
#9126=CARTESIAN_POINT('Ctrl Pts',(4.06660477596062,-0.406411827768004,52.6156556127191));
#9127=CARTESIAN_POINT('Ctrl Pts',(4.075161791792,-0.283339673746216,52.6216503737577));
#9128=CARTESIAN_POINT('Ctrl Pts',(4.08345099316412,-0.164119388533449,52.6274575128826));
#9129=CARTESIAN_POINT('Ctrl Pts',(4.08650779254272,-0.0444821194083759,
52.6332646520076));
#9130=CARTESIAN_POINT('Ctrl Pts',(4.08431000327408,0.0750786065086086,52.6390717911325));
#9131=CARTESIAN_POINT('Ctrl Pts',(4.08211252854322,0.194622221428443,52.6448780991656));
#9132=CARTESIAN_POINT('Ctrl Pts',(4.07466196826704,0.314088907287876,52.6506844071987));
#9133=CARTESIAN_POINT('Ctrl Pts',(4.06198826299498,0.432985393854173,52.6564907152318));
#9134=CARTESIAN_POINT('Ctrl Pts',(4.04931339004772,0.55189283479214,52.6622975582215));
#9135=CARTESIAN_POINT('Ctrl Pts',(4.03141445853581,0.670229566454351,52.6681044012111));
#9136=CARTESIAN_POINT('Ctrl Pts',(4.00837319014032,0.787508329203119,52.6739112442008));
#9137=CARTESIAN_POINT('Ctrl Pts',(3.98532437847418,0.904825486776082,52.6797199882398));
#9138=CARTESIAN_POINT('Ctrl Pts',(3.95712996032764,1.02108358664462,52.6855287322788));
#9139=CARTESIAN_POINT('Ctrl Pts',(3.92392244191665,1.13580705660022,52.6913374763179));
#9140=CARTESIAN_POINT('Ctrl Pts',(3.89067843061372,1.25065660014977,52.6971526037869));
#9141=CARTESIAN_POINT('Ctrl Pts',(3.8524104362825,1.36396775564721,52.7029677312558));
#9142=CARTESIAN_POINT('Ctrl Pts',(3.80930042078689,1.47528143219958,52.7087828587248));
#9143=CARTESIAN_POINT('Ctrl Pts',(3.76616201198175,1.58666842265907,52.7146018161789));
#9144=CARTESIAN_POINT('Ctrl Pts',(3.7181753941769,1.69605494150659,52.7204207736329));
#9145=CARTESIAN_POINT('Ctrl Pts',(3.66556943056963,1.80300464493951,52.7262397310869));
#9146=CARTESIAN_POINT('Ctrl Pts',(3.61288943947137,1.91010484876563,52.7320668770198));
#9147=CARTESIAN_POINT('Ctrl Pts',(3.55557732414915,2.01476103695856,52.7378940229527));
#9148=CARTESIAN_POINT('Ctrl Pts',(3.49390639434769,2.11656398616633,52.7437211688856));
#9149=CARTESIAN_POINT('Ctrl Pts',(3.48043308645596,2.13880497529003,52.7449942311134));
#9150=CARTESIAN_POINT('Ctrl Pts',(3.46675189086912,2.16090990094908,52.7462672933412));
#9151=CARTESIAN_POINT('Ctrl Pts',(3.45286591532056,2.18287470341692,52.747540355569));
#9152=CARTESIAN_POINT('Ctrl Pts',(3.38931155483806,2.28340483679403,52.7533670009825));
#9153=CARTESIAN_POINT('Ctrl Pts',(3.32126201023034,2.38131708177875,52.7591936463961));
#9154=CARTESIAN_POINT('Ctrl Pts',(3.24895949813556,2.4761839954807,52.7650202918096));
#9155=CARTESIAN_POINT('Ctrl Pts',(3.17674743658946,2.57093223053445,52.7708396480812));
#9156=CARTESIAN_POINT('Ctrl Pts',(3.10029323527421,2.66264239043829,52.7766590043528));
#9157=CARTESIAN_POINT('Ctrl Pts',(3.01988345646099,2.75091419520734,52.7824783606244));
#9158=CARTESIAN_POINT('Ctrl Pts',(2.93955338007064,2.83909850468893,52.7882919487319));
#9159=CARTESIAN_POINT('Ctrl Pts',(2.85527579944563,2.92385093948815,52.7941055368394));
#9160=CARTESIAN_POINT('Ctrl Pts',(2.76737840353038,3.00480311695686,52.799919124947));
#9161=CARTESIAN_POINT('Ctrl Pts',(2.67674189491262,3.08827797596,52.8059138796621));
#9162=CARTESIAN_POINT('Ctrl Pts',(2.5822565373443,3.16771149489399,52.8119086343772));
#9163=CARTESIAN_POINT('Ctrl Pts',(2.48432412614819,3.24273937223423,52.8179033890923));
#9164=CARTESIAN_POINT('Ctrl Pts',(2.389456383202,3.31541934911195,52.8237105457057));
#9165=CARTESIAN_POINT('Ctrl Pts',(2.29135445900398,3.38396504402743,52.829517702319));
#9166=CARTESIAN_POINT('Ctrl Pts',(2.19041776181656,3.44808570495551,52.8353248589324));
#9167=CARTESIAN_POINT('Ctrl Pts',(2.08949550808893,3.51219719058646,52.8411311845751));
#9168=CARTESIAN_POINT('Ctrl Pts',(1.98573963224814,3.57188468292064,52.8469375102178));
#9169=CARTESIAN_POINT('Ctrl Pts',(1.87957808327149,3.62690105033008,52.8527438358605));
#9170=CARTESIAN_POINT('Ctrl Pts',(1.77340675140529,3.68192248755107,52.8585506965617));
#9171=CARTESIAN_POINT('Ctrl Pts',(1.66482966773145,3.73227175636399,52.8643575572629));
#9172=CARTESIAN_POINT('Ctrl Pts',(1.55429833197111,3.77774823078932,52.8701644179642));
#9173=CARTESIAN_POINT('Ctrl Pts',(1.44373080889862,3.8232395939461,52.8759731797976));
#9174=CARTESIAN_POINT('Ctrl Pts',(1.33120813820938,3.86385483482828,52.881781941631));
#9175=CARTESIAN_POINT('Ctrl Pts',(1.21720008567028,3.8994421333627,52.8875907034644));
#9176=CARTESIAN_POINT('Ctrl Pts',(1.10306674545585,3.93506854009874,52.8934058487616));
#9177=CARTESIAN_POINT('Ctrl Pts',(0.987445154693642,3.96565585411625,52.8992209940587));
#9178=CARTESIAN_POINT('Ctrl Pts',(0.870818613648606,3.99110259729352,52.9050361393558));
#9179=CARTESIAN_POINT('Ctrl Pts',(0.754115258948155,4.01656610044108,52.910855114678));
#9180=CARTESIAN_POINT('Ctrl Pts',(0.636406036678969,4.03688222061418,52.9166740900001));
#9181=CARTESIAN_POINT('Ctrl Pts',(0.518181146399915,4.05200114752151,52.9224930653222));
#9182=CARTESIAN_POINT('Ctrl Pts',(0.399789891239966,4.06714134963129,52.9283202290481));
#9183=CARTESIAN_POINT('Ctrl Pts',(0.280881924693484,4.07706972837865,52.934147392774));
#9184=CARTESIAN_POINT('Ctrl Pts',(0.161949343723945,4.08178850628831,52.9399745564999));
#9185=CARTESIAN_POINT('Ctrl Pts',(0.135969542851364,4.08281928279594,52.9412474503698));
#9186=CARTESIAN_POINT('Ctrl Pts',(0.109988553447076,4.08360167160106,52.9425203442398));
#9187=CARTESIAN_POINT('Ctrl Pts',(0.0840114739612687,4.08413602518854,52.9437932381097));
#9188=CARTESIAN_POINT('Ctrl Pts',(-0.034897975426568,4.08658201573572,52.9496198788329));
#9189=CARTESIAN_POINT('Ctrl Pts',(-0.15410357739852,4.08383452756355,52.9554465195561));
#9190=CARTESIAN_POINT('Ctrl Pts',(-0.273115193520258,4.07585979776886,52.9612731602793));
#9191=CARTESIAN_POINT('Ctrl Pts',(-0.391977925072666,4.06789504443067,52.9670925118242));
#9192=CARTESIAN_POINT('Ctrl Pts',(-0.510646750076163,4.05471608350436,52.972911863369));
#9193=CARTESIAN_POINT('Ctrl Pts',(-0.628629723682521,4.0363411241498,52.9787312149139));
#9194=CARTESIAN_POINT('Ctrl Pts',(-0.746495751490381,4.01798437822238,52.9845447982645));
#9195=CARTESIAN_POINT('Ctrl Pts',(-0.863676879673685,3.99444194254858,52.9903583816151));
#9196=CARTESIAN_POINT('Ctrl Pts',(-0.979685081592328,3.96578392514083,52.9961719649657));
#9197=CARTESIAN_POINT('Ctrl Pts',(-1.09930853567253,3.93623281605797,53.0021667214525));
#9198=CARTESIAN_POINT('Ctrl Pts',(-1.21768431984795,3.90124209033029,53.0081614779394));
#9199=CARTESIAN_POINT('Ctrl Pts',(-1.3342869301514,3.86094591881668,53.0141562344262));
#9200=CARTESIAN_POINT('Ctrl Pts',(-1.44724048568803,3.82191080772327,53.0199633862387));
#9201=CARTESIAN_POINT('Ctrl Pts',(-1.55852978083371,3.77789750739931,53.0257705380513));
#9202=CARTESIAN_POINT('Ctrl Pts',(-1.66769197672091,3.72907876972058,53.0315776898638));
#9203=CARTESIAN_POINT('Ctrl Pts',(-1.77683855196805,3.68026701779293,53.0373840106979));
#9204=CARTESIAN_POINT('Ctrl Pts',(-1.88385826112438,3.62665136253305,53.0431903315319));
#9205=CARTESIAN_POINT('Ctrl Pts',(-1.98830890445525,3.56845242373553,53.048996652366));
#9206=CARTESIAN_POINT('Ctrl Pts',(-2.09276917297909,3.51024812186892,53.0548035082563));
#9207=CARTESIAN_POINT('Ctrl Pts',(-2.19465954872222,3.44745989522938,53.0606103641465));
#9208=CARTESIAN_POINT('Ctrl Pts',(-2.29356363027887,3.380353661063,53.0664172200368));
#9209=CARTESIAN_POINT('Ctrl Pts',(-2.39250009253079,3.3132254566555,53.0722259770622));
#9210=CARTESIAN_POINT('Ctrl Pts',(-2.48844797885417,3.24177666199389,53.0780347340876));
#9211=CARTESIAN_POINT('Ctrl Pts',(-2.58102152001363,3.16631535277625,53.0838434911131));
#9212=CARTESIAN_POINT('Ctrl Pts',(-2.67369679420993,3.09077111588775,53.0896586316309));
#9213=CARTESIAN_POINT('Ctrl Pts',(-2.76299000531434,3.01120582074493,53.0954737721487));
#9214=CARTESIAN_POINT('Ctrl Pts',(-2.84854990754255,2.92796660230941,53.1012889126665));
#9215=CARTESIAN_POINT('Ctrl Pts',(-2.93416616224167,2.8446725598791,53.1071078832206));
#9216=CARTESIAN_POINT('Ctrl Pts',(-3.01604393215193,2.75770007124546,53.1129268537748));
#9217=CARTESIAN_POINT('Ctrl Pts',(-3.09387126105113,2.667430527688,53.118745824329));
#9218=CARTESIAN_POINT('Ctrl Pts',(-3.17180810857496,2.57703395682027,53.1245729833391));
#9219=CARTESIAN_POINT('Ctrl Pts',(-3.24568288782318,2.4833313902525,53.1304001423491));
#9220=CARTESIAN_POINT('Ctrl Pts',(-3.31522599577638,2.38673450491012,53.1362273013592));
#9221=CARTESIAN_POINT('Ctrl Pts',(-3.33041765044895,2.36563296706175,53.1375002411229));
#9222=CARTESIAN_POINT('Ctrl Pts',(-3.34540276909452,2.34439340882316,53.1387731808866));
#9223=CARTESIAN_POINT('Ctrl Pts',(-3.36017883296746,2.32302027767246,53.1400461206503));
#9224=CARTESIAN_POINT('Ctrl Pts',(-3.42855138775025,2.22412143742332,53.1459363323112));
#9225=CARTESIAN_POINT('Ctrl Pts',(-3.49265941604598,2.12204927775056,53.1518265439721));
#9226=CARTESIAN_POINT('Ctrl Pts',(-3.55219939808078,2.01720213074311,53.1577167556331));
#9227=CARTESIAN_POINT('Ctrl Pts',(-3.61166123393254,1.91249259553971,53.1635992363955));
#9228=CARTESIAN_POINT('Ctrl Pts',(-3.66656675741592,1.80501565989358,53.1694817171579));
#9229=CARTESIAN_POINT('Ctrl Pts',(-3.71665474298537,1.69519984705178,53.1753641979204));
#9230=CARTESIAN_POINT('Ctrl Pts',(-3.7666878415431,1.58550437168689,53.1812402325903));
#9231=CARTESIAN_POINT('Ctrl Pts',(-3.81191374341681,1.47347547702521,53.1871162672601));
#9232=CARTESIAN_POINT('Ctrl Pts',(-3.85211657335827,1.3595671757065,53.19299230193));
#9233=CARTESIAN_POINT('Ctrl Pts',(-3.89227897573479,1.24577341943986,53.198862427718));
#9234=CARTESIAN_POINT('Ctrl Pts',(-3.9274282343796,1.13010439218986,53.204732553506));
#9235=CARTESIAN_POINT('Ctrl Pts',(-3.95739640388031,1.01303440344108,53.210602679294));
#9236=CARTESIAN_POINT('Ctrl Pts',(-3.98734661432799,0.896034571334156,53.2164692872863));
#9237=CARTESIAN_POINT('Ctrl Pts',(-4.01212181647168,0.777635831074868,53.2223358952785));
#9238=CARTESIAN_POINT('Ctrl Pts',(-4.03160383849986,0.658327797828088,53.2282025032707));
#9239=CARTESIAN_POINT('Ctrl Pts',(-4.05108012858619,0.539054867031542,53.2340673852072));
#9240=CARTESIAN_POINT('Ctrl Pts',(-4.06526627018128,0.418873565411573,53.2399322671437));
#9241=CARTESIAN_POINT('Ctrl Pts',(-4.074095230338,0.298283513016052,53.2457971490802));
#9242=CARTESIAN_POINT('Ctrl Pts',(-4.08141537212827,0.19830160502653,53.2506597565216));
#9243=CARTESIAN_POINT('Ctrl Pts',(-4.0850538085329,0.0980390096750171,53.2555223639631));
#9244=CARTESIAN_POINT('Ctrl Pts',(-4.08499939840981,-0.0022169780104106,
53.2603849714045));
#9245=CARTESIAN_POINT('Origin',(0.,0.,46.4896150285955));
#9246=CARTESIAN_POINT('',(-2.31338095599002,-3.36682247118298,50.953013989131));
#9247=CARTESIAN_POINT('',(-2.31338095599002,-3.36682247118299,51.0573853382455));
#9248=CARTESIAN_POINT('',(-2.31338095599002,-3.36682247118298,46.4896150285955));
#9249=CARTESIAN_POINT('',(-4.08744329586254,-0.00250500349578786,50.7603840336099));
#9250=CARTESIAN_POINT('Ctrl Pts',(-4.08499922105558,-0.00252269208140621,
50.7603849714045));
#9251=CARTESIAN_POINT('Ctrl Pts',(-4.08489554760012,-0.17040128016159,50.7685938243239));
#9252=CARTESIAN_POINT('Ctrl Pts',(-4.07444292066524,-0.337949364085238,
50.7768026772432));
#9253=CARTESIAN_POINT('Ctrl Pts',(-4.05376347893569,-0.504208941657341,
50.7850115301626));
#9254=CARTESIAN_POINT('Ctrl Pts',(-4.0390990543464,-0.622108692987181,50.7908326788268));
#9255=CARTESIAN_POINT('Ctrl Pts',(-4.0192630313701,-0.739559716220486,50.796653827491));
#9256=CARTESIAN_POINT('Ctrl Pts',(-3.99429146142702,-0.856072848051627,
50.8024749761552));
#9257=CARTESIAN_POINT('Ctrl Pts',(-3.96935207559578,-0.972435814247411,
50.8082886223475));
#9258=CARTESIAN_POINT('Ctrl Pts',(-3.93929039337994,-1.08786289707374,50.8141022685399));
#9259=CARTESIAN_POINT('Ctrl Pts',(-3.90419418194402,-1.2018705378178,50.8199159147323));
#9260=CARTESIAN_POINT('Ctrl Pts',(-3.86913946520073,-1.31574338589288,50.8257226873776));
#9261=CARTESIAN_POINT('Ctrl Pts',(-3.82906218921653,-1.42819974450792,50.8315294600229));
#9262=CARTESIAN_POINT('Ctrl Pts',(-3.78410087487403,-1.53876754864975,50.8373362326682));
#9263=CARTESIAN_POINT('Ctrl Pts',(-3.73916942985995,-1.64926189884342,50.8431391476772));
#9264=CARTESIAN_POINT('Ctrl Pts',(-3.68936055212682,-1.75786981223455,50.8489420626861));
#9265=CARTESIAN_POINT('Ctrl Pts',(-3.63486208925382,-1.8641358834874,50.8547449776951));
#9266=CARTESIAN_POINT('Ctrl Pts',(-3.58038693189061,-1.97035651153262,50.8605454111682));
#9267=CARTESIAN_POINT('Ctrl Pts',(-3.52122636487616,-2.07423692646578,50.8663458446412));
#9268=CARTESIAN_POINT('Ctrl Pts',(-3.45761544334531,-2.17534375351115,50.8721462781143));
#9269=CARTESIAN_POINT('Ctrl Pts',(-3.39401666823448,-2.27643127434372,50.8779456040024));
#9270=CARTESIAN_POINT('Ctrl Pts',(-3.3259694479581,-2.37474591591575,50.8837449298905));
#9271=CARTESIAN_POINT('Ctrl Pts',(-3.2537533285065,-2.4698814297923,50.8895442557786));
#9272=CARTESIAN_POINT('Ctrl Pts',(-3.18150701820337,-2.56505671625976,50.8953460061474));
#9273=CARTESIAN_POINT('Ctrl Pts',(-3.10508857127888,-2.65704989170036,50.9011477565161));
#9274=CARTESIAN_POINT('Ctrl Pts',(-3.02481911174047,-2.74548617575278,50.9069495068849));
#9275=CARTESIAN_POINT('Ctrl Pts',(-2.94453257356551,-2.83394127606684,50.9127524916707));
#9276=CARTESIAN_POINT('Ctrl Pts',(-2.86039367350361,-2.91883768214517,50.9185554764565));
#9277=CARTESIAN_POINT('Ctrl Pts',(-2.77276092894155,-2.9998369673926,50.9243584612423));
#9278=CARTESIAN_POINT('Ctrl Pts',(-2.6850428209863,-3.080915154355,50.9301670987379));
#9279=CARTESIAN_POINT('Ctrl Pts',(-2.59382437887124,-3.15808836898283,50.9359757362334));
#9280=CARTESIAN_POINT('Ctrl Pts',(-2.49949784853709,-3.23105795447226,50.941784373729));
#9281=CARTESIAN_POINT('Ctrl Pts',(-2.43871189780588,-3.27808105192665,50.945527578863));
#9282=CARTESIAN_POINT('Ctrl Pts',(-2.37663587796835,-3.32335931471133,50.949270783997));
#9283=CARTESIAN_POINT('Ctrl Pts',(-2.31338095599002,-3.36682247118298,50.953013989131));
#9284=CARTESIAN_POINT('',(3.17505078219416,-2.57026798806822,50.));
#9285=CARTESIAN_POINT('Ctrl Pts',(3.17505078219411,-2.57026798806828,50.));
#9286=CARTESIAN_POINT('Ctrl Pts',(4.02021879563803,-1.52623235652025,50.0654176275135));
#9287=CARTESIAN_POINT('Ctrl Pts',(4.58685143039127,1.44312147364938,50.1962528825406));
#9288=CARTESIAN_POINT('Ctrl Pts',(1.3219330033413,4.62797967283566,50.3925057650812));
#9289=CARTESIAN_POINT('Ctrl Pts',(-2.94254776511638,3.69335577407833,50.5805492729265));
#9290=CARTESIAN_POINT('Ctrl Pts',(-4.08029497582926,1.16864264796801,50.7031751532581));
#9291=CARTESIAN_POINT('Ctrl Pts',(-4.08907877044555,-0.00249316702003614,
50.7603834060762));
#9292=CARTESIAN_POINT('',(1.46246200503919,-3.81424040718683,50.0000002080809));
#9293=CARTESIAN_POINT('Origin',(0.,0.,50.));
#9294=CARTESIAN_POINT('',(-4.08499988058316,0.000987742680470998,50.8646150285511));
#9295=CARTESIAN_POINT('Ctrl Pts',(1.46246200503919,-3.81424040718683,50.0000002080809));
#9296=CARTESIAN_POINT('Ctrl Pts',(1.57281875983439,-3.77192724816746,50.005789033466));
#9297=CARTESIAN_POINT('Ctrl Pts',(1.68152243212576,-3.72474980731752,50.0115778588512));
#9298=CARTESIAN_POINT('Ctrl Pts',(1.78811065278834,-3.67285791903048,50.0173666842363));
#9299=CARTESIAN_POINT('Ctrl Pts',(1.89456686500696,-3.62103029832745,50.0231483402192));
#9300=CARTESIAN_POINT('Ctrl Pts',(1.9989124667768,-3.56450002029049,50.028929996202));
#9301=CARTESIAN_POINT('Ctrl Pts',(2.1007027958165,-3.50346582167555,50.0347116521849));
#9302=CARTESIAN_POINT('Ctrl Pts',(2.20239442697394,-3.44249080300635,50.0404877021617));
#9303=CARTESIAN_POINT('Ctrl Pts',(2.30153536049967,-3.37702076131729,50.0462637521385));
#9304=CARTESIAN_POINT('Ctrl Pts',(2.39770399593268,-3.30730109725263,50.0520398021153));
#9305=CARTESIAN_POINT('Ctrl Pts',(2.49380794685844,-3.2376283277092,50.0578119670318));
#9306=CARTESIAN_POINT('Ctrl Pts',(2.58694324233037,-3.16371186332526,50.0635841319483));
#9307=CARTESIAN_POINT('Ctrl Pts',(2.67671637718872,-3.08584096091968,50.0693562968649));
#9308=CARTESIAN_POINT('Ctrl Pts',(2.7664581058625,-3.00799730082816,50.0751264424503));
#9309=CARTESIAN_POINT('Ctrl Pts',(2.85283969999958,-2.92620222359289,50.0808965880358));
#9310=CARTESIAN_POINT('Ctrl Pts',(2.93550041055213,-2.84078551454492,50.0866667336213));
#9311=CARTESIAN_POINT('Ctrl Pts',(3.01815231908193,-2.75537790098878,50.09243626478));
#9312=CARTESIAN_POINT('Ctrl Pts',(3.09708384437165,-2.66634971987523,50.0982057959388));
#9313=CARTESIAN_POINT('Ctrl Pts',(3.17197133573925,-2.57406737387516,50.1039753270975));
#9314=CARTESIAN_POINT('Ctrl Pts',(3.24686907737394,-2.48177239667758,50.109745647964));
#9315=CARTESIAN_POINT('Ctrl Pts',(3.31772142436844,-2.38622269065863,50.1155159688305));
#9316=CARTESIAN_POINT('Ctrl Pts',(3.38424568780932,-2.287816890519,50.121286289697));
#9317=CARTESIAN_POINT('Ctrl Pts',(3.45083484815304,-2.1893150918471,50.127062239727));
#9318=CARTESIAN_POINT('Ctrl Pts',(3.51308726037022,-2.08795197779127,50.132838189757));
#9319=CARTESIAN_POINT('Ctrl Pts',(3.57076411768132,-1.98415438307596,50.138614139787));
#9320=CARTESIAN_POINT('Ctrl Pts',(3.62847000267175,-1.88030454898018,50.1443929967441));
#9321=CARTESIAN_POINT('Ctrl Pts',(3.68159556108044,-1.77401816375787,50.1501718537013));
#9322=CARTESIAN_POINT('Ctrl Pts',(3.72994921676155,-1.66574423018059,50.1559507106585));
#9323=CARTESIAN_POINT('Ctrl Pts',(3.77837747178567,-1.55730325309447,50.1617384831552));
#9324=CARTESIAN_POINT('Ctrl Pts',(3.82201896532527,-1.44686898697977,50.167526255652));
#9325=CARTESIAN_POINT('Ctrl Pts',(3.86073114014527,-1.33490826033575,50.1733140281488));
#9326=CARTESIAN_POINT('Ctrl Pts',(3.89203796568312,-1.24436478267184,50.1779946430885));
#9327=CARTESIAN_POINT('Ctrl Pts',(3.92012191362614,-1.1528233751915,50.1826752580281));
#9328=CARTESIAN_POINT('Ctrl Pts',(3.94493205986919,-1.06053573396478,50.1873558729678));
#9329=CARTESIAN_POINT('Ctrl Pts',(3.97586421810565,-0.945475714014513,50.1931914500958));
#9330=CARTESIAN_POINT('Ctrl Pts',(4.00180582916819,-0.828884727081285,50.1990270272237));
#9331=CARTESIAN_POINT('Ctrl Pts',(4.0226077902163,-0.711232427615012,50.2048626043517));
#9332=CARTESIAN_POINT('Ctrl Pts',(4.04338434750931,-0.593723807400644,50.2106910549606));
#9333=CARTESIAN_POINT('Ctrl Pts',(4.05903367022548,-0.475156849716197,50.2165195055695));
#9334=CARTESIAN_POINT('Ctrl Pts',(4.06945674036903,-0.356015221957,50.2223479561784));
#9335=CARTESIAN_POINT('Ctrl Pts',(4.07986976374012,-0.236988434528732,50.2281707887577));
#9336=CARTESIAN_POINT('Ctrl Pts',(4.08506652215019,-0.117388481742685,50.2339936213369));
#9337=CARTESIAN_POINT('Ctrl Pts',(4.08499935671531,0.00229251727920632,
50.2398164539162));
#9338=CARTESIAN_POINT('Ctrl Pts',(4.08493024750646,0.125437095626447,50.2458077998159));
#9339=CARTESIAN_POINT('Ctrl Pts',(4.07928781543186,0.248667050864927,50.2517991457155));
#9340=CARTESIAN_POINT('Ctrl Pts',(4.06807764895099,0.371442111378571,50.2577904916152));
#9341=CARTESIAN_POINT('Ctrl Pts',(4.05719422942123,0.490638600890343,50.2636072054959));
#9342=CARTESIAN_POINT('Ctrl Pts',(4.04106319214363,0.609405915005833,50.2694239193766));
#9343=CARTESIAN_POINT('Ctrl Pts',(4.0197424561347,0.727252078957643,50.2752406332573));
#9344=CARTESIAN_POINT('Ctrl Pts',(3.99842440272144,0.845083415390828,50.2810566152734));
#9345=CARTESIAN_POINT('Ctrl Pts',(3.97191802161883,0.961993432446621,50.2868725972895));
#9346=CARTESIAN_POINT('Ctrl Pts',(3.94033263351198,1.07749883400428,50.2926885793056));
#9347=CARTESIAN_POINT('Ctrl Pts',(3.90874385921344,1.19301661861163,50.2985051848388));
#9348=CARTESIAN_POINT('Ctrl Pts',(3.87207510227841,1.30712909633735,50.304321790372));
#9349=CARTESIAN_POINT('Ctrl Pts',(3.83048581820237,1.41936725217631,50.3101383959053));
#9350=CARTESIAN_POINT('Ctrl Pts',(3.78670914526065,1.5375085750892,50.3162609258722));
#9351=CARTESIAN_POINT('Ctrl Pts',(3.73748046088016,1.65357258449981,50.3223834558391));
#9352=CARTESIAN_POINT('Ctrl Pts',(3.68304315640458,1.76703653274666,50.328505985806));
#9353=CARTESIAN_POINT('Ctrl Pts',(3.63124944958615,1.87499041706503,50.3343311919794));
#9354=CARTESIAN_POINT('Ctrl Pts',(3.57474134718814,1.98059048751101,50.3401563981528));
#9355=CARTESIAN_POINT('Ctrl Pts',(3.51377502506969,2.08341308270743,50.3459816043262));
#9356=CARTESIAN_POINT('Ctrl Pts',(3.45276743203757,2.18630528325814,50.3518107538502));
#9357=CARTESIAN_POINT('Ctrl Pts',(3.38729583027118,2.2864159246399,50.3576399033742));
#9358=CARTESIAN_POINT('Ctrl Pts',(3.31765886986535,2.38335155258383,50.3634690528981));
#9359=CARTESIAN_POINT('Ctrl Pts',(3.24792504971802,2.48042201064974,50.3693063103279));
#9360=CARTESIAN_POINT('Ctrl Pts',(3.17401455895687,2.57430832408995,50.3751435677577));
#9361=CARTESIAN_POINT('Ctrl Pts',(3.09626535598136,2.6646511676671,50.3809808251875));
#9362=CARTESIAN_POINT('Ctrl Pts',(3.08459780545874,2.67820860171726,50.3818568019611));
#9363=CARTESIAN_POINT('Ctrl Pts',(3.07284387231894,2.69168630714175,50.3827327787348));
#9364=CARTESIAN_POINT('Ctrl Pts',(3.06100476611686,2.70508314508258,50.3836087555084));
#9365=CARTESIAN_POINT('Ctrl Pts',(2.98233802783124,2.79410046836335,50.3894293161504));
#9366=CARTESIAN_POINT('Ctrl Pts',(2.89965717996909,2.87982798958123,50.3952498767924));
#9367=CARTESIAN_POINT('Ctrl Pts',(2.81326808570803,2.96188245511814,50.4010704374344));
#9368=CARTESIAN_POINT('Ctrl Pts',(2.72698833177785,3.04383306654605,50.4068836311508));
#9369=CARTESIAN_POINT('Ctrl Pts',(2.63700996013592,3.12211958956528,50.4126968248672));
#9370=CARTESIAN_POINT('Ctrl Pts',(2.54367836128961,3.19639255948124,50.4185100185837));
#9371=CARTESIAN_POINT('Ctrl Pts',(2.45044049148093,3.27059094014683,50.4243173743518));
#9372=CARTESIAN_POINT('Ctrl Pts',(2.3538564115977,3.34078353291223,50.4301247301199));
#9373=CARTESIAN_POINT('Ctrl Pts',(2.25430710778994,3.40665884170513,50.4359320858879));
#9374=CARTESIAN_POINT('Ctrl Pts',(2.15150582662759,3.47468609937388,50.4419291505613));
#9375=CARTESIAN_POINT('Ctrl Pts',(2.04554259183216,3.53810886625143,50.4479262152347));
#9376=CARTESIAN_POINT('Ctrl Pts',(1.93687288945575,3.59663014641363,50.4539232799081));
#9377=CARTESIAN_POINT('Ctrl Pts',(1.83175977362679,3.65323611813923,50.4597240701915));
#9378=CARTESIAN_POINT('Ctrl Pts',(1.72411496627118,3.70525621613186,50.4655248604749));
#9379=CARTESIAN_POINT('Ctrl Pts',(1.61437806486332,3.75246698369062,50.4713256507583));
#9380=CARTESIAN_POINT('Ctrl Pts',(1.50465761465709,3.79967067364971,50.4771255714166));
#9381=CARTESIAN_POINT('Ctrl Pts',(1.39284606955893,3.84206630548709,50.4829254920749));
#9382=CARTESIAN_POINT('Ctrl Pts',(1.2794043061154,3.87947800889416,50.4887254127331));
#9383=CARTESIAN_POINT('Ctrl Pts',(1.16595269870593,3.91689295872056,50.4945258366824));
#9384=CARTESIAN_POINT('Ctrl Pts',(1.05087097998002,3.9493229922709,50.5003262606317));
#9385=CARTESIAN_POINT('Ctrl Pts',(0.934635909121122,3.97664188950694,50.506126684581));
#9386=CARTESIAN_POINT('Ctrl Pts',(0.818363240305797,4.00396962344519,50.5119289847633));
#9387=CARTESIAN_POINT('Ctrl Pts',(0.700936875202572,4.026182839741,50.5177312849457));
#9388=CARTESIAN_POINT('Ctrl Pts',(0.582843859901059,4.04320640519077,50.5235335851281));
#9389=CARTESIAN_POINT('Ctrl Pts',(0.464621020012701,4.06024868535745,50.5293422640215));
#9390=CARTESIAN_POINT('Ctrl Pts',(0.345730471955937,4.07208986877292,50.535150942915));
#9391=CARTESIAN_POINT('Ctrl Pts',(0.226664622678819,4.07870667599741,50.5409596218084));
#9392=CARTESIAN_POINT('Ctrl Pts',(0.107520475418681,4.08532783444993,50.5467721205028));
#9393=CARTESIAN_POINT('Ctrl Pts',(-0.0117987948272657,4.08671777019441,
50.5525846191972));
#9394=CARTESIAN_POINT('Ctrl Pts',(-0.130802197900687,4.08290531178772,50.5583971178916));
#9395=CARTESIAN_POINT('Ctrl Pts',(-0.2499739328687,4.07908746060796,50.5642178384426));
#9396=CARTESIAN_POINT('Ctrl Pts',(-0.368828502858761,4.07005255946358,50.5700385589936));
#9397=CARTESIAN_POINT('Ctrl Pts',(-0.486881335483542,4.05588110836077,50.5758592795445));
#9398=CARTESIAN_POINT('Ctrl Pts',(-0.51393925465946,4.05263298656631,50.5771933990461));
#9399=CARTESIAN_POINT('Ctrl Pts',(-0.5409551053352,4.04911523465669,50.5785275185476));
#9400=CARTESIAN_POINT('Ctrl Pts',(-0.567923149774569,4.04532919500381,50.5798616380491));
#9401=CARTESIAN_POINT('Ctrl Pts',(-0.685726289369142,4.02879083017196,50.5856894045461));
#9402=CARTESIAN_POINT('Ctrl Pts',(-0.802993418979347,4.00707616775879,50.5915171710431));
#9403=CARTESIAN_POINT('Ctrl Pts',(-0.919235126998391,3.98023011662545,50.5973449375401));
#9404=CARTESIAN_POINT('Ctrl Pts',(-1.0353315133892,3.95341762755799,50.6031654183517));
#9405=CARTESIAN_POINT('Ctrl Pts',(-1.15040463430047,3.9214866007382,50.6089858991633));
#9406=CARTESIAN_POINT('Ctrl Pts',(-1.26397159091224,3.88453353922537,50.6148063799749));
#9407=CARTESIAN_POINT('Ctrl Pts',(-1.37742604064251,3.84761708584079,50.6206210946361));
#9408=CARTESIAN_POINT('Ctrl Pts',(-1.48937690910271,3.80568862107416,50.6264358092974));
#9409=CARTESIAN_POINT('Ctrl Pts',(-1.59935344743643,3.75889525661107,50.6322505239587));
#9410=CARTESIAN_POINT('Ctrl Pts',(-1.71272719878724,3.71065642905853,50.6382448571516));
#9411=CARTESIAN_POINT('Ctrl Pts',(-1.82400223363396,3.65724736251386,50.6442391903446));
#9412=CARTESIAN_POINT('Ctrl Pts',(-1.93268140335395,3.59888421502135,50.6502335235376));
#9413=CARTESIAN_POINT('Ctrl Pts',(-2.0379873814761,3.54233254694345,50.6560418042016));
#9414=CARTESIAN_POINT('Ctrl Pts',(-2.14085586804854,3.48112998805264,50.6618500848658));
#9415=CARTESIAN_POINT('Ctrl Pts',(-2.24085734570053,3.4155209494629,50.6676583655299));
#9416=CARTESIAN_POINT('Ctrl Pts',(-2.34084446549131,3.34992133078868,50.6734658122614));
#9417=CARTESIAN_POINT('Ctrl Pts',(-2.43796505430244,3.27991671423282,50.6792732589929));
#9418=CARTESIAN_POINT('Ctrl Pts',(-2.53181760052623,3.20579547658075,50.6850807057245));
#9419=CARTESIAN_POINT('Ctrl Pts',(-2.62567872512337,3.13166746404962,50.6908886832722));
#9420=CARTESIAN_POINT('Ctrl Pts',(-2.71627089332352,3.05342233495526,50.6966966608199));
#9421=CARTESIAN_POINT('Ctrl Pts',(-2.80322528081623,2.97138907331113,50.7025046383675));
#9422=CARTESIAN_POINT('Ctrl Pts',(-2.89020804844925,2.88932903768189,50.7083145115208));
#9423=CARTESIAN_POINT('Ctrl Pts',(-2.97355037769829,2.80347869014922,50.714124384674));
#9424=CARTESIAN_POINT('Ctrl Pts',(-3.05292040165361,2.71420375454149,50.7199342578272));
#9425=CARTESIAN_POINT('Ctrl Pts',(-3.13237744299417,2.62483094229122,50.7257505006392));
#9426=CARTESIAN_POINT('Ctrl Pts',(-3.20785321528757,2.53202635258575,50.7315667434512));
#9427=CARTESIAN_POINT('Ctrl Pts',(-3.27905615631144,2.43618877013996,50.7373829862632));
#9428=CARTESIAN_POINT('Ctrl Pts',(-3.35030590092513,2.34028819109833,50.7432030522465));
#9429=CARTESIAN_POINT('Ctrl Pts',(-3.41727699259905,2.24135098549292,50.7490231182298));
#9430=CARTESIAN_POINT('Ctrl Pts',(-3.47972211153957,2.13980350183436,50.7548431842132));
#9431=CARTESIAN_POINT('Ctrl Pts',(-3.54225489158131,2.0381134647722,50.7606714204651));
#9432=CARTESIAN_POINT('Ctrl Pts',(-3.60024882084813,1.933806191218,50.766499656717));
#9433=CARTESIAN_POINT('Ctrl Pts',(-3.65350321437514,1.82733118578723,50.7723278929689));
#9434=CARTESIAN_POINT('Ctrl Pts',(-3.66503640948176,1.80427211159105,50.7735901021758));
#9435=CARTESIAN_POINT('Ctrl Pts',(-3.67634749467981,1.78111143438283,50.7748523113828));
#9436=CARTESIAN_POINT('Ctrl Pts',(-3.68743473585548,1.7578538246414,50.7761145205898));
#9437=CARTESIAN_POINT('Ctrl Pts',(-3.74247739978587,1.64239130546845,50.782380764472));
#9438=CARTESIAN_POINT('Ctrl Pts',(-3.79215297082213,1.52421596465456,50.7886470083543));
#9439=CARTESIAN_POINT('Ctrl Pts',(-3.83620714792583,1.40383037372853,50.7949132522366));
#9440=CARTESIAN_POINT('Ctrl Pts',(-3.88012390350456,1.28382031067697,50.8011599493506));
#9441=CARTESIAN_POINT('Ctrl Pts',(-3.91845412677658,1.16161403697445,50.8074066464647));
#9442=CARTESIAN_POINT('Ctrl Pts',(-3.95099138915027,1.03773409063231,50.8136533435787));
#9443=CARTESIAN_POINT('Ctrl Pts',(-3.98346592666386,0.914092958244832,50.8198879984011));
#9444=CARTESIAN_POINT('Ctrl Pts',(-4.01016967757586,0.788784880497225,50.8261226532235));
#9445=CARTESIAN_POINT('Ctrl Pts',(-4.03094500985105,0.662349852839839,50.8323573080459));
#9446=CARTESIAN_POINT('Ctrl Pts',(-4.05165968241143,0.53628398956535,50.8385737589533));
#9447=CARTESIAN_POINT('Ctrl Pts',(-4.06648039935784,0.40909804205386,50.8447902098606));
#9448=CARTESIAN_POINT('Ctrl Pts',(-4.07530010119103,0.281343358251793,50.851006660768));
#9449=CARTESIAN_POINT('Ctrl Pts',(-4.08173580692684,0.188121210057571,50.8555427833624));
#9450=CARTESIAN_POINT('Ctrl Pts',(-4.08497724620056,0.0945965863802722,
50.8600789059567));
#9451=CARTESIAN_POINT('Ctrl Pts',(-4.08499988058316,0.000987742680465642,
50.8646150285511));
#9452=CARTESIAN_POINT('Ctrl Pts',(-4.08499988058338,0.000987741764322645,
50.8646150285955));
#9453=CARTESIAN_POINT('Ctrl Pts',(-4.08502967467695,-0.122231578376562,
50.8705860236432));
#9454=CARTESIAN_POINT('Ctrl Pts',(-4.07947997096532,-0.24539499124926,50.8765570186908));
#9455=CARTESIAN_POINT('Ctrl Pts',(-4.06839208895291,-0.367982079108958,
50.8825280137385));
#9456=CARTESIAN_POINT('Ctrl Pts',(-4.05729609641797,-0.490658836513985,
50.8885033764273));
#9457=CARTESIAN_POINT('Ctrl Pts',(-4.04065388598581,-0.612758056698495,
50.8944787391161));
#9458=CARTESIAN_POINT('Ctrl Pts',(-4.01855840692874,-0.7337665365103,50.9004541018049));
#9459=CARTESIAN_POINT('Ctrl Pts',(-3.99639854085159,-0.855127639381329,
50.9064468769154));
#9460=CARTESIAN_POINT('Ctrl Pts',(-3.96875366769712,-0.975391269297092,
50.9124396520259));
#9461=CARTESIAN_POINT('Ctrl Pts',(-3.93576823229061,-1.09405366490498,50.9184324271363));
#9462=CARTESIAN_POINT('Ctrl Pts',(-3.90279218938141,-1.21268227177498,50.9244234958232));
#9463=CARTESIAN_POINT('Ctrl Pts',(-3.86447878240159,-1.32971021344599,50.9304145645101));
#9464=CARTESIAN_POINT('Ctrl Pts',(-3.82102101337489,-1.44465338934553,50.936405633197));
#9465=CARTESIAN_POINT('Ctrl Pts',(-3.77747245573135,-1.55983669565648,50.9424092179622));
#9466=CARTESIAN_POINT('Ctrl Pts',(-3.72875819676169,-1.67292618416678,50.9484128027274));
#9467=CARTESIAN_POINT('Ctrl Pts',(-3.67511885388689,-1.78345911357819,50.9544163874925));
#9468=CARTESIAN_POINT('Ctrl Pts',(-3.6216574237353,-1.89362542376159,50.9604000593718));
#9469=CARTESIAN_POINT('Ctrl Pts',(-3.56330377686136,-2.00125182718268,50.9663837312511));
#9470=CARTESIAN_POINT('Ctrl Pts',(-3.50033892327115,-2.105908930185,50.9723674031304));
#9471=CARTESIAN_POINT('Ctrl Pts',(-3.43902918689205,-2.20781497823259,50.9781937860183));
#9472=CARTESIAN_POINT('Ctrl Pts',(-3.37316769210698,-2.30720406476472,50.9840201689062));
#9473=CARTESIAN_POINT('Ctrl Pts',(-3.30298702653468,-2.40364342250334,50.9898465517941));
#9474=CARTESIAN_POINT('Ctrl Pts',(-3.23291250694739,-2.49993691883502,50.9956641224665));
#9475=CARTESIAN_POINT('Ctrl Pts',(-3.15853205917908,-2.59328924068462,51.0014816931389));
#9476=CARTESIAN_POINT('Ctrl Pts',(-3.08012300868858,-2.68329410451915,51.0072992638113));
#9477=CARTESIAN_POINT('Ctrl Pts',(-3.00178278679312,-2.77321996078648,51.0131117277362));
#9478=CARTESIAN_POINT('Ctrl Pts',(-2.91942125901157,-2.85980389522568,51.0189241916612));
#9479=CARTESIAN_POINT('Ctrl Pts',(-2.83335766623238,-2.94267044284646,51.0247366555862));
#9480=CARTESIAN_POINT('Ctrl Pts',(-2.74735299251528,-3.02548026009955,51.0305451403033));
#9481=CARTESIAN_POINT('Ctrl Pts',(-2.65765158807283,-3.10457747088664,51.0363536250205));
#9482=CARTESIAN_POINT('Ctrl Pts',(-2.5646109376554,-3.17962194898361,51.0421621097376));
#9483=CARTESIAN_POINT('Ctrl Pts',(-2.48332874727353,-3.24518231994423,51.0472365192402));
#9484=CARTESIAN_POINT('Ctrl Pts',(-2.39949871580841,-3.30765000597534,51.0523109287428));
#9485=CARTESIAN_POINT('Ctrl Pts',(-2.31338095599002,-3.36682247118299,51.0573853382455));
#9486=CARTESIAN_POINT('Origin',(0.,0.,0.));
#9487=CARTESIAN_POINT('',(-3.38700661857411,0.136349654327207,58.7578931987404));
#9488=CARTESIAN_POINT('',(-3.38228028396882,0.136179104830184,59.1010527180904));
#9489=CARTESIAN_POINT('',(-3.38700661857411,0.136349654327212,0.));
#9490=CARTESIAN_POINT('',(-3.38941152592639,0.000621225212723754,59.1089821571774));
#9491=CARTESIAN_POINT('Ctrl Pts',(-3.3822802839685,0.136179104839289,59.1010527180899));
#9492=CARTESIAN_POINT('Ctrl Pts',(-3.38391039591696,0.0910238355186148,
59.1036956766094));
#9493=CARTESIAN_POINT('Ctrl Pts',(-3.38468059381083,0.045828374490169,59.1063386351288));
#9494=CARTESIAN_POINT('Ctrl Pts',(-3.38459238031828,0.000629980057637551,
59.1089815936483));
#9495=CARTESIAN_POINT('',(0.784811935329644,3.29764693208114,60.));
#9496=CARTESIAN_POINT('Ctrl Pts',(-3.38974994318795,0.00062061041689021,
59.1089821967504));
#9497=CARTESIAN_POINT('Ctrl Pts',(-3.38976958113811,-0.106641109035038,
59.1152447433034));
#9498=CARTESIAN_POINT('Ctrl Pts',(-3.38469376469629,-0.213844138759583,
59.1215072898564));
#9499=CARTESIAN_POINT('Ctrl Pts',(-3.37456524596793,-0.320490972112212,
59.1277698364093));
#9500=CARTESIAN_POINT('Ctrl Pts',(-3.36442804830286,-0.427229189125262,
59.1340377492204));
#9501=CARTESIAN_POINT('Ctrl Pts',(-3.34922955936844,-0.533409872464934,
59.1403056620314));
#9502=CARTESIAN_POINT('Ctrl Pts',(-3.32906407250675,-0.638543235532868,
59.1465735748424));
#9503=CARTESIAN_POINT('Ctrl Pts',(-3.30886074569859,-0.743873878282574,
59.1528532492085));
#9504=CARTESIAN_POINT('Ctrl Pts',(-3.28367187382311,-0.848152890830866,
59.1591329235747));
#9505=CARTESIAN_POINT('Ctrl Pts',(-3.25364250612429,-0.950902468627188,
59.1654125979408));
#9506=CARTESIAN_POINT('Ctrl Pts',(-3.2235828914976,-1.05375554041308,59.171698597477));
#9507=CARTESIAN_POINT('Ctrl Pts',(-3.18867318755257,-1.15507573799927,59.1779845970132));
#9508=CARTESIAN_POINT('Ctrl Pts',(-3.14910709129851,-1.25440407765338,59.1842705965494));
#9509=CARTESIAN_POINT('Ctrl Pts',(-3.10945856420961,-1.35393935503287,59.1905696921511));
#9510=CARTESIAN_POINT('Ctrl Pts',(-3.06513441912835,-1.45147412624603,59.1968687877528));
#9511=CARTESIAN_POINT('Ctrl Pts',(-3.01637526412841,-1.54657212196983,59.2031678833546));
#9512=CARTESIAN_POINT('Ctrl Pts',(-2.98587555195019,-1.60605759702173,59.2071080788488));
#9513=CARTESIAN_POINT('Ctrl Pts',(-2.95364144219183,-1.66459015785701,59.2110482743431));
#9514=CARTESIAN_POINT('Ctrl Pts',(-2.91974031768174,-1.72206897068721,59.2149884698374));
#9515=CARTESIAN_POINT('Ctrl Pts',(-2.86712558833523,-1.81127640034992,59.2211036746426));
#9516=CARTESIAN_POINT('Ctrl Pts',(-2.81033235993871,-1.89821685460951,59.2272188794477));
#9517=CARTESIAN_POINT('Ctrl Pts',(-2.74958134053344,-1.98247509802528,59.2333340842529));
#9518=CARTESIAN_POINT('Ctrl Pts',(-2.68890965946338,-2.06662330363714,59.2394413028518));
#9519=CARTESIAN_POINT('Ctrl Pts',(-2.62429071108117,-2.14809592057705,59.2455485214508));
#9520=CARTESIAN_POINT('Ctrl Pts',(-2.55599019115997,-2.22650380758579,59.2516557400497));
#9521=CARTESIAN_POINT('Ctrl Pts',(-2.4877595740189,-2.30483144733883,59.2577567081609));
#9522=CARTESIAN_POINT('Ctrl Pts',(-2.41585515688706,-2.38010027576606,59.2638576762722));
#9523=CARTESIAN_POINT('Ctrl Pts',(-2.34058436746746,-2.45195225917368,59.2699586443834));
#9524=CARTESIAN_POINT('Ctrl Pts',(-2.26536746257994,-2.52375280548952,59.2760552449596));
#9525=CARTESIAN_POINT('Ctrl Pts',(-2.1867892855036,-2.59214107869901,59.2821518455358));
#9526=CARTESIAN_POINT('Ctrl Pts',(-2.10519520272108,-2.65679472691063,59.288248446112));
#9527=CARTESIAN_POINT('Ctrl Pts',(-2.0236315585697,-2.72142425611164,59.2943427723544));
#9528=CARTESIAN_POINT('Ctrl Pts',(-1.93905457831871,-2.78232166560899,59.3004370985968));
#9529=CARTESIAN_POINT('Ctrl Pts',(-1.8518433121115,-2.83920436212117,59.3065314248393));
#9530=CARTESIAN_POINT('Ctrl Pts',(-1.76464226969447,-2.89608039026607,59.3126250366429));
#9531=CARTESIAN_POINT('Ctrl Pts',(-1.67480791200506,-2.94894240899023,59.3187186484465));
#9532=CARTESIAN_POINT('Ctrl Pts',(-1.58274817452861,-2.99755121366197,59.3248122602502));
#9533=CARTESIAN_POINT('Ctrl Pts',(-1.49067567919406,-3.04616675465786,59.3309067165211));
#9534=CARTESIAN_POINT('Ctrl Pts',(-1.39637756776693,-3.09052771183969,59.337001172792));
#9535=CARTESIAN_POINT('Ctrl Pts',(-1.30028546643281,-3.13044130567618,59.3430956290629));
#9536=CARTESIAN_POINT('Ctrl Pts',(-1.20409757987879,-3.17039468563776,59.3491961603267));
#9537=CARTESIAN_POINT('Ctrl Pts',(-1.10611252594308,-3.20589168543545,59.3552966915905));
#9538=CARTESIAN_POINT('Ctrl Pts',(-1.00678092200151,-3.23678810514278,59.3613972228543));
#9539=CARTESIAN_POINT('Ctrl Pts',(-0.907397221978165,-3.26770072898196,
59.3675009536413));
#9540=CARTESIAN_POINT('Ctrl Pts',(-0.806665976843181,-3.29400785806359,
59.3736046844284));
#9541=CARTESIAN_POINT('Ctrl Pts',(-0.705050068363768,-3.31561600062496,
59.3797084152154));
#9542=CARTESIAN_POINT('Ctrl Pts',(-0.603275798898071,-3.33725781790143,
59.385821658222));
#9543=CARTESIAN_POINT('Ctrl Pts',(-0.500614532174362,-3.354185950616,59.3919349012286));
#9544=CARTESIAN_POINT('Ctrl Pts',(-0.397536566596506,-3.36635852824958,
59.3980481442351));
#9545=CARTESIAN_POINT('Ctrl Pts',(-0.323384486521762,-3.37511521981155,
59.4024458802828));
#9546=CARTESIAN_POINT('Ctrl Pts',(-0.24901688977199,-3.38141197800158,59.4068436163304));
#9547=CARTESIAN_POINT('Ctrl Pts',(-0.174608662886954,-3.38524989880287,
59.411241352378));
#9548=CARTESIAN_POINT('Ctrl Pts',(-0.0712383170763532,-3.39058166407979,
59.4173508313303));
#9549=CARTESIAN_POINT('Ctrl Pts',(0.032545193583603,-3.39118312805083,59.4234603102825));
#9550=CARTESIAN_POINT('Ctrl Pts',(0.136274250313483,-3.38700965324894,59.4295697892348));
#9551=CARTESIAN_POINT('Ctrl Pts',(0.239870040415355,-3.38284154034787,59.4356714189914));
#9552=CARTESIAN_POINT('Ctrl Pts',(0.343411093082286,-3.37391070268049,59.441773048748));
#9553=CARTESIAN_POINT('Ctrl Pts',(0.446426780436103,-3.36022442586942,59.4478746785046));
#9554=CARTESIAN_POINT('Ctrl Pts',(0.549339343826491,-3.34655184972031,59.4539702002183));
#9555=CARTESIAN_POINT('Ctrl Pts',(0.651727167272397,-3.32813335731369,59.460065721932));
#9556=CARTESIAN_POINT('Ctrl Pts',(0.753122600543466,-3.30502820124892,59.4661612436456));
#9557=CARTESIAN_POINT('Ctrl Pts',(0.854449270320235,-3.28193871444277,59.4722526315501));
#9558=CARTESIAN_POINT('Ctrl Pts',(0.954784473738238,-3.25416897903038,59.4783440194545));
#9559=CARTESIAN_POINT('Ctrl Pts',(1.05366943498394,-3.22182957095509,59.484435407359));
#9560=CARTESIAN_POINT('Ctrl Pts',(1.1525198355889,-3.18950146561633,59.4905246663021));
#9561=CARTESIAN_POINT('Ctrl Pts',(1.24992059666244,-3.15260699449364,59.4966139252451));
#9562=CARTESIAN_POINT('Ctrl Pts',(1.34542759362092,-3.11130674360845,59.5027031841882));
#9563=CARTESIAN_POINT('Ctrl Pts',(1.44092574753966,-3.07001031673377,59.5087918793237));
#9564=CARTESIAN_POINT('Ctrl Pts',(1.53453009476259,-3.02430909064457,59.5148805744593));
#9565=CARTESIAN_POINT('Ctrl Pts',(1.62581684242783,-2.97441164894471,59.5209692695949));
#9566=CARTESIAN_POINT('Ctrl Pts',(1.71711859007868,-2.92450600823539,59.5270589652079));
#9567=CARTESIAN_POINT('Ctrl Pts',(1.80610160734986,-2.87040298633066,59.533148660821));
#9568=CARTESIAN_POINT('Ctrl Pts',(1.89236783500343,-2.81235649225777,59.5392383564341));
#9569=CARTESIAN_POINT('Ctrl Pts',(1.97872391772104,-2.7542495368481,59.5453343950856));
#9570=CARTESIAN_POINT('Ctrl Pts',(2.06235720538278,-2.69219114507215,59.551430433737));
#9571=CARTESIAN_POINT('Ctrl Pts',(2.14289974529792,-2.62647782098043,59.5575264723884));
#9572=CARTESIAN_POINT('Ctrl Pts',(2.22348644605957,-2.56072846678559,59.5636258534503));
#9573=CARTESIAN_POINT('Ctrl Pts',(2.30097870578457,-2.49132047282192,59.5697252345122));
#9574=CARTESIAN_POINT('Ctrl Pts',(2.37504418729172,-2.4185884666292,59.5758246155741));
#9575=CARTESIAN_POINT('Ctrl Pts',(2.4492285035767,-2.34573976516061,59.5819337828222));
#9576=CARTESIAN_POINT('Ctrl Pts',(2.51997476855938,-2.26955671052065,59.5880429500703));
#9577=CARTESIAN_POINT('Ctrl Pts',(2.58698967555324,-2.19040851922214,59.5941521173184));
#9578=CARTESIAN_POINT('Ctrl Pts',(2.63577541747057,-2.13278994736818,59.5985994898518));
#9579=CARTESIAN_POINT('Ctrl Pts',(2.68258452817756,-2.07360068171943,59.6030468623852));
#9580=CARTESIAN_POINT('Ctrl Pts',(2.72731848949463,-2.01299252839168,59.6074942349187));
#9581=CARTESIAN_POINT('Ctrl Pts',(2.78816077688645,-1.93055988494842,59.613543069179));
#9582=CARTESIAN_POINT('Ctrl Pts',(2.84537453202934,-1.84521426173784,59.6195919034394));
#9583=CARTESIAN_POINT('Ctrl Pts',(2.89866549401247,-1.75731141700083,59.6256407376998));
#9584=CARTESIAN_POINT('Ctrl Pts',(2.95188611923875,-1.6695245919562,59.6316815883291));
#9585=CARTESIAN_POINT('Ctrl Pts',(3.00119401608682,-1.57918762171329,59.6377224389583));
#9586=CARTESIAN_POINT('Ctrl Pts',(3.04633616420661,-1.48668794208702,59.6437632895875));
#9587=CARTESIAN_POINT('Ctrl Pts',(3.09143222324147,-1.3942827024856,59.6497979726486));
#9588=CARTESIAN_POINT('Ctrl Pts',(3.13237079724932,-1.29971953192066,59.6558326557096));
#9589=CARTESIAN_POINT('Ctrl Pts',(3.16894357674446,-1.20341251028482,59.6618673387706));
#9590=CARTESIAN_POINT('Ctrl Pts',(3.2054922146009,-1.1071690607743,59.6678980383461));
#9591=CARTESIAN_POINT('Ctrl Pts',(3.23768063031878,-1.00918445394829,59.6739287379216));
#9592=CARTESIAN_POINT('Ctrl Pts',(3.26534803997469,-0.90989408193123,59.679959437497));
#9593=CARTESIAN_POINT('Ctrl Pts',(3.29300616308019,-0.810637036671354,59.6859881128716));
#9594=CARTESIAN_POINT('Ctrl Pts',(3.31614617738074,-0.710075516331877,59.6920167882462));
#9595=CARTESIAN_POINT('Ctrl Pts',(3.33465701319445,-0.608660551418521,59.6980454636208));
#9596=CARTESIAN_POINT('Ctrl Pts',(3.35316664186638,-0.507252200049869,59.7040737458491));
#9597=CARTESIAN_POINT('Ctrl Pts',(3.36704761369299,-0.404990943633947,59.7101020280775));
#9598=CARTESIAN_POINT('Ctrl Pts',(3.37624008473162,-0.302337481552332,59.7161303103058));
#9599=CARTESIAN_POINT('Ctrl Pts',(3.38543444239343,-0.199662951316172,59.7221598297528));
#9600=CARTESIAN_POINT('Ctrl Pts',(3.38993834900092,-0.0965964897647501,
59.7281893491998));
#9601=CARTESIAN_POINT('Ctrl Pts',(3.38974396269868,0.00639764393193157,
59.7342188686468));
#9602=CARTESIAN_POINT('Ctrl Pts',(3.38954934829926,0.10951263321651,59.7402554632649));
#9603=CARTESIAN_POINT('Ctrl Pts',(3.38464543380326,0.212554688382857,59.746292057883));
#9604=CARTESIAN_POINT('Ctrl Pts',(3.37507651961816,0.315061183299604,59.7523286525011));
#9605=CARTESIAN_POINT('Ctrl Pts',(3.36550181885814,0.417629666598875,59.7583688976073));
#9606=CARTESIAN_POINT('Ctrl Pts',(3.3512565639643,0.519661513581867,59.7644091427135));
#9607=CARTESIAN_POINT('Ctrl Pts',(3.33243646798291,0.620703028313545,59.7704493878197));
#9608=CARTESIAN_POINT('Ctrl Pts',(3.31358238495012,0.721927013057994,59.7765005409531));
#9609=CARTESIAN_POINT('Ctrl Pts',(3.29013705966018,0.822156669244242,59.7825516940866));
#9610=CARTESIAN_POINT('Ctrl Pts',(3.26224653946451,0.920951995628335,59.7886028472201));
#9611=CARTESIAN_POINT('Ctrl Pts',(3.2389792621021,1.00337061833462,59.7936509372999));
#9612=CARTESIAN_POINT('Ctrl Pts',(3.21261929588641,1.08479119739988,59.7986990273796));
#9613=CARTESIAN_POINT('Ctrl Pts',(3.18327663589853,1.16496992314933,59.8037471174594));
#9614=CARTESIAN_POINT('Ctrl Pts',(3.14686255675042,1.26447127942173,59.8100117693957));
#9615=CARTESIAN_POINT('Ctrl Pts',(3.10572884959804,1.36240134727722,59.8162764213321));
#9616=CARTESIAN_POINT('Ctrl Pts',(3.06002946255804,1.45829515214745,59.8225410732684));
#9617=CARTESIAN_POINT('Ctrl Pts',(3.01439608204426,1.55405045150688,59.8287966767702));
#9618=CARTESIAN_POINT('Ctrl Pts',(2.96421031748651,1.6477749831512,59.8350522802721));
#9619=CARTESIAN_POINT('Ctrl Pts',(2.90967481768643,1.73902200038454,59.8413078837739));
#9620=CARTESIAN_POINT('Ctrl Pts',(2.85520568671812,1.83015797145604,59.8475558743062));
#9621=CARTESIAN_POINT('Ctrl Pts',(2.79639756218108,1.91882208860135,59.8538038648385));
#9622=CARTESIAN_POINT('Ctrl Pts',(2.73349955967788,2.00459103553339,59.8600518553708));
#9623=CARTESIAN_POINT('Ctrl Pts',(2.67067421049986,2.09026091096962,59.8662926288649));
#9624=CARTESIAN_POINT('Ctrl Pts',(2.60376863072127,2.17304195745685,59.872533402359));
#9625=CARTESIAN_POINT('Ctrl Pts',(2.53307546014354,2.25253940603014,59.8787741758531));
#9626=CARTESIAN_POINT('Ctrl Pts',(2.46243000911888,2.3319831919556,59.8850107366783));
#9627=CARTESIAN_POINT('Ctrl Pts',(2.38800232095185,2.40814749359993,59.8912472975035));
#9628=CARTESIAN_POINT('Ctrl Pts',(2.3101254528726,2.48067036393193,59.8974838583287));
#9629=CARTESIAN_POINT('Ctrl Pts',(2.23228512686462,2.55315920444273,59.9037174927798));
#9630=CARTESIAN_POINT('Ctrl Pts',(2.15099913524756,2.62200974333339,59.9099511272309));
#9631=CARTESIAN_POINT('Ctrl Pts',(2.06663715137858,2.68689708530897,59.9161847616819));
#9632=CARTESIAN_POINT('Ctrl Pts',(1.9822974027976,2.75176732492789,59.922416753134));
#9633=CARTESIAN_POINT('Ctrl Pts',(1.89488359359858,2.81267620483484,59.9286487445861));
#9634=CARTESIAN_POINT('Ctrl Pts',(1.80479776397003,2.86933966160662,59.9348807360381));
#9635=CARTESIAN_POINT('Ctrl Pts',(1.71469299596977,2.92601503050276,59.941114037616));
#9636=CARTESIAN_POINT('Ctrl Pts',(1.62191542118583,2.97844297598582,59.9473473391939));
#9637=CARTESIAN_POINT('Ctrl Pts',(1.52689515218141,3.02638336248812,59.9535806407717));
#9638=CARTESIAN_POINT('Ctrl Pts',(1.43186603238507,3.07432821446279,59.9598145229589));
#9639=CARTESIAN_POINT('Ctrl Pts',(1.33459416225473,3.11778450052887,59.9660484051461));
#9640=CARTESIAN_POINT('Ctrl Pts',(1.23553234644241,3.15655902580555,59.9722822873333));
#9641=CARTESIAN_POINT('Ctrl Pts',(1.13640492145646,3.19535923165896,59.9785202982543));
#9642=CARTESIAN_POINT('Ctrl Pts',(1.03548555781407,3.22947134348404,59.9847583091752));
#9643=CARTESIAN_POINT('Ctrl Pts',(0.933245001729504,3.25875111495906,59.9909963200961));
#9644=CARTESIAN_POINT('Ctrl Pts',(0.884055110280037,3.27283817429909,59.9939975467307));
#9645=CARTESIAN_POINT('Ctrl Pts',(0.834559611961812,3.28580740796592,59.9969987733654));
#9646=CARTESIAN_POINT('Ctrl Pts',(0.784811935329691,3.29764693208113,60.));
#9647=CARTESIAN_POINT('',(-3.37882581077538,0.271921317549902,59.9999963691758));
#9648=CARTESIAN_POINT('Origin',(0.,0.,60.));
#9649=CARTESIAN_POINT('',(-3.38974910170284,-0.00246779350202193,58.7660178032823));
#9650=CARTESIAN_POINT('Ctrl Pts',(-3.37882581077538,0.271921317549902,59.9999963691758));
#9651=CARTESIAN_POINT('Ctrl Pts',(-3.3705827143447,0.374347957842939,59.9939311509688));
#9652=CARTESIAN_POINT('Ctrl Pts',(-3.35766337532631,0.476579186057627,59.9878659327618));
#9653=CARTESIAN_POINT('Ctrl Pts',(-3.34008176227551,0.578151263783581,59.9818007145547));
#9654=CARTESIAN_POINT('Ctrl Pts',(-3.32252284426811,0.679592228243256,59.9757433255719));
#9655=CARTESIAN_POINT('Ctrl Pts',(-3.30031368710692,0.780375309900067,59.9696859365891));
#9656=CARTESIAN_POINT('Ctrl Pts',(-3.27352015539963,0.88004025742712,59.9636285476062));
#9657=CARTESIAN_POINT('Ctrl Pts',(-3.24569321907837,0.983549200503179,59.9573375300823));
#9658=CARTESIAN_POINT('Ctrl Pts',(-3.2129211553574,1.08585154404973,59.9510465125584));
#9659=CARTESIAN_POINT('Ctrl Pts',(-3.17533659756997,1.18644112986391,59.9447554950345));
#9660=CARTESIAN_POINT('Ctrl Pts',(-3.13920831724097,1.28313320151276,59.938708233658));
#9661=CARTESIAN_POINT('Ctrl Pts',(-3.09863371580969,1.37824232821105,59.9326609722816));
#9662=CARTESIAN_POINT('Ctrl Pts',(-3.05378153165466,1.4713338912106,59.9266137109051));
#9663=CARTESIAN_POINT('Ctrl Pts',(-3.00894339869995,1.5643962906761,59.9205683440023));
#9664=CARTESIAN_POINT('Ctrl Pts',(-2.95983053393135,1.6554419922977,59.9145229770995));
#9665=CARTESIAN_POINT('Ctrl Pts',(-2.90665925565672,1.74405763494362,59.9084776101967));
#9666=CARTESIAN_POINT('Ctrl Pts',(-2.85349042996258,1.8326691901009,59.9024325221428));
#9667=CARTESIAN_POINT('Ctrl Pts',(-2.79626378655923,1.91885053782882,59.8963874340888));
#9668=CARTESIAN_POINT('Ctrl Pts',(-2.73524041089657,2.00221501270428,59.8903423460348));
#9669=CARTESIAN_POINT('Ctrl Pts',(-2.67420354727771,2.08559791357424,59.8842959218391));
#9670=CARTESIAN_POINT('Ctrl Pts',(-2.60936854071464,2.16616235540417,59.8782494976433));
#9671=CARTESIAN_POINT('Ctrl Pts',(-2.54103779588299,2.24355342757735,59.8722030734475));
#9672=CARTESIAN_POINT('Ctrl Pts',(-2.47263591117817,2.32102507242794,59.8661503542545));
#9673=CARTESIAN_POINT('Ctrl Pts',(-2.4007313125139,2.39531642933056,59.8600976350615));
#9674=CARTESIAN_POINT('Ctrl Pts',(-2.32566426496307,2.46610843013315,59.8540449158685));
#9675=CARTESIAN_POINT('Ctrl Pts',(-2.25055077251949,2.53694423080521,59.8479884517847));
#9676=CARTESIAN_POINT('Ctrl Pts',(-2.17227126463747,2.60427608378036,59.8419319877009));
#9677=CARTESIAN_POINT('Ctrl Pts',(-2.09119865285149,2.66782556716366,59.8358755236172));
#9678=CARTESIAN_POINT('Ctrl Pts',(-2.01000848889477,2.73146719485508,59.8298102778933));
#9679=CARTESIAN_POINT('Ctrl Pts',(-1.92601749196678,2.79131525928248,59.8237450321693));
#9680=CARTESIAN_POINT('Ctrl Pts',(-1.83962685362631,2.84713506913826,59.8176797864454));
#9681=CARTESIAN_POINT('Ctrl Pts',(-1.81571829597486,2.86258316823403,59.8160012333077));
#9682=CARTESIAN_POINT('Ctrl Pts',(-1.79162608731277,2.87772301716914,59.8143226801699));
#9683=CARTESIAN_POINT('Ctrl Pts',(-1.76735903007707,2.89255027982316,59.8126441270322));
#9684=CARTESIAN_POINT('Ctrl Pts',(-1.67896520419358,2.94655923775484,59.8065299232227));
#9685=CARTESIAN_POINT('Ctrl Pts',(-1.58795127391211,2.99659951709765,59.8004157194132));
#9686=CARTESIAN_POINT('Ctrl Pts',(-1.49470788425146,3.04240914461821,59.7943015156036));
#9687=CARTESIAN_POINT('Ctrl Pts',(-1.40158320174281,3.08816045239689,59.788195095721));
#9688=CARTESIAN_POINT('Ctrl Pts',(-1.30623508230095,3.12969163111811,59.7820886758383));
#9689=CARTESIAN_POINT('Ctrl Pts',(-1.20908150021065,3.16678496086305,59.7759822559556));
#9690=CARTESIAN_POINT('Ctrl Pts',(-1.11202415897218,3.20384154575951,59.7698818851247));
#9691=CARTESIAN_POINT('Ctrl Pts',(-1.01316530769847,3.23646887353432,59.7637815142938));
#9692=CARTESIAN_POINT('Ctrl Pts',(-0.912945011732789,3.26449635748797,59.7576811434629));
#9693=CARTESIAN_POINT('Ctrl Pts',(-0.81279147236823,3.29250517237316,59.7515848360806));
#9694=CARTESIAN_POINT('Ctrl Pts',(-0.711278700560812,3.31592012224861,59.7454885286984));
#9695=CARTESIAN_POINT('Ctrl Pts',(-0.608863371791357,3.33461998689369,59.7393922213161));
#9696=CARTESIAN_POINT('Ctrl Pts',(-0.506483110413252,3.35331344863522,59.7332980013322));
#9697=CARTESIAN_POINT('Ctrl Pts',(-0.403201324673627,3.36729495786349,59.7272037813484));
#9698=CARTESIAN_POINT('Ctrl Pts',(-0.299485598072089,3.37649425277867,59.7211095613645));
#9699=CARTESIAN_POINT('Ctrl Pts',(-0.195778851751454,3.38569275116805,59.715015869052));
#9700=CARTESIAN_POINT('Ctrl Pts',(-0.0916386632773638,3.39010982122857,
59.7089221767394));
#9701=CARTESIAN_POINT('Ctrl Pts',(0.0124624203631624,3.3897270908701,59.7028284844268));
#9702=CARTESIAN_POINT('Ctrl Pts',(0.116581120678082,3.38934429574347,59.6967337608992));
#9703=CARTESIAN_POINT('Ctrl Pts',(0.220660277360656,3.38416008768294,59.6906390373717));
#9704=CARTESIAN_POINT('Ctrl Pts',(0.324228393133874,3.37420820513285,59.6845443138442));
#9705=CARTESIAN_POINT('Ctrl Pts',(0.427904615032644,3.36424593464186,59.6784432285426));
#9706=CARTESIAN_POINT('Ctrl Pts',(0.531068306318182,3.34950609234175,59.6723421432411));
#9707=CARTESIAN_POINT('Ctrl Pts',(0.633254156655067,3.33007420871954,59.6662410579395));
#9708=CARTESIAN_POINT('Ctrl Pts',(0.735496284187732,3.31063162330334,59.6601366125644));
#9709=CARTESIAN_POINT('Ctrl Pts',(0.836759083943799,3.28649194763691,59.6540321671893));
#9710=CARTESIAN_POINT('Ctrl Pts',(0.936590396338981,3.25779119834062,59.6479277218143));
#9711=CARTESIAN_POINT('Ctrl Pts',(1.03658141668464,3.22904453421322,59.6418135106809));
#9712=CARTESIAN_POINT('Ctrl Pts',(1.13513597172525,3.19572235713619,59.6356992995476));
#9713=CARTESIAN_POINT('Ctrl Pts',(1.23181973666577,3.15800968948176,59.6295850884143));
#9714=CARTESIAN_POINT('Ctrl Pts',(1.30136430405099,3.13088299288918,59.62518714044));
#9715=CARTESIAN_POINT('Ctrl Pts',(1.36994134546611,3.10148571668628,59.6207891924658));
#9716=CARTESIAN_POINT('Ctrl Pts',(1.43739728720325,3.06990131783429,59.6163912444915));
#9717=CARTESIAN_POINT('Ctrl Pts',(1.53093592444134,3.02610441054166,59.6102927741482));
#9718=CARTESIAN_POINT('Ctrl Pts',(1.62263027937754,2.97795391002212,59.604194303805));
#9719=CARTESIAN_POINT('Ctrl Pts',(1.7120474884185,2.92562787447411,59.5980958334617));
#9720=CARTESIAN_POINT('Ctrl Pts',(1.80134670584262,2.87337088641264,59.5920054104327));
#9721=CARTESIAN_POINT('Ctrl Pts',(1.88837438447763,2.81694953136673,59.5859149874036));
#9722=CARTESIAN_POINT('Ctrl Pts',(1.97271919323224,2.75658920536832,59.5798245643746));
#9723=CARTESIAN_POINT('Ctrl Pts',(2.05697690872072,2.69629120659566,59.5737404302309));
#9724=CARTESIAN_POINT('Ctrl Pts',(2.13855691653878,2.63206257248482,59.5676562960872));
#9725=CARTESIAN_POINT('Ctrl Pts',(2.21707475798935,2.56417327417366,59.5615721619436));
#9726=CARTESIAN_POINT('Ctrl Pts',(2.2955363800184,2.49633258515955,59.5554923840901));
#9727=CARTESIAN_POINT('Ctrl Pts',(2.37093987270381,2.42483672341953,59.5494126062366));
#9728=CARTESIAN_POINT('Ctrl Pts',(2.44293259664658,2.3499968916451,59.5433328283831));
#9729=CARTESIAN_POINT('Ctrl Pts',(2.51489854712299,2.2751848921516,59.537255311546));
#9730=CARTESIAN_POINT('Ctrl Pts',(2.58345595319024,2.19703170245457,59.5311777947089));
#9731=CARTESIAN_POINT('Ctrl Pts',(2.64828849560439,2.11588589166558,59.5251002778718));
#9732=CARTESIAN_POINT('Ctrl Pts',(2.7131137731791,2.03474917370659,59.5190234420535));
#9733=CARTESIAN_POINT('Ctrl Pts',(2.7742147497887,1.95062083606934,59.5129466062352));
#9734=CARTESIAN_POINT('Ctrl Pts',(2.8313155254947,1.86388236152196,59.506869770417));
#9735=CARTESIAN_POINT('Ctrl Pts',(2.88842473940007,1.77713106899562,59.5007920365802));
#9736=CARTESIAN_POINT('Ctrl Pts',(2.94153234254682,1.6877692310256,59.4947143027435));
#9737=CARTESIAN_POINT('Ctrl Pts',(2.99040639390585,1.59620633433995,59.4886365689068));
#9738=CARTESIAN_POINT('Ctrl Pts',(3.03933077822348,1.50454914157369,59.4825525759138));
#9739=CARTESIAN_POINT('Ctrl Pts',(3.08401270199905,1.41068674191281,59.4764685829207));
#9740=CARTESIAN_POINT('Ctrl Pts',(3.12426678168413,1.31505214321147,59.4703845899277));
#9741=CARTESIAN_POINT('Ctrl Pts',(3.16454255151007,1.21936601363592,59.4642973186914));
#9742=CARTESIAN_POINT('Ctrl Pts',(3.20038557718903,1.1219061849542,59.4582100474552));
#9743=CARTESIAN_POINT('Ctrl Pts',(3.23165981215085,1.02312263244887,59.4521227762189));
#9744=CARTESIAN_POINT('Ctrl Pts',(3.26298442443984,0.924179956903502,59.4460256994524));
#9745=CARTESIAN_POINT('Ctrl Pts',(3.28972543462535,0.823909712182205,59.439928622686));
#9746=CARTESIAN_POINT('Ctrl Pts',(3.31179749576697,0.722774106849198,59.4338315459196));
#9747=CARTESIAN_POINT('Ctrl Pts',(3.32832108597023,0.647061952612234,59.4292671512633));
#9748=CARTESIAN_POINT('Ctrl Pts',(3.34222910857796,0.570865067973735,59.4247027566071));
#9749=CARTESIAN_POINT('Ctrl Pts',(3.35350482013033,0.494378886950759,59.4201383619509));
#9750=CARTESIAN_POINT('Ctrl Pts',(3.36858890646888,0.392059476517221,59.4140323417004));
#9751=CARTESIAN_POINT('Ctrl Pts',(3.37901099388049,0.288878871688489,59.4079263214499));
#9752=CARTESIAN_POINT('Ctrl Pts',(3.38468164869492,0.18529759709133,59.4018203011994));
#9753=CARTESIAN_POINT('Ctrl Pts',(3.39034491257526,0.0818513267220041,59.3957222393231));
#9754=CARTESIAN_POINT('Ctrl Pts',(3.39126903291786,-0.0219941523002653,
59.3896241774468));
#9755=CARTESIAN_POINT('Ctrl Pts',(3.38741596139382,-0.125770294562564,59.3835261155706));
#9756=CARTESIAN_POINT('Ctrl Pts',(3.3835668141757,-0.229440742101569,59.3774342644953));
#9757=CARTESIAN_POINT('Ctrl Pts',(3.37495016640692,-0.333041568791544,59.37134241342));
#9758=CARTESIAN_POINT('Ctrl Pts',(3.36157997946325,-0.436102171711884,59.3652505623446));
#9759=CARTESIAN_POINT('Ctrl Pts',(3.34821916601326,-0.539090521498238,59.3591629821092));
#9760=CARTESIAN_POINT('Ctrl Pts',(3.33011149556153,-0.641538978427963,59.3530754018738));
#9761=CARTESIAN_POINT('Ctrl Pts',(3.30732286692106,-0.742980831812695,59.3469878216383));
#9762=CARTESIAN_POINT('Ctrl Pts',(3.28454251641038,-0.844385835730001,59.3409024527593));
#9763=CARTESIAN_POINT('Ctrl Pts',(3.25708468084369,-0.944784546674081,59.3348170838802));
#9764=CARTESIAN_POINT('Ctrl Pts',(3.22506644606084,-1.04372002040419,59.3287317150011));
#9765=CARTESIAN_POINT('Ctrl Pts',(3.19305158275161,-1.14264507637259,59.3226469869026));
#9766=CARTESIAN_POINT('Ctrl Pts',(3.15647740670422,-1.24010679528403,59.316562258804));
#9767=CARTESIAN_POINT('Ctrl Pts',(3.11551073277267,-1.33566385609489,59.3104775307055));
#9768=CARTESIAN_POINT('Ctrl Pts',(3.07453780506184,-1.4312355041961,59.304391873741));
#9769=CARTESIAN_POINT('Ctrl Pts',(3.02917121550791,-1.52490152402909,59.2983062167766));
#9770=CARTESIAN_POINT('Ctrl Pts',(2.9796253644156,-1.6162418600665,59.2922205598121));
#9771=CARTESIAN_POINT('Ctrl Pts',(2.93002855914626,-1.70767613276156,59.2861286442077));
#9772=CARTESIAN_POINT('Ctrl Pts',(2.87624411312226,-1.79677956922563,59.2800367286033));
#9773=CARTESIAN_POINT('Ctrl Pts',(2.8185317074462,-1.88315800628104,59.2739448129989));
#9774=CARTESIAN_POINT('Ctrl Pts',(2.76078813751174,-1.96958308703293,59.2678496078066));
#9775=CARTESIAN_POINT('Ctrl Pts',(2.69911263613288,-2.05327989343153,59.2617544026143));
#9776=CARTESIAN_POINT('Ctrl Pts',(2.63380624001871,-2.13388606831257,59.255659197422));
#9777=CARTESIAN_POINT('Ctrl Pts',(2.56839544543498,-2.21462109981097,59.249554248466));
#9778=CARTESIAN_POINT('Ctrl Pts',(2.4993424454928,-2.29225531125116,59.2434492995099));
#9779=CARTESIAN_POINT('Ctrl Pts',(2.42698643575381,-2.36646189556625,59.2373443505539));
#9780=CARTESIAN_POINT('Ctrl Pts',(2.37381480846378,-2.42099343839043,59.2328580601727));
#9781=CARTESIAN_POINT('Ctrl Pts',(2.31886027471514,-2.47367475259768,59.2283717697915));
#9782=CARTESIAN_POINT('Ctrl Pts',(2.26226850542853,-2.52439027724442,59.2238854794102));
#9783=CARTESIAN_POINT('Ctrl Pts',(2.18524772879517,-2.59341354944284,59.2177796874599));
#9784=CARTESIAN_POINT('Ctrl Pts',(2.10493719415618,-2.65902336062621,59.2116738955096));
#9785=CARTESIAN_POINT('Ctrl Pts',(2.02167171369199,-2.72089113059632,59.2055681035593));
#9786=CARTESIAN_POINT('Ctrl Pts',(1.93851454729975,-2.78267842123632,59.1994702541944));
#9787=CARTESIAN_POINT('Ctrl Pts',(1.85241041719165,-2.8407330957871,59.1933724048295));
#9788=CARTESIAN_POINT('Ctrl Pts',(1.7637291654895,-2.8947650152131,59.1872745554646));
#9789=CARTESIAN_POINT('Ctrl Pts',(1.67513800473733,-2.94874204381543,59.1811829008819));
#9790=CARTESIAN_POINT('Ctrl Pts',(1.58397529153529,-2.99870422304866,59.1750912462992));
#9791=CARTESIAN_POINT('Ctrl Pts',(1.49064126746975,-3.04440366479483,59.1689995917165));
#9792=CARTESIAN_POINT('Ctrl Pts',(1.39737229531499,-3.09007125496236,59.1629121828928));
#9793=CARTESIAN_POINT('Ctrl Pts',(1.30193540428378,-3.13148182870483,59.1568247740691));
#9794=CARTESIAN_POINT('Ctrl Pts',(1.20475623387012,-3.1684329690639,59.1507373652453));
#9795=CARTESIAN_POINT('Ctrl Pts',(1.10761211796475,-3.20537078039319,59.1446521522741));
#9796=CARTESIAN_POINT('Ctrl Pts',(1.00872737056014,-3.23785220392031,59.1385669393029));
#9797=CARTESIAN_POINT('Ctrl Pts',(0.90854771262464,-3.26572290869641,59.1324817263317));
#9798=CARTESIAN_POINT('Ctrl Pts',(0.808378344346053,-3.2935907508156,59.1263971383851));
#9799=CARTESIAN_POINT('Ctrl Pts',(0.706914741463906,-3.31684870154608,59.1203125504385));
#9800=CARTESIAN_POINT('Ctrl Pts',(0.604617016221556,-3.33539252955261,59.1142279624919));
#9801=CARTESIAN_POINT('Ctrl Pts',(0.502303404986299,-3.35393923726266,59.108142429659));
#9802=CARTESIAN_POINT('Ctrl Pts',(0.399155834257855,-3.36777029158176,59.1020568968261));
#9803=CARTESIAN_POINT('Ctrl Pts',(0.295642918161283,-3.37683288414471,59.0959713639931));
#9804=CARTESIAN_POINT('Ctrl Pts',(0.192023105992799,-3.38590483549672,59.0898795467314));
#9805=CARTESIAN_POINT('Ctrl Pts',(0.0880376212267635,-3.39019845399246,
59.0837877294696));
#9806=CARTESIAN_POINT('Ctrl Pts',(-0.0158415490729636,-3.38971298310387,
59.0776959122079));
#9807=CARTESIAN_POINT('Ctrl Pts',(-0.119777056577213,-3.38922724892793,
59.0716007911466));
#9808=CARTESIAN_POINT('Ctrl Pts',(-0.223605708239737,-3.38395728413858,
59.0655056700853));
#9809=CARTESIAN_POINT('Ctrl Pts',(-0.326859245018531,-3.37395437083045,
59.059410549024));
#9810=CARTESIAN_POINT('Ctrl Pts',(-0.43027825514994,-3.36393542692761,59.0533056599669));
#9811=CARTESIAN_POINT('Ctrl Pts',(-0.533119886389554,-3.3491684437396,59.0472007709097));
#9812=CARTESIAN_POINT('Ctrl Pts',(-0.634924492216723,-3.32975613997232,
59.0410958818526));
#9813=CARTESIAN_POINT('Ctrl Pts',(-0.709762020412863,-3.31548597195062,
59.0366081201916));
#9814=CARTESIAN_POINT('Ctrl Pts',(-0.784039355673478,-3.29870661602957,
59.0321203585306));
#9815=CARTESIAN_POINT('Ctrl Pts',(-0.857579600464567,-3.27947591718052,
59.0276325968696));
#9816=CARTESIAN_POINT('Ctrl Pts',(-0.957605192774021,-3.2533193270255,59.0215285783208));
#9817=CARTESIAN_POINT('Ctrl Pts',(-1.05660029666248,-3.22253858110059,59.015424559772));
#9818=CARTESIAN_POINT('Ctrl Pts',(-1.15410634620905,-3.18723133834681,59.0093205412232));
#9819=CARTESIAN_POINT('Ctrl Pts',(-1.25148501946813,-3.15197021894152,59.0032244966127));
#9820=CARTESIAN_POINT('Ctrl Pts',(-1.34737810717236,-3.11219450292162,58.9971284520022));
#9821=CARTESIAN_POINT('Ctrl Pts',(-1.44133974546717,-3.06805228127498,58.9910324073917));
#9822=CARTESIAN_POINT('Ctrl Pts',(-1.53520545770926,-3.0239551247119,58.9849425862731));
#9823=CARTESIAN_POINT('Ctrl Pts',(-1.62714325687212,-2.97550050789795,58.9788527651545));
#9824=CARTESIAN_POINT('Ctrl Pts',(-1.71672571818852,-2.92288519634455,58.9727629440359));
#9825=CARTESIAN_POINT('Ctrl Pts',(-1.80624520006417,-2.87030687509983,58.9666774042635));
#9826=CARTESIAN_POINT('Ctrl Pts',(-1.89341226959328,-2.81357389188496,58.9605918644911));
#9827=CARTESIAN_POINT('Ctrl Pts',(-1.9778233931322,-2.75292929224109,58.9545063247187));
#9828=CARTESIAN_POINT('Ctrl Pts',(-2.06220376487716,-2.69230678601518,58.9484230019677));
#9829=CARTESIAN_POINT('Ctrl Pts',(-2.14382983944766,-2.62777574473887,58.9423396792167));
#9830=CARTESIAN_POINT('Ctrl Pts',(-2.22232709072012,-2.55962250426727,58.9362563564656));
#9831=CARTESIAN_POINT('Ctrl Pts',(-2.30081603298364,-2.49147647788119,58.9301736776401));
#9832=CARTESIAN_POINT('Ctrl Pts',(-2.37617648789699,-2.41970929495399,58.9240909988146));
#9833=CARTESIAN_POINT('Ctrl Pts',(-2.44806776033335,-2.34464694641144,58.9180083199891));
#9834=CARTESIAN_POINT('Ctrl Pts',(-2.51997000363706,-2.26957314308387,58.9119247129249));
#9835=CARTESIAN_POINT('Ctrl Pts',(-2.58840171704246,-2.19120348373446,58.9058411058606));
#9836=CARTESIAN_POINT('Ctrl Pts',(-2.65306039369009,-2.10989943123671,58.8997574987964));
#9837=CARTESIAN_POINT('Ctrl Pts',(-2.71778571353709,-2.02851157927908,58.8936676214052));
#9838=CARTESIAN_POINT('Ctrl Pts',(-2.77872996416887,-1.94418362945578,58.8875777440141));
#9839=CARTESIAN_POINT('Ctrl Pts',(-2.83563218486111,-1.85730858359073,58.881487866623));
#9840=CARTESIAN_POINT('Ctrl Pts',(-2.89256517573887,-1.77038655957182,58.8753946960975));
#9841=CARTESIAN_POINT('Ctrl Pts',(-2.945451565345,-1.68091506381603,58.8693015255721));
#9842=CARTESIAN_POINT('Ctrl Pts',(-2.99407584872459,-1.58931270509744,58.8632083550466));
#9843=CARTESIAN_POINT('Ctrl Pts',(-3.04277809978119,-1.49756346456133,58.8571054142928));
#9844=CARTESIAN_POINT('Ctrl Pts',(-3.08720441007919,-1.4036769222985,58.851002473539));
#9845=CARTESIAN_POINT('Ctrl Pts',(-3.12718692467644,-1.30809288685196,58.8448995327852));
#9846=CARTESIAN_POINT('Ctrl Pts',(-3.15671128899992,-1.23751058570211,58.8403929266331));
#9847=CARTESIAN_POINT('Ctrl Pts',(-3.18381354062492,-1.16600310139847,58.835886320481));
#9848=CARTESIAN_POINT('Ctrl Pts',(-3.20844371669675,-1.09375224767274,58.831379714329));
#9849=CARTESIAN_POINT('Ctrl Pts',(-3.24747463784324,-0.97925784185478,58.8242381904987));
#9850=CARTESIAN_POINT('Ctrl Pts',(-3.28040259243278,-0.86258554788198,58.8170966666684));
#9851=CARTESIAN_POINT('Ctrl Pts',(-3.30701686360868,-0.744341673096319,
58.8099551428382));
#9852=CARTESIAN_POINT('Ctrl Pts',(-3.3343070306534,-0.623094877586172,58.8026322529122));
#9853=CARTESIAN_POINT('Ctrl Pts',(-3.35495839545225,-0.50019566529006,58.7953093629862));
#9854=CARTESIAN_POINT('Ctrl Pts',(-3.36879618663337,-0.376320761351867,
58.7879864730602));
#9855=CARTESIAN_POINT('Ctrl Pts',(-3.3826339778145,-0.252445857413681,58.7806635831342));
#9856=CARTESIAN_POINT('Ctrl Pts',(-3.389658006751,-0.127595374439921,58.7733406932083));
#9857=CARTESIAN_POINT('Ctrl Pts',(-3.38974910170284,-0.00246779350203549,
58.7660178032823));
#9858=CARTESIAN_POINT('Ctrl Pts',(-3.38974910170325,-0.00246779294397778,
58.7660178032496));
#9859=CARTESIAN_POINT('Ctrl Pts',(-3.38978279105707,0.0438077493895984,
58.7633096017465));
#9860=CARTESIAN_POINT('Ctrl Pts',(-3.38886871311492,0.0900941169352991,
58.7606014002435));
#9861=CARTESIAN_POINT('Ctrl Pts',(-3.38700661857411,0.136349654327206,58.7578931987404));
#9862=CARTESIAN_POINT('Origin',(0.,0.,0.));
#9863=CARTESIAN_POINT('',(-3.38700661857411,0.136349654327205,57.5081828107941));
#9864=CARTESIAN_POINT('',(-3.38700661857411,0.136349654327218,57.8510343478015));
#9865=CARTESIAN_POINT('',(-3.38700661857411,0.136349654327212,0.));
#9866=CARTESIAN_POINT('',(-3.39333846869908,0.00164290954011615,57.8589835450503));
#9867=CARTESIAN_POINT('Ctrl Pts',(-3.38700661857411,0.136349654327218,57.8510343478015));
#9868=CARTESIAN_POINT('Ctrl Pts',(-3.38881233164404,0.0914946662507057,
57.8536836307845));
#9869=CARTESIAN_POINT('Ctrl Pts',(-3.38972753681572,0.0465908495261081,
57.8563329137674));
#9870=CARTESIAN_POINT('Ctrl Pts',(-3.38974959155796,0.00166404104890279,
57.8589821967504));
#9871=CARTESIAN_POINT('Ctrl Pts',(-3.39400293157413,0.00163899714564557,
57.8589837946813));
#9872=CARTESIAN_POINT('Ctrl Pts',(-3.38782206386631,-1.00856606823546,57.9184795879854));
#9873=CARTESIAN_POINT('Ctrl Pts',(-2.37784689341624,-3.14025136115915,58.0433930088032));
#9874=CARTESIAN_POINT('Ctrl Pts',(1.22855586861976,-3.7978891647466,58.2337240571342));
#9875=CARTESIAN_POINT('Ctrl Pts',(3.84552201587359,-1.07034770082512,58.4299769396749));
#9876=CARTESIAN_POINT('Ctrl Pts',(3.01399994759664,2.6171086526788,58.6262298222154));
#9877=CARTESIAN_POINT('Ctrl Pts',(-0.520106131442002,3.9575204291085,58.8224827047562));
#9878=CARTESIAN_POINT('Ctrl Pts',(-2.99442679320825,2.17678596204204,58.9807570033809));
#9879=CARTESIAN_POINT('Ctrl Pts',(-3.36535655531616,0.604978518233871,59.0736136744922));
#9880=CARTESIAN_POINT('Ctrl Pts',(-3.3822802839685,0.136179104839289,59.1010527180899));
#9881=CARTESIAN_POINT('',(-3.38974888547239,0.00274880677970033,57.5160178032002));
#9882=CARTESIAN_POINT('Ctrl Pts',(-3.38700661857411,0.136349654327206,58.7578931987404));
#9883=CARTESIAN_POINT('Ctrl Pts',(-3.38282665423314,0.240182457997669,58.7518139232455));
#9884=CARTESIAN_POINT('Ctrl Pts',(-3.37386618535491,0.343859661797899,58.7457346477506));
#9885=CARTESIAN_POINT('Ctrl Pts',(-3.36016005561475,0.446911023752028,58.7396553722557));
#9886=CARTESIAN_POINT('Ctrl Pts',(-3.34645455965355,0.549957620554638,58.7335763778699));
#9887=CARTESIAN_POINT('Ctrl Pts',(-3.3280038956582,0.652378009419878,58.7274973834841));
#9888=CARTESIAN_POINT('Ctrl Pts',(-3.30489460670436,0.753708631419604,58.7214183890982));
#9889=CARTESIAN_POINT('Ctrl Pts',(-3.28178041472971,0.855060752399686,58.7153381049524));
#9890=CARTESIAN_POINT('Ctrl Pts',(-3.25400572848584,0.955322230365361,58.7092578208066));
#9891=CARTESIAN_POINT('Ctrl Pts',(-3.22170766277606,1.05404212349887,58.7031775366608));
#9892=CARTESIAN_POINT('Ctrl Pts',(-3.18937349363719,1.15287236771948,58.6970904558507));
#9893=CARTESIAN_POINT('Ctrl Pts',(-3.15250598156084,1.25015717926762,58.6910033750407));
#9894=CARTESIAN_POINT('Ctrl Pts',(-3.11129136442251,1.34546315749258,58.6849162942307));
#9895=CARTESIAN_POINT('Ctrl Pts',(-3.07005235229948,1.44082554744819,58.6788256104697));
#9896=CARTESIAN_POINT('Ctrl Pts',(-3.02446129818378,1.53420638755629,58.6727349267087));
#9897=CARTESIAN_POINT('Ctrl Pts',(-2.97475071023258,1.62519638027862,58.6666442429478));
#9898=CARTESIAN_POINT('Ctrl Pts',(-2.92495694619027,1.7163386180706,58.6605433682136));
#9899=CARTESIAN_POINT('Ctrl Pts',(-2.87103010251823,1.8050816529281,58.6544424934795));
#9900=CARTESIAN_POINT('Ctrl Pts',(-2.81324647326607,1.89104451115145,58.6483416187454));
#9901=CARTESIAN_POINT('Ctrl Pts',(-2.77152577017277,1.95311106756895,58.6439366897597));
#9902=CARTESIAN_POINT('Ctrl Pts',(-2.72779540413566,2.01372892167687,58.639531760774));
#9903=CARTESIAN_POINT('Ctrl Pts',(-2.68217193456761,2.07276597229833,58.6351268317883));
#9904=CARTESIAN_POINT('Ctrl Pts',(-2.61894095240248,2.15458725266719,58.6290219040226));
#9905=CARTESIAN_POINT('Ctrl Pts',(-2.55185713164622,2.23364896070159,58.6229169762569));
#9906=CARTESIAN_POINT('Ctrl Pts',(-2.48119001523206,2.30956731246628,58.6168120484912));
#9907=CARTESIAN_POINT('Ctrl Pts',(-2.4106150404825,2.38538667556893,58.6107150808381));
#9908=CARTESIAN_POINT('Ctrl Pts',(-2.33646634760533,2.45807052070856,58.6046181131851));
#9909=CARTESIAN_POINT('Ctrl Pts',(-2.25905490583226,2.52726650651157,58.598521145532));
#9910=CARTESIAN_POINT('Ctrl Pts',(-2.18172232341004,2.59639200208217,58.5924303888847));
#9911=CARTESIAN_POINT('Ctrl Pts',(-2.10113391854465,2.66203642071304,58.5863396322374));
#9912=CARTESIAN_POINT('Ctrl Pts',(-2.01763822366384,2.72388345215258,58.5802488755901));
#9913=CARTESIAN_POINT('Ctrl Pts',(-1.93420101584568,2.78568716098478,58.5741623853959));
#9914=CARTESIAN_POINT('Ctrl Pts',(-1.84786091017546,2.84369851883857,58.5680758952017));
#9915=CARTESIAN_POINT('Ctrl Pts',(-1.75899966580321,2.89764132324969,58.5619894050075));
#9916=CARTESIAN_POINT('Ctrl Pts',(-1.67017066097764,2.95156455679419,58.555905123039));
#9917=CARTESIAN_POINT('Ctrl Pts',(-1.5788227002225,3.00142194926522,58.5498208410706));
#9918=CARTESIAN_POINT('Ctrl Pts',(-1.4853660154705,3.04698094227471,58.5437365591021));
#9919=CARTESIAN_POINT('Ctrl Pts',(-1.39191910427867,3.09253517079293,58.5376529134187));
#9920=CARTESIAN_POINT('Ctrl Pts',(-1.29636429164641,3.13379170662789,58.5315692677353));
#9921=CARTESIAN_POINT('Ctrl Pts',(-1.19913505020843,3.17056464905884,58.5254856220519));
#9922=CARTESIAN_POINT('Ctrl Pts',(-1.10189086985465,3.20734324151733,58.5194010416387));
#9923=CARTESIAN_POINT('Ctrl Pts',(-1.00297214914811,3.23963672076132,58.5133164612255));
#9924=CARTESIAN_POINT('Ctrl Pts',(-0.902830048011686,3.26730821425026,58.5072318808123));
#9925=CARTESIAN_POINT('Ctrl Pts',(-0.802584679727155,3.29500824275279,58.5011410259425));
#9926=CARTESIAN_POINT('Ctrl Pts',(-0.701113824220023,3.31807665342246,58.4950501710727));
#9927=CARTESIAN_POINT('Ctrl Pts',(-0.598881396724873,3.33642715118386,58.4889593162029));
#9928=CARTESIAN_POINT('Ctrl Pts',(-0.496593632920135,3.35478758169214,58.4828651644787));
#9929=CARTESIAN_POINT('Ctrl Pts',(-0.393543899527129,3.36842495639041,58.4767710127545));
#9930=CARTESIAN_POINT('Ctrl Pts',(-0.290201880048848,3.37730483245385,58.4706768610302));
#9931=CARTESIAN_POINT('Ctrl Pts',(-0.186694246128748,3.38619893927961,58.4645729429057));
#9932=CARTESIAN_POINT('Ctrl Pts',(-0.0828938174908368,3.39032030050129,
58.4584690247811));
#9933=CARTESIAN_POINT('Ctrl Pts',(0.0207288678506607,3.38968661922273,58.4523651066565));
#9934=CARTESIAN_POINT('Ctrl Pts',(0.0970727249459632,3.38921975549676,58.4478680541869));
#9935=CARTESIAN_POINT('Ctrl Pts',(0.173320104370365,3.38617295840839,58.4433710017173));
#9936=CARTESIAN_POINT('Ctrl Pts',(0.249285366297637,3.38057123407418,58.4388739492476));
#9937=CARTESIAN_POINT('Ctrl Pts',(0.352408029035052,3.37296690658806,58.4327692111954));
#9938=CARTESIAN_POINT('Ctrl Pts',(0.455354476334407,3.36062703606681,58.4266644731431));
#9939=CARTESIAN_POINT('Ctrl Pts',(0.557655937346654,3.34356470223653,58.4205597350908));
#9940=CARTESIAN_POINT('Ctrl Pts',(0.659823944337117,3.32652462651525,58.4144629607747));
#9941=CARTESIAN_POINT('Ctrl Pts',(0.761348219898703,3.30477440501136,58.4083661864587));
#9942=CARTESIAN_POINT('Ctrl Pts',(0.861763362557287,3.27837901552794,58.4022694121426));
#9943=CARTESIAN_POINT('Ctrl Pts',(0.962076153657685,3.2520105304453,58.3961788521716));
#9944=CARTESIAN_POINT('Ctrl Pts',(1.06128164893468,3.22100640084455,58.3900882922006));
#9945=CARTESIAN_POINT('Ctrl Pts',(1.15892377503534,3.18548281209581,58.3839977322296));
#9946=CARTESIAN_POINT('Ctrl Pts',(1.25649743506835,3.14998413227243,58.3779114429224));
#9947=CARTESIAN_POINT('Ctrl Pts',(1.35250950557861,3.10997244097856,58.3718251536152));
#9948=CARTESIAN_POINT('Ctrl Pts',(1.44651903453195,3.06561376321884,58.365738864308));
#9949=CARTESIAN_POINT('Ctrl Pts',(1.54049441616414,3.02127119797486,58.3596547857392));
#9950=CARTESIAN_POINT('Ctrl Pts',(1.6324683159849,2.97258496663961,58.3535707071704));
#9951=CARTESIAN_POINT('Ctrl Pts',(1.7220204754936,2.91976891970594,58.3474866286016));
#9952=CARTESIAN_POINT('Ctrl Pts',(1.81156323605196,2.86695841608251,58.3414031885875));
#9953=CARTESIAN_POINT('Ctrl Pts',(1.8986843937914,2.81001917588827,58.3353197485733));
#9954=CARTESIAN_POINT('Ctrl Pts',(1.98298978407304,2.74921017362478,58.3292363085592));
#9955=CARTESIAN_POINT('Ctrl Pts',(2.06730809989726,2.68839184824035,58.3231519358436));
#9956=CARTESIAN_POINT('Ctrl Pts',(2.14880944403362,2.62370283195656,58.317067563128));
#9957=CARTESIAN_POINT('Ctrl Pts',(2.22713078689163,2.55544389893018,58.3109831904125));
#9958=CARTESIAN_POINT('Ctrl Pts',(2.30553287369099,2.48711459561795,58.3048925451252));
#9959=CARTESIAN_POINT('Ctrl Pts',(2.38074808968624,2.4152083071782,58.298801899838));
#9960=CARTESIAN_POINT('Ctrl Pts',(2.45244855371389,2.34006434823632,58.2927112545508));
#9961=CARTESIAN_POINT('Ctrl Pts',(2.52418781313072,2.26487973071333,58.2866173137625));
#9962=CARTESIAN_POINT('Ctrl Pts',(2.59240825199432,2.1864542755058,58.2805233729742));
#9963=CARTESIAN_POINT('Ctrl Pts',(2.65682205553713,2.10516071303629,58.2744294321859));
#9964=CARTESIAN_POINT('Ctrl Pts',(2.72133909036212,2.02373686733206,58.2683257250854));
#9965=CARTESIAN_POINT('Ctrl Pts',(2.78203705375953,1.93943607942494,58.2622220179848));
#9966=CARTESIAN_POINT('Ctrl Pts',(2.83867115315711,1.85266055896208,58.2561183108842));
#9967=CARTESIAN_POINT('Ctrl Pts',(2.88041650865635,1.78869776995535,58.2516192294918));
#9968=CARTESIAN_POINT('Ctrl Pts',(2.91995477631312,1.72339099862094,58.2471201480994));
#9969=CARTESIAN_POINT('Ctrl Pts',(2.95720429512956,1.65690911620622,58.242621066707));
#9970=CARTESIAN_POINT('Ctrl Pts',(3.007748760591,1.56669879091099,58.2365161914959));
#9971=CARTESIAN_POINT('Ctrl Pts',(3.05424592228751,1.47402311063358,58.2304113162848));
#9972=CARTESIAN_POINT('Ctrl Pts',(3.09644810697051,1.37928031354715,58.2243064410737));
#9973=CARTESIAN_POINT('Ctrl Pts',(3.13859525242559,1.284661078083,58.2182095277163));
#9974=CARTESIAN_POINT('Ctrl Pts',(3.17645838472971,1.18798047256889,58.2121126143588));
#9975=CARTESIAN_POINT('Ctrl Pts',(3.20983497811777,1.08966255132115,58.2060157010014));
#9976=CARTESIAN_POINT('Ctrl Pts',(3.24317756125452,0.99144481457008,58.1999250003078));
#9977=CARTESIAN_POINT('Ctrl Pts',(3.27204256008405,0.891593482270475,58.1938342996142));
#9978=CARTESIAN_POINT('Ctrl Pts',(3.29627530702397,0.790553073995696,58.1877435989206));
#9979=CARTESIAN_POINT('Ctrl Pts',(3.32049107022531,0.689583480799553,58.1816571669494));
#9980=CARTESIAN_POINT('Ctrl Pts',(3.34008093841483,0.587426883153269,58.1755707349782));
#9981=CARTESIAN_POINT('Ctrl Pts',(3.35494015657279,0.484542679560132,58.1694843030069));
#9982=CARTESIAN_POINT('Ctrl Pts',(3.3697939802863,0.38169582672904,58.1634000806351));
#9983=CARTESIAN_POINT('Ctrl Pts',(3.37992050636866,0.278122315325744,58.1573158582632));
#9984=CARTESIAN_POINT('Ctrl Pts',(3.38526628596686,0.174290664110741,58.1512316358914));
#9985=CARTESIAN_POINT('Ctrl Pts',(3.39061150535953,0.0704698938276971,58.1451480511094));
#9986=CARTESIAN_POINT('Ctrl Pts',(3.39117695263656,-0.0336085358387061,
58.1390644663274));
#9987=CARTESIAN_POINT('Ctrl Pts',(3.38696121061733,-0.137472980158313,58.1329808815454));
#9988=CARTESIAN_POINT('Ctrl Pts',(3.38274482171547,-0.241353361910595,58.1268963632705));
#9989=CARTESIAN_POINT('Ctrl Pts',(3.3737458032382,-0.345019266201955,58.1208118449956));
#9990=CARTESIAN_POINT('Ctrl Pts',(3.36001477761114,-0.448001960637173,58.1147273267207));
#9991=CARTESIAN_POINT('Ctrl Pts',(3.34626959581532,-0.551090826340421,58.1086365355373));
#9992=CARTESIAN_POINT('Ctrl Pts',(3.32778272108133,-0.653494651343808,58.1025457443539));
#9993=CARTESIAN_POINT('Ctrl Pts',(3.30465631083005,-0.754752760704529,58.0964549531705));
#9994=CARTESIAN_POINT('Ctrl Pts',(3.28151738621992,-0.856065663710415,58.0903608660866));
#9995=CARTESIAN_POINT('Ctrl Pts',(3.25373403933155,-0.956231204422519,58.0842667790027));
#9996=CARTESIAN_POINT('Ctrl Pts',(3.22145840105767,-1.05480369394259,58.0781726919189));
#9997=CARTESIAN_POINT('Ctrl Pts',(3.18913104260161,-1.15353414121003,58.072068839349));
#9998=CARTESIAN_POINT('Ctrl Pts',(3.1522971644833,-1.25066603830035,58.065964986779));
#9999=CARTESIAN_POINT('Ctrl Pts',(3.11115721811499,-1.34577331920016,58.0598611342091));
#10000=CARTESIAN_POINT('Ctrl Pts',(3.08084307172125,-1.41585352811672,58.0553634841949));
#10001=CARTESIAN_POINT('Ctrl Pts',(3.04819193518403,-1.48483489285143,58.0508658341806));
#10002=CARTESIAN_POINT('Ctrl Pts',(3.01329951819504,-1.55255630369579,58.0463681841664));
#10003=CARTESIAN_POINT('Ctrl Pts',(2.96593859253262,-1.64447738516647,58.0402633371434));
#10004=CARTESIAN_POINT('Ctrl Pts',(2.91428875370229,-1.73438266965953,58.0341584901204));
#10005=CARTESIAN_POINT('Ctrl Pts',(2.8585455375631,-1.82184589693478,58.0280536430974));
#10006=CARTESIAN_POINT('Ctrl Pts',(2.80287502211957,-1.90919505405212,58.0219567580589));
#10007=CARTESIAN_POINT('Ctrl Pts',(2.74312197083997,-1.99410812869571,58.0158598730205));
#10008=CARTESIAN_POINT('Ctrl Pts',(2.6795283575144,-2.07618227614441,58.009762987982));
#10009=CARTESIAN_POINT('Ctrl Pts',(2.61599954638329,-2.15817278964649,58.0036723156984));
#10010=CARTESIAN_POINT('Ctrl Pts',(2.54863821592229,-2.2373297927258,57.9975816434148));
#10011=CARTESIAN_POINT('Ctrl Pts',(2.47772981006929,-2.31327906893959,57.9914909711312));
#10012=CARTESIAN_POINT('Ctrl Pts',(2.40687110142809,-2.38917511497254,57.9854045675859));
#10013=CARTESIAN_POINT('Ctrl Pts',(2.33247055190456,-2.46186759358317,57.9793181640407));
#10014=CARTESIAN_POINT('Ctrl Pts',(2.25485354936579,-2.53101571180672,57.9732317604954));
#10015=CARTESIAN_POINT('Ctrl Pts',(2.17726472477847,-2.60013872660894,57.9671475665483));
#10016=CARTESIAN_POINT('Ctrl Pts',(2.09646208666316,-2.66571965459013,57.9610633726011));
#10017=CARTESIAN_POINT('Ctrl Pts',(2.01280693231826,-2.72745546539473,57.954979178654));
#10018=CARTESIAN_POINT('Ctrl Pts',(1.92916054406832,-2.78918480699866,57.9488956222602));
#10019=CARTESIAN_POINT('Ctrl Pts',(1.84266257777046,-2.84706957905873,57.9428120658663));
#10020=CARTESIAN_POINT('Ctrl Pts',(1.75370564057816,-2.90084842566866,57.9367285094725));
#10021=CARTESIAN_POINT('Ctrl Pts',(1.66473505231483,-2.95463552502288,57.930644019514));
#10022=CARTESIAN_POINT('Ctrl Pts',(1.57330510906221,-3.0043152260501,57.9245595295554));
#10023=CARTESIAN_POINT('Ctrl Pts',(1.47983469569119,-3.04967118488675,57.9184750395969));
#10024=CARTESIAN_POINT('Ctrl Pts',(1.38626791299425,-3.09507390636221,57.9123842764426));
#10025=CARTESIAN_POINT('Ctrl Pts',(1.29065684406284,-3.13614379654276,57.9062935132883));
#10026=CARTESIAN_POINT('Ctrl Pts',(1.19344208163425,-3.17271194095596,57.9002027501341));
#10027=CARTESIAN_POINT('Ctrl Pts',(1.09617471138763,-3.20929987423906,57.8941086909602));
#10028=CARTESIAN_POINT('Ctrl Pts',(0.997302325330367,-3.24138107727344,
57.8880146317864));
#10029=CARTESIAN_POINT('Ctrl Pts',(0.897280583532307,-3.26883658461477,
57.8819205726125));
#10030=CARTESIAN_POINT('Ctrl Pts',(0.797098553032237,-3.29633609046637,
57.8758167474736));
#10031=CARTESIAN_POINT('Ctrl Pts',(0.695763904434107,-3.31919499893302,
57.8697129223348));
#10032=CARTESIAN_POINT('Ctrl Pts',(0.593742585796657,-3.33734547272402,
57.8636090971959));
#10033=CARTESIAN_POINT('Ctrl Pts',(0.518562689793627,-3.35072062558655,
57.8591111653392));
#10034=CARTESIAN_POINT('Ctrl Pts',(0.443010110845109,-3.36154004818632,
57.8546132334825));
#10035=CARTESIAN_POINT('Ctrl Pts',(0.367272061257948,-3.36979469634566,
57.8501153016258));
#10036=CARTESIAN_POINT('Ctrl Pts',(0.264476422700178,-3.38099833617048,
57.8440104734724));
#10037=CARTESIAN_POINT('Ctrl Pts',(0.160996214210303,-3.38751270563579,
57.8379056453191));
#10038=CARTESIAN_POINT('Ctrl Pts',(0.0572948345254091,-3.38926575594725,
57.8318008171657));
#10039=CARTESIAN_POINT('Ctrl Pts',(-0.0462712898655252,-3.39101651979603,
57.8257039513975));
#10040=CARTESIAN_POINT('Ctrl Pts',(-0.150057588315461,-3.38801830365918,
57.8196070856293));
#10041=CARTESIAN_POINT('Ctrl Pts',(-0.25359457547218,-3.38025070871838,
57.8135102198611));
#10042=CARTESIAN_POINT('Ctrl Pts',(-0.35702605129341,-3.3724910294929,57.8074195672199));
#10043=CARTESIAN_POINT('Ctrl Pts',(-0.460208297240954,-3.35997166840492,
57.8013289145787));
#10044=CARTESIAN_POINT('Ctrl Pts',(-0.562671726406928,-3.34272427681409,
57.7952382619375));
#10045=CARTESIAN_POINT('Ctrl Pts',(-0.665063334264679,-3.3254889747096,
57.7891518785136));
#10046=CARTESIAN_POINT('Ctrl Pts',(-0.766736707231087,-3.30353230334752,
57.7830654950897));
#10047=CARTESIAN_POINT('Ctrl Pts',(-0.867228101709965,-3.27693766832763,
57.7769791116657));
#10048=CARTESIAN_POINT('Ctrl Pts',(-0.967683009098095,-3.25035268946652,
57.7708949381268));
#10049=CARTESIAN_POINT('Ctrl Pts',(-1.06695637841463,-3.21913320311101,
57.7648107645878));
#10050=CARTESIAN_POINT('Ctrl Pts',(-1.16459615416106,-3.18341339763049,
57.7587265910489));
#10051=CARTESIAN_POINT('Ctrl Pts',(-1.26222569413651,-3.14769733672789,
57.7526430553259));
#10052=CARTESIAN_POINT('Ctrl Pts',(-1.35822157991567,-3.10748204170256,
57.7465595196029));
#10053=CARTESIAN_POINT('Ctrl Pts',(-1.4521492442437,-3.06295080517831,57.7404759838799));
#10054=CARTESIAN_POINT('Ctrl Pts',(-1.54609131880207,-3.01841273674378,
57.7343915148307));
#10055=CARTESIAN_POINT('Ctrl Pts',(-1.63796415544571,-2.96955759429246,
57.7283070457815));
#10056=CARTESIAN_POINT('Ctrl Pts',(-1.72735623495422,-2.91661541860849,
57.7222225767323));
#10057=CARTESIAN_POINT('Ctrl Pts',(-1.81684047570835,-2.86361866071898,
57.7161318347308));
#10058=CARTESIAN_POINT('Ctrl Pts',(-1.90383848355673,-2.80652667310344,
57.7100410927294));
#10059=CARTESIAN_POINT('Ctrl Pts',(-1.98796632453116,-2.74561376654293,
57.7039503507279));
#10060=CARTESIAN_POINT('Ctrl Pts',(-2.07213968919168,-2.68466789847996,
57.6978563128731));
#10061=CARTESIAN_POINT('Ctrl Pts',(-2.15343945909388,-2.6198972591512,57.6917622750183));
#10062=CARTESIAN_POINT('Ctrl Pts',(-2.23151505029761,-2.551616280477,57.6856682371635));
#10063=CARTESIAN_POINT('Ctrl Pts',(-2.30971576035376,-2.48322587915787,
57.6795644334009));
#10064=CARTESIAN_POINT('Ctrl Pts',(-2.38468166214938,-2.4113141971973,57.6734606296383));
#10065=CARTESIAN_POINT('Ctrl Pts',(-2.45609914174325,-2.3362324517111,57.6673568258758));
#10066=CARTESIAN_POINT('Ctrl Pts',(-2.50872952104403,-2.28090172923287,
57.6628586902789));
#10067=CARTESIAN_POINT('Ctrl Pts',(-2.55943361250277,-2.22385016738898,
57.658360554682));
#10068=CARTESIAN_POINT('Ctrl Pts',(-2.60810058429678,-2.16522894971659,
57.6538624190851));
#10069=CARTESIAN_POINT('Ctrl Pts',(-2.67373571648578,-2.08616893777884,
57.6477959696303));
#10070=CARTESIAN_POINT('Ctrl Pts',(-2.73589066789206,-2.00397965075741,
57.6417295201755));
#10071=CARTESIAN_POINT('Ctrl Pts',(-2.79425071179814,-1.91900182962799,
57.6356630707207));
#10072=CARTESIAN_POINT('Ctrl Pts',(-2.85253886398197,-1.83412868974119,
57.6296040943154));
#10073=CARTESIAN_POINT('Ctrl Pts',(-2.90704115285841,-1.74647419305729,
57.6235451179101));
#10074=CARTESIAN_POINT('Ctrl Pts',(-2.95748218850592,-1.65641304244147,
57.6174861415049));
#10075=CARTESIAN_POINT('Ctrl Pts',(-3.00787453655392,-1.56643882226191,
57.6114330134533));
#10076=CARTESIAN_POINT('Ctrl Pts',(-3.05421321077881,-1.47406293961936,
57.6053798854017));
#10077=CARTESIAN_POINT('Ctrl Pts',(-3.09626591985976,-1.37968924617648,
57.5993267573502));
#10078=CARTESIAN_POINT('Ctrl Pts',(-3.13828924777158,-1.28538148925726,
57.5932778584668));
#10079=CARTESIAN_POINT('Ctrl Pts',(-3.17603238760129,-1.18907909040798,
57.5872289595834));
#10080=CARTESIAN_POINT('Ctrl Pts',(-3.20930930246251,-1.09120981650074,
57.5811800607));
#10081=CARTESIAN_POINT('Ctrl Pts',(-3.2425771234788,-0.993367288101756,
57.5751328148469));
#10082=CARTESIAN_POINT('Ctrl Pts',(-3.27138099973524,-0.893959142898774,
57.5690855689938));
#10083=CARTESIAN_POINT('Ctrl Pts',(-3.29558359012354,-0.793431700279532,
57.5630383231407));
#10084=CARTESIAN_POINT('Ctrl Pts',(-3.31978197071577,-0.69292174339323,
57.5569921291449));
#10085=CARTESIAN_POINT('Ctrl Pts',(-3.33938056028478,-0.591293298260086,
57.5509459351491));
#10086=CARTESIAN_POINT('Ctrl Pts',(-3.35429262218253,-0.489005181232123,
57.5448997411534));
#10087=CARTESIAN_POINT('Ctrl Pts',(-3.36921114701185,-0.386672732232781,
57.5388509267193));
#10088=CARTESIAN_POINT('Ctrl Pts',(-3.3794390275335,-0.283680469449326,
57.5328021122852));
#10089=CARTESIAN_POINT('Ctrl Pts',(-3.38494119867162,-0.180494166209239,
57.5267532978511));
#10090=CARTESIAN_POINT('Ctrl Pts',(-3.38819630092862,-0.119448815176464,
57.5231747996506));
#10091=CARTESIAN_POINT('Ctrl Pts',(-3.3897984199058,-0.0583356402219657,
57.5195963014501));
#10092=CARTESIAN_POINT('Ctrl Pts',(-3.38974888547307,0.00274880593522399,
57.5160178032496));
#10093=CARTESIAN_POINT('Ctrl Pts',(-3.38974888547239,0.00274880677971095,
57.5160178032001));
#10094=CARTESIAN_POINT('Ctrl Pts',(-3.38971273417821,0.0473295354305304,
57.5134061390648));
#10095=CARTESIAN_POINT('Ctrl Pts',(-3.38879708094694,0.0918735026493397,
57.5107944749295));
#10096=CARTESIAN_POINT('Ctrl Pts',(-3.38700661857411,0.136349654327205,
57.5081828107941));
#10097=CARTESIAN_POINT('Origin',(0.,0.,0.));
#10098=CARTESIAN_POINT('',(-3.38700661857411,0.13634965432721,56.2578983182294));
#10099=CARTESIAN_POINT('',(-3.3870066172248,0.136349687844955,56.6023307114865));
#10100=CARTESIAN_POINT('',(-3.38700661857411,0.136349654327212,0.));
#10101=CARTESIAN_POINT('',(-3.3897488059115,-0.00284522785732173,56.6089821967874));
#10102=CARTESIAN_POINT('Ctrl Pts',(-3.3870066172248,0.136349687844955,56.6023307114865));
#10103=CARTESIAN_POINT('Ctrl Pts',(-3.38887261232141,0.089997269736533,
56.6048299798626));
#10104=CARTESIAN_POINT('Ctrl Pts',(-3.38978720352182,0.0436035573379319,
56.6073139437703));
#10105=CARTESIAN_POINT('Ctrl Pts',(-3.38974884178032,-0.0028021686143346,
56.6097894001601));
#10106=CARTESIAN_POINT('Ctrl Pts',(-3.3897488059115,-0.00284522785732173,
56.6089821967874));
#10107=CARTESIAN_POINT('Ctrl Pts',(-3.38964186002974,-0.130258459125678,
56.6164508124252));
#10108=CARTESIAN_POINT('Ctrl Pts',(-3.38234738719693,-0.257365485074957,
56.6239194280629));
#10109=CARTESIAN_POINT('Ctrl Pts',(-3.36799108566911,-0.383459397268334,
56.6313880437007));
#10110=CARTESIAN_POINT('Ctrl Pts',(-3.35341785295837,-0.511458654057483,
56.6389695140052));
#10111=CARTESIAN_POINT('Ctrl Pts',(-3.33156780950142,-0.638414026791939,
56.6465509843097));
#10112=CARTESIAN_POINT('Ctrl Pts',(-3.30262132280961,-0.763608185277818,
56.6541324546142));
#10113=CARTESIAN_POINT('Ctrl Pts',(-3.29044357591801,-0.816277194494058,
56.6573219686791));
#10114=CARTESIAN_POINT('Ctrl Pts',(-3.27701043211885,-0.868634749644346,
56.6605114827441));
#10115=CARTESIAN_POINT('Ctrl Pts',(-3.26233783895011,-0.920628528264424,
56.663700996809));
#10116=CARTESIAN_POINT('Ctrl Pts',(-3.23425399410816,-1.02014639771804,
56.6698058357486));
#10117=CARTESIAN_POINT('Ctrl Pts',(-3.20156546326927,-1.11854402577515,
56.6759106746882));
#10118=CARTESIAN_POINT('Ctrl Pts',(-3.16437887173264,-1.21536472658707,
56.6820155136278));
#10119=CARTESIAN_POINT('Ctrl Pts',(-3.12724078050966,-1.31205914977679,
56.6881123903802));
#10120=CARTESIAN_POINT('Ctrl Pts',(-3.08561644387675,-1.40718033914296,
56.6942092671326));
#10121=CARTESIAN_POINT('Ctrl Pts',(-3.03966266118234,-1.50028529577341,
56.700306143885));
#10122=CARTESIAN_POINT('Ctrl Pts',(-2.99375570710999,-1.59329537497332,
56.7063968076921));
#10123=CARTESIAN_POINT('Ctrl Pts',(-2.94352826842955,-1.68429292610074,
56.7124874714992));
#10124=CARTESIAN_POINT('Ctrl Pts',(-2.88918544961746,-1.77285433699972,
56.7185781353063));
#10125=CARTESIAN_POINT('Ctrl Pts',(-2.83488072008213,-1.86135367456201,
56.7246645301229));
#10126=CARTESIAN_POINT('Ctrl Pts',(-2.77646656944074,-1.94741990442321,
56.7307509249395));
#10127=CARTESIAN_POINT('Ctrl Pts',(-2.71419390788892,-2.03065420317657,
56.736837319756));
#10128=CARTESIAN_POINT('Ctrl Pts',(-2.65194385528968,-2.11385828256455,
56.7429215048227));
#10129=CARTESIAN_POINT('Ctrl Pts',(-2.58583833174825,-2.1942321326681,56.7490056898893));
#10130=CARTESIAN_POINT('Ctrl Pts',(-2.5161709647831,-2.27140677521277,56.7550898749559));
#10131=CARTESIAN_POINT('Ctrl Pts',(-2.44651089978538,-2.34857332893838,
56.7611734223277));
#10132=CARTESIAN_POINT('Ctrl Pts',(-2.37329002005761,-2.42254102484428,
56.7672569696994));
#10133=CARTESIAN_POINT('Ctrl Pts',(-2.29684094310858,-2.49297548013616,
56.7733405170712));
#10134=CARTESIAN_POINT('Ctrl Pts',(-2.22038013614038,-2.5634207425894,56.7794249978764));
#10135=CARTESIAN_POINT('Ctrl Pts',(-2.14069046205971,-2.63033139785018,
56.7855094786817));
#10136=CARTESIAN_POINT('Ctrl Pts',(-2.05813926266371,-2.69341193247191,
56.7915939594869));
#10137=CARTESIAN_POINT('Ctrl Pts',(-1.97550295369874,-2.75655750257649,
56.797684713339));
#10138=CARTESIAN_POINT('Ctrl Pts',(-1.88999956796191,-2.81586480642358,
56.803775467191));
#10139=CARTESIAN_POINT('Ctrl Pts',(-1.80202717536295,-2.87108047984612,
56.8098662210431));
#10140=CARTESIAN_POINT('Ctrl Pts',(-1.71400717777831,-2.92632603243035,
56.8159602708183));
#10141=CARTESIAN_POINT('Ctrl Pts',(-1.62351588388813,-2.97747533393892,
56.8220543205936));
#10142=CARTESIAN_POINT('Ctrl Pts',(-1.53097608683248,-3.02432096247193,
56.8281483703689));
#10143=CARTESIAN_POINT('Ctrl Pts',(-1.43828799191684,-3.07124166255989,
56.8342521860456));
#10144=CARTESIAN_POINT('Ctrl Pts',(-1.34354522606689,-3.11384473766319,
56.8403560017223));
#10145=CARTESIAN_POINT('Ctrl Pts',(-1.24719085733065,-3.15197081647195,
56.8464598173991));
#10146=CARTESIAN_POINT('Ctrl Pts',(-1.17618544640889,-3.18006666649056,
56.8509578380493));
#10147=CARTESIAN_POINT('Ctrl Pts',(-1.1043052625122,-3.20573229902079,56.8554558586995));
#10148=CARTESIAN_POINT('Ctrl Pts',(-1.03173196761373,-3.22892152420958,
56.8599538793498));
#10149=CARTESIAN_POINT('Ctrl Pts',(-0.933233438622099,-3.26039459667716,
56.8660587202288));
#10150=CARTESIAN_POINT('Ctrl Pts',(-0.83312918691071,-3.28740899750557,
56.8721635611079));
#10151=CARTESIAN_POINT('Ctrl Pts',(-0.731858946297637,-3.30980173805382,
56.8782684019869));
#10152=CARTESIAN_POINT('Ctrl Pts',(-0.630720786782408,-3.33216527300587,
56.8843652806642));
#10153=CARTESIAN_POINT('Ctrl Pts',(-0.528420075449584,-3.34991904009002,
56.8904621593415));
#10154=CARTESIAN_POINT('Ctrl Pts',(-0.425412807722758,-3.36294945033752,
56.8965590380188));
#10155=CARTESIAN_POINT('Ctrl Pts',(-0.322510508502637,-3.37596658207822,
56.902649703734));
#10156=CARTESIAN_POINT('Ctrl Pts',(-0.218903506322892,-3.38426987525457,
56.9087403694492));
#10157=CARTESIAN_POINT('Ctrl Pts',(-0.115058273113641,-3.38779672593975,
56.9148310351644));
#10158=CARTESIAN_POINT('Ctrl Pts',(-0.0112858263194771,-3.39132110461144,
56.9209174318563));
#10159=CARTESIAN_POINT('Ctrl Pts',(0.0927240936923374,-3.3900756840317,
56.9270038285482));
#10160=CARTESIAN_POINT('Ctrl Pts',(0.196500422972065,-3.38404974051384,
56.93309022524));
#10161=CARTESIAN_POINT('Ctrl Pts',(0.300239074474865,-3.37802598481817,
56.9391744121612));
#10162=CARTESIAN_POINT('Ctrl Pts',(0.403743877766324,-3.36722518059719,
56.9452585990823));
#10163=CARTESIAN_POINT('Ctrl Pts',(0.506545097994257,-3.35168869768629,
56.9513427860034));
#10164=CARTESIAN_POINT('Ctrl Pts',(0.609335543050182,-3.33615384324122,
56.9574263352068));
#10165=CARTESIAN_POINT('Ctrl Pts',(0.71142212929874,-3.31588436108925,56.9635098844102));
#10166=CARTESIAN_POINT('Ctrl Pts',(0.812342469304759,-3.29097322612382,
56.9695934336136));
#10167=CARTESIAN_POINT('Ctrl Pts',(0.913278293676121,-3.26605826900407,
56.9756779162255));
#10168=CARTESIAN_POINT('Ctrl Pts',(1.01304710150471,-3.23650034651049,56.9817623988373));
#10169=CARTESIAN_POINT('Ctrl Pts',(1.11119977064915,-3.20244283824228,56.9878468814492));
#10170=CARTESIAN_POINT('Ctrl Pts',(1.20945363351478,-3.16835021726622,56.9939376370584));
#10171=CARTESIAN_POINT('Ctrl Pts',(1.30608762594269,-3.12974888679338,57.0000283926676));
#10172=CARTESIAN_POINT('Ctrl Pts',(1.4006708312588,-3.08683110729447,57.0061191482769));
#10173=CARTESIAN_POINT('Ctrl Pts',(1.49530521850413,-3.04389010364339,57.0122131997844));
#10174=CARTESIAN_POINT('Ctrl Pts',(1.58788622756578,-2.99662819249913,57.0183072512919));
#10175=CARTESIAN_POINT('Ctrl Pts',(1.67800762340419,-2.94528359895909,57.0244013027994));
#10176=CARTESIAN_POINT('Ctrl Pts',(1.76827344064313,-2.89385672464611,57.0305051201504));
#10177=CARTESIAN_POINT('Ctrl Pts',(1.85607140987124,-2.83833432715919,57.0366089375015));
#10178=CARTESIAN_POINT('Ctrl Pts',(1.94102419005542,-2.77899804895932,57.0427127548526));
#10179=CARTESIAN_POINT('Ctrl Pts',(2.00362727638359,-2.73527217985315,57.0472107571985));
#10180=CARTESIAN_POINT('Ctrl Pts',(2.06468591806405,-2.68947610120408,57.0517087595444));
#10181=CARTESIAN_POINT('Ctrl Pts',(2.12406137954748,-2.64173585326294,57.0562067618903));
#10182=CARTESIAN_POINT('Ctrl Pts',(2.20464782856905,-2.57694112222646,57.0623116076918));
#10183=CARTESIAN_POINT('Ctrl Pts',(2.28240112429059,-2.50834752067921,57.0684164534933));
#10184=CARTESIAN_POINT('Ctrl Pts',(2.35694274785019,-2.43623191544985,57.0745212992948));
#10185=CARTESIAN_POINT('Ctrl Pts',(2.43138715149251,-2.36421036603573,57.0806181829326));
#10186=CARTESIAN_POINT('Ctrl Pts',(2.50262790623314,-2.28867623998084,57.0867150665705));
#10187=CARTESIAN_POINT('Ctrl Pts',(2.57031872641208,-2.20994721818314,57.0928119502083));
#10188=CARTESIAN_POINT('Ctrl Pts',(2.63794056735124,-2.13129842392674,57.0989026209151));
#10189=CARTESIAN_POINT('Ctrl Pts',(2.70201939034689,-2.04946153042162,57.1049932916219));
#10190=CARTESIAN_POINT('Ctrl Pts',(2.76224565651917,-1.96479108190693,57.1110839623287));
#10191=CARTESIAN_POINT('Ctrl Pts',(2.82242970964086,-1.88017997955717,57.1171703640378));
#10192=CARTESIAN_POINT('Ctrl Pts',(2.87876632891486,-1.79273961889025,57.123256765747));
#10193=CARTESIAN_POINT('Ctrl Pts',(2.93098671498355,-1.70285699314122,57.1293431674561));
#10194=CARTESIAN_POINT('Ctrl Pts',(2.98318814167932,-1.61300700059061,57.1354273594083));
#10195=CARTESIAN_POINT('Ctrl Pts',(3.03127609108103,-1.52071687430974,57.1415115513605));
#10196=CARTESIAN_POINT('Ctrl Pts',(3.07502594752727,-1.42640123546429,57.1475957433127));
#10197=CARTESIAN_POINT('Ctrl Pts',(3.11877121836459,-1.33209548224291,57.1536792975548));
#10198=CARTESIAN_POINT('Ctrl Pts',(3.15817912073798,-1.23576502620311,57.1597628517969));
#10199=CARTESIAN_POINT('Ctrl Pts',(3.19307213516039,-1.13784682719699,57.165846406039));
#10200=CARTESIAN_POINT('Ctrl Pts',(3.22797050327646,-1.03991360443757,57.1719308936911));
#10201=CARTESIAN_POINT('Ctrl Pts',(3.25835246372619,-0.940392557154895,
57.1780153813431));
#10202=CARTESIAN_POINT('Ctrl Pts',(3.28408985649337,-0.839737385720894,
57.1840998689952));
#10203=CARTESIAN_POINT('Ctrl Pts',(3.30985378392782,-0.738978441091709,
57.1901906296157));
#10204=CARTESIAN_POINT('Ctrl Pts',(3.33096347518221,-0.63708345197482,57.1962813902363));
#10205=CARTESIAN_POINT('Ctrl Pts',(3.3473415838649,-0.534517898137028,57.2023721508569));
#10206=CARTESIAN_POINT('Ctrl Pts',(3.36372855522335,-0.431896843064933,
57.208466207367));
#10207=CARTESIAN_POINT('Ctrl Pts',(3.37537879595003,-0.328604925011197,
57.214560263877));
#10208=CARTESIAN_POINT('Ctrl Pts',(3.38226691334684,-0.225112392771277,
57.2206543203871));
#10209=CARTESIAN_POINT('Ctrl Pts',(3.38916606901154,-0.12145401285063,57.2267581426756));
#10210=CARTESIAN_POINT('Ctrl Pts',(3.39128784853051,-0.0175948038696428,
57.2328619649642));
#10211=CARTESIAN_POINT('Ctrl Pts',(3.38865901194834,0.0859951349860837,
57.2389657872527));
#10212=CARTESIAN_POINT('Ctrl Pts',(3.38672180256772,0.162331337339262,57.2434637396454));
#10213=CARTESIAN_POINT('Ctrl Pts',(3.38220594902991,0.238521339296662,57.2479616920382));
#10214=CARTESIAN_POINT('Ctrl Pts',(3.37514004745206,0.314379901687965,57.252459644431));
#10215=CARTESIAN_POINT('Ctrl Pts',(3.3655498818297,0.417338620995183,57.2585644716682));
#10216=CARTESIAN_POINT('Ctrl Pts',(3.3512282943769,0.520029839227596,57.2646692989055));
#10217=CARTESIAN_POINT('Ctrl Pts',(3.33219741053062,0.621985112163518,57.2707741261427));
#10218=CARTESIAN_POINT('Ctrl Pts',(3.31319134761721,0.723807410456397,57.2768709911903));
#10219=CARTESIAN_POINT('Ctrl Pts',(3.2894882771873,0.824895255252237,57.2829678562378));
#10220=CARTESIAN_POINT('Ctrl Pts',(3.26116214807592,0.924784572998947,57.2890647212854));
#10221=CARTESIAN_POINT('Ctrl Pts',(3.23286488434433,1.02457209981326,57.2951553734006));
#10222=CARTESIAN_POINT('Ctrl Pts',(3.19995404621545,1.12316311943898,57.3012460255157));
#10223=CARTESIAN_POINT('Ctrl Pts',(3.16255460053077,1.2201038731033,57.3073366776309));
#10224=CARTESIAN_POINT('Ctrl Pts',(3.12518136802837,1.31697668122459,57.3134230608225));
#10225=CARTESIAN_POINT('Ctrl Pts',(3.08332593766757,1.4122011261315,57.3195094440141));
#10226=CARTESIAN_POINT('Ctrl Pts',(3.03716281489217,1.50533952925453,57.3255958272058));
#10227=CARTESIAN_POINT('Ctrl Pts',(2.9910164519659,1.59844411781974,57.3316800006928));
#10228=CARTESIAN_POINT('Ctrl Pts',(2.94056569453136,1.68946378749746,57.3377641741799));
#10229=CARTESIAN_POINT('Ctrl Pts',(2.88603246536578,1.77798247217309,57.3438483476669));
#10230=CARTESIAN_POINT('Ctrl Pts',(2.83150495141147,1.86649187988141,57.3499318835182));
#10231=CARTESIAN_POINT('Ctrl Pts',(2.77289604067865,1.95250046012701,57.3560154193695));
#10232=CARTESIAN_POINT('Ctrl Pts',(2.71047226819966,2.03561910627224,57.3620989552208));
#10233=CARTESIAN_POINT('Ctrl Pts',(2.6480389169188,2.11875050680593,57.3681834245783));
#10234=CARTESIAN_POINT('Ctrl Pts',(2.58178979742299,2.19899075056465,57.3742678939359));
#10235=CARTESIAN_POINT('Ctrl Pts',(2.51203263613444,2.27598266634337,57.3803523632935));
#10236=CARTESIAN_POINT('Ctrl Pts',(2.44220355359522,2.35305396257238,57.3864431058801));
#10237=CARTESIAN_POINT('Ctrl Pts',(2.36885949378041,2.42686992552575,57.3925338484666));
#10238=CARTESIAN_POINT('Ctrl Pts',(2.29234603865026,2.49710926905181,57.3986245910532));
#10239=CARTESIAN_POINT('Ctrl Pts',(2.21579117822909,2.56738662263055,57.4047186296479));
#10240=CARTESIAN_POINT('Ctrl Pts',(2.13606383375847,2.63408322725902,57.4108126682425));
#10241=CARTESIAN_POINT('Ctrl Pts',(2.05354222432641,2.69691849995667,57.4169067068372));
#10242=CARTESIAN_POINT('Ctrl Pts',(1.97088836784478,2.75985447087725,57.4230105115844));
#10243=CARTESIAN_POINT('Ctrl Pts',(1.88543165288359,2.81891650580038,57.4291143163316));
#10244=CARTESIAN_POINT('Ctrl Pts',(1.79757894289601,2.87386760421507,57.4352181210788));
#10245=CARTESIAN_POINT('Ctrl Pts',(1.73283680382821,2.91436324351857,57.4397162563764));
#10246=CARTESIAN_POINT('Ctrl Pts',(1.66679403384351,2.95262724157718,57.4442143916741));
#10247=CARTESIAN_POINT('Ctrl Pts',(1.59962093464496,2.98858125670787,57.4487125269717));
#10248=CARTESIAN_POINT('Ctrl Pts',(1.50845391382177,3.03737788043381,57.4548173754785));
#10249=CARTESIAN_POINT('Ctrl Pts',(1.41489998978665,3.08208049854593,57.4609222239854));
#10250=CARTESIAN_POINT('Ctrl Pts',(1.31936209339541,3.12244915555262,57.4670270724923));
#10251=CARTESIAN_POINT('Ctrl Pts',(1.22394880286001,3.16276516150413,57.473123958715));
#10252=CARTESIAN_POINT('Ctrl Pts',(1.12655707469873,3.19875827943407,57.4792208449377));
#10253=CARTESIAN_POINT('Ctrl Pts',(1.0276147816758,3.23023419011399,57.4853177311605));
#10254=CARTESIAN_POINT('Ctrl Pts',(0.928773316141099,3.26167802515754,57.4914084043301));
#10255=CARTESIAN_POINT('Ctrl Pts',(0.828384832915229,3.28861367809401,57.4974990774997));
#10256=CARTESIAN_POINT('Ctrl Pts',(0.726896744520214,3.31089507313444,57.5035897506694));
#10257=CARTESIAN_POINT('Ctrl Pts',(0.625479793060733,3.33316085028131,57.50967615465));
#10258=CARTESIAN_POINT('Ctrl Pts',(0.522965185272561,3.35077876581744,57.5157625586307));
#10259=CARTESIAN_POINT('Ctrl Pts',(0.419814248494312,3.3636529338297,57.5218489626114));
#10260=CARTESIAN_POINT('Ctrl Pts',(0.316700764153846,3.37652242743966,57.5279331567172));
#10261=CARTESIAN_POINT('Ctrl Pts',(0.212951833497619,3.38465154396669,57.534017350823));
#10262=CARTESIAN_POINT('Ctrl Pts',(0.109036914208985,3.38799586980855,57.5401015449287));
#10263=CARTESIAN_POINT('Ctrl Pts',(0.00513288872784269,3.39133984505165,
57.5461851012046));
#10264=CARTESIAN_POINT('Ctrl Pts',(-0.0989366638004335,3.38990001342401,
57.5522686574806));
#10265=CARTESIAN_POINT('Ctrl Pts',(-0.202700162559035,3.3836840435535,57.5583522137565));
#10266=CARTESIAN_POINT('Ctrl Pts',(-0.306479579844468,3.37746712008095,
57.5644367033206));
#10267=CARTESIAN_POINT('Ctrl Pts',(-0.409952423606365,3.36647262816061,
57.5705211928848));
#10268=CARTESIAN_POINT('Ctrl Pts',(-0.512651027293548,3.35076021026794,
57.5766056824489));
#10269=CARTESIAN_POINT('Ctrl Pts',(-0.615455507529982,3.33503159374621,
57.5826964447835));
#10270=CARTESIAN_POINT('Ctrl Pts',(-0.717483730624558,3.31457540278575,
57.588787207118));
#10271=CARTESIAN_POINT('Ctrl Pts',(-0.818277078790952,3.28950265007118,
57.5948779694525));
#10272=CARTESIAN_POINT('Ctrl Pts',(-0.919124967402067,3.26441633020056,
57.6009720275689));
#10273=CARTESIAN_POINT('Ctrl Pts',(-1.01873624064291,3.23470859464613,57.6070660856853));
#10274=CARTESIAN_POINT('Ctrl Pts',(-1.11666822677616,3.20054013157289,57.6131601438017));
#10275=CARTESIAN_POINT('Ctrl Pts',(-1.21475714666922,3.16631691432188,57.6192639675063));
#10276=CARTESIAN_POINT('Ctrl Pts',(-1.31116100733615,3.1276188497666,57.6253677912109));
#10277=CARTESIAN_POINT('Ctrl Pts',(-1.40545768724504,3.08465455956803,57.6314716149155));
#10278=CARTESIAN_POINT('Ctrl Pts',(-1.47494527903619,3.05299400628238,57.6359695464478));
#10279=CARTESIAN_POINT('Ctrl Pts',(-1.5432890631108,3.01901777520069,57.6404674779801));
#10280=CARTESIAN_POINT('Ctrl Pts',(-1.61032977317947,2.98282468209443,57.6449654095124));
#10281=CARTESIAN_POINT('Ctrl Pts',(-1.70132164212005,2.93370113938277,57.651070285133));
#10282=CARTESIAN_POINT('Ctrl Pts',(-1.79021541915787,2.88032828602235,57.6571751607536));
#10283=CARTESIAN_POINT('Ctrl Pts',(-1.87658868844505,2.82290983860627,57.6632800363743));
#10284=CARTESIAN_POINT('Ctrl Pts',(-1.96284930980489,2.76556627626918,57.6693769500225));
#10285=CARTESIAN_POINT('Ctrl Pts',(-2.04659560599201,2.70418784422879,57.6754738636708));
#10286=CARTESIAN_POINT('Ctrl Pts',(-2.12742946736201,2.63902423708078,57.6815707773191));
#10287=CARTESIAN_POINT('Ctrl Pts',(-2.20818095867115,2.57392703193554,57.6876614781854));
#10288=CARTESIAN_POINT('Ctrl Pts',(-2.28602558597022,2.50505258858575,57.6937521790518));
#10289=CARTESIAN_POINT('Ctrl Pts',(-2.36059470035883,2.43269351196113,57.6998428799182));
#10290=CARTESIAN_POINT('Ctrl Pts',(-2.43511155014103,2.36038515095372,57.7059293118847));
#10291=CARTESIAN_POINT('Ctrl Pts',(-2.50635714674996,2.28459731025723,57.7120157438512));
#10292=CARTESIAN_POINT('Ctrl Pts',(-2.57399702834815,2.2056618871792,57.7181021758177));
#10293=CARTESIAN_POINT('Ctrl Pts',(-2.64161235296234,2.12675512198578,57.7241863980758));
#10294=CARTESIAN_POINT('Ctrl Pts',(-2.70562428671699,2.04470336971534,57.730270620334));
#10295=CARTESIAN_POINT('Ctrl Pts',(-2.7657368153539,1.95987370274108,57.7363548425921));
#10296=CARTESIAN_POINT('Ctrl Pts',(-2.82584304348597,1.87505292692047,57.7424384271517));
#10297=CARTESIAN_POINT('Ctrl Pts',(-2.88205043230161,1.78745516398121,57.7485220117113));
#10298=CARTESIAN_POINT('Ctrl Pts',(-2.93410523756445,1.69747798730849,57.7546055962709));
#10299=CARTESIAN_POINT('Ctrl Pts',(-2.9861680294256,1.60748700573221,57.7606901142149));
#10300=CARTESIAN_POINT('Ctrl Pts',(-3.03407675797104,1.51511625491464,57.766774632159));
#10301=CARTESIAN_POINT('Ctrl Pts',(-3.0776231889659,1.42078871379223,57.772859150103));
#10302=CARTESIAN_POINT('Ctrl Pts',(-3.12121451350251,1.32636392710206,57.7789499407899));
#10303=CARTESIAN_POINT('Ctrl Pts',(-3.16043438014796,1.22997871011556,57.7850407314767));
#10304=CARTESIAN_POINT('Ctrl Pts',(-3.19512239351121,1.13207683174914,57.7911315221635));
#10305=CARTESIAN_POINT('Ctrl Pts',(-3.22982917701831,1.03412197737859,57.7972256086579));
#10306=CARTESIAN_POINT('Ctrl Pts',(-3.25999909849915,0.93464923570353,57.8033196951523));
#10307=CARTESIAN_POINT('Ctrl Pts',(-3.28552199259297,0.834116477890183,
57.8094137816467));
#10308=CARTESIAN_POINT('Ctrl Pts',(-3.3110857853109,0.733422623476364,57.8155176334817));
#10309=CARTESIAN_POINT('Ctrl Pts',(-3.33198758973352,0.63166577852094,57.8216214853166));
#10310=CARTESIAN_POINT('Ctrl Pts',(-3.3481685573649,0.529313115247516,57.8277253371516));
#10311=CARTESIAN_POINT('Ctrl Pts',(-3.36009157867525,0.453894078933964,
57.8322229887854));
#10312=CARTESIAN_POINT('Ctrl Pts',(-3.36945248049841,0.378151716943184,
57.8367206404191));
#10313=CARTESIAN_POINT('Ctrl Pts',(-3.3762458274381,0.302273345180905,57.8412182920529));
#10314=CARTESIAN_POINT('Ctrl Pts',(-3.38118795262616,0.247072217423914,
57.8444903106358));
#10315=CARTESIAN_POINT('Ctrl Pts',(-3.38477645790119,0.191748173648244,
57.8477623292186));
#10316=CARTESIAN_POINT('Ctrl Pts',(-3.38700661857411,0.136349654327218,
57.8510343478015));
#10317=CARTESIAN_POINT('',(-3.3897497300897,-0.00135272198828424,56.2660178032046));
#10318=CARTESIAN_POINT('Ctrl Pts',(-3.38700661857411,0.136349654327205,
57.5081828107941));
#10319=CARTESIAN_POINT('Ctrl Pts',(-3.38197763548836,0.261272589263766,
57.5008472672152));
#10320=CARTESIAN_POINT('Ctrl Pts',(-3.37004365615613,0.385659014010383,
57.4935117236363));
#10321=CARTESIAN_POINT('Ctrl Pts',(-3.351341836764,0.508834900193837,57.4861761800574));
#10322=CARTESIAN_POINT('Ctrl Pts',(-3.33243756055803,0.633344228698431,
57.4787612254464));
#10323=CARTESIAN_POINT('Ctrl Pts',(-3.30661817902444,0.756616668127261,
57.4713462708354));
#10324=CARTESIAN_POINT('Ctrl Pts',(-3.27407407757502,0.877977218981941,
57.4639313162244));
#10325=CARTESIAN_POINT('Ctrl Pts',(-3.26482535208107,0.912466738454293,
57.4618240563311));
#10326=CARTESIAN_POINT('Ctrl Pts',(-3.2550338057071,0.946801975209491,57.4597167964378));
#10327=CARTESIAN_POINT('Ctrl Pts',(-3.24470450886454,0.980967742922328,
57.4576095365445));
#10328=CARTESIAN_POINT('Ctrl Pts',(-3.21478000253734,1.07994773620546,57.451504695821));
#10329=CARTESIAN_POINT('Ctrl Pts',(-3.18027237352543,1.17772228881658,57.4453998550974));
#10330=CARTESIAN_POINT('Ctrl Pts',(-3.14129669794409,1.27383677054227,57.4392950143739));
#10331=CARTESIAN_POINT('Ctrl Pts',(-3.10237185595529,1.36982589602131,57.4331981358212));
#10332=CARTESIAN_POINT('Ctrl Pts',(-3.05899071214014,1.46415886250153,57.4271012572685));
#10333=CARTESIAN_POINT('Ctrl Pts',(-3.01131825421448,1.55639565481745,57.4210043787158));
#10334=CARTESIAN_POINT('Ctrl Pts',(-2.96369437618153,1.64853845463394,57.4149137130943));
#10335=CARTESIAN_POINT('Ctrl Pts',(-2.91178807523235,1.73858895048893,57.4088230474729));
#10336=CARTESIAN_POINT('Ctrl Pts',(-2.85581227638309,1.82612740644229,57.4027323818515));
#10337=CARTESIAN_POINT('Ctrl Pts',(-2.79987571124005,1.91360450627149,57.3966459852069));
#10338=CARTESIAN_POINT('Ctrl Pts',(-2.73987554994441,1.99857270870129,57.3905595885622));
#10339=CARTESIAN_POINT('Ctrl Pts',(-2.67607005565742,2.08063791172652,57.3844731919176));
#10340=CARTESIAN_POINT('Ctrl Pts',(-2.61228772675038,2.16267331995697,57.3783890050151));
#10341=CARTESIAN_POINT('Ctrl Pts',(-2.54470307272899,2.2418074866813,57.3723048181126));
#10342=CARTESIAN_POINT('Ctrl Pts',(-2.47361651326741,2.31767694206738,57.3662206312101));
#10343=CARTESIAN_POINT('Ctrl Pts',(-2.40253740445278,2.39353844550684,57.3601370819968));
#10344=CARTESIAN_POINT('Ctrl Pts',(-2.3279574122225,2.46613560635786,57.3540535327835));
#10345=CARTESIAN_POINT('Ctrl Pts',(-2.25021529798158,2.5351402673678,57.3479699835701));
#10346=CARTESIAN_POINT('Ctrl Pts',(-2.17246125528165,2.60415551619462,57.3418855009198));
#10347=CARTESIAN_POINT('Ctrl Pts',(-2.09154444613331,2.66957688640996,57.3358010182694));
#10348=CARTESIAN_POINT('Ctrl Pts',(-2.0078376294502,2.73111572736562,57.3297165356191));
#10349=CARTESIAN_POINT('Ctrl Pts',(-1.92404451186821,2.79271801425675,57.3236257799274));
#10350=CARTESIAN_POINT('Ctrl Pts',(-1.83745598730845,2.85042952472751,57.3175350242357));
#10351=CARTESIAN_POINT('Ctrl Pts',(-1.74847475588216,2.90400431999383,57.311444268544));
#10352=CARTESIAN_POINT('Ctrl Pts',(-1.65944537357163,2.95760810647238,57.3053502169295));
#10353=CARTESIAN_POINT('Ctrl Pts',(-1.56802108103132,3.0070705154332,57.2992561653149));
#10354=CARTESIAN_POINT('Ctrl Pts',(-1.47462844538664,3.05219200093254,57.2931621137004));
#10355=CARTESIAN_POINT('Ctrl Pts',(-1.38108614551753,3.0973857948327,57.2870582962034));
#10356=CARTESIAN_POINT('Ctrl Pts',(-1.28556959457737,3.13822460130784,57.2809544787063));
#10357=CARTESIAN_POINT('Ctrl Pts',(-1.18852474005114,3.17455729272388,57.2748506612093));
#10358=CARTESIAN_POINT('Ctrl Pts',(-1.11701080816268,3.20133144403706,57.2703526588075));
#10359=CARTESIAN_POINT('Ctrl Pts',(-1.04466732731285,3.22565959362453,57.2658546564056));
#10360=CARTESIAN_POINT('Ctrl Pts',(-0.971676782487739,3.24749892884883,
57.2613566540038));
#10361=CARTESIAN_POINT('Ctrl Pts',(-0.872611577735475,3.27714000387892,
57.2552518149458));
#10362=CARTESIAN_POINT('Ctrl Pts',(-0.772023609033435,3.30229340003505,
57.2491469758878));
#10363=CARTESIAN_POINT('Ctrl Pts',(-0.670355556791719,3.32280431111711,
57.2430421368298));
#10364=CARTESIAN_POINT('Ctrl Pts',(-0.568820104711306,3.34328847092326,
57.2369452599844));
#10365=CARTESIAN_POINT('Ctrl Pts',(-0.466207785054198,3.35914209977304,
57.230848383139));
#10366=CARTESIAN_POINT('Ctrl Pts',(-0.362976620984671,3.37026008419507,
57.2247515062936));
#10367=CARTESIAN_POINT('Ctrl Pts',(-0.259850653755282,3.38136673892959,
57.2186608424187));
#10368=CARTESIAN_POINT('Ctrl Pts',(-0.156107518723505,3.38774730025256,
57.2125701785438));
#10369=CARTESIAN_POINT('Ctrl Pts',(-0.0522147683012444,3.38934782524179,
57.2064795146689));
#10370=CARTESIAN_POINT('Ctrl Pts',(0.0516051622878733,3.39094722840142,
57.2003931198226));
#10371=CARTESIAN_POINT('Ctrl Pts',(0.155574073778021,3.38777325138421,57.1943067249763));
#10372=CARTESIAN_POINT('Ctrl Pts',(0.25922078458868,3.37982390774094,57.1882203301301));
#10373=CARTESIAN_POINT('Ctrl Pts',(0.362829864626517,3.37187745024757,57.1821361450572));
#10374=CARTESIAN_POINT('Ctrl Pts',(0.466116550979529,3.35915910472149,57.1760519599843));
#10375=CARTESIAN_POINT('Ctrl Pts',(0.568611956956358,3.34171894463108,57.1699677749114));
#10376=CARTESIAN_POINT('Ctrl Pts',(0.671096619803711,3.32428061254356,57.1638842275567));
#10377=CARTESIAN_POINT('Ctrl Pts',(0.772789746067758,3.30212152180799,57.1578006802021));
#10378=CARTESIAN_POINT('Ctrl Pts',(0.873230752176608,3.27534320582639,57.1517171328474));
#10379=CARTESIAN_POINT('Ctrl Pts',(0.973687169137708,3.24856078119746,57.1456326520826));
#10380=CARTESIAN_POINT('Ctrl Pts',(1.07289067143477,3.21715783327026,57.1395481713179));
#10381=CARTESIAN_POINT('Ctrl Pts',(1.17039487321885,3.18128604549214,57.1334636905531));
#10382=CARTESIAN_POINT('Ctrl Pts',(1.26799960041298,3.14537727442397,57.1273729367774));
#10383=CARTESIAN_POINT('Ctrl Pts',(1.36390112678428,3.1049906105359,57.1212821830017));
#10384=CARTESIAN_POINT('Ctrl Pts',(1.45767217527427,3.06032627213688,57.115191429226));
#10385=CARTESIAN_POINT('Ctrl Pts',(1.55149396630011,3.01563776442516,57.1090973795472));
#10386=CARTESIAN_POINT('Ctrl Pts',(1.64318260613709,2.96666717254557,57.1030033298684));
#10387=CARTESIAN_POINT('Ctrl Pts',(1.73233634749698,2.91366021382742,57.0969092801895));
#10388=CARTESIAN_POINT('Ctrl Pts',(1.82163295999673,2.86056831010867,57.090805464641));
#10389=CARTESIAN_POINT('Ctrl Pts',(1.90838620250743,2.80342735365667,57.0847016490924));
#10390=CARTESIAN_POINT('Ctrl Pts',(1.99222402192131,2.74252593588095,57.0785978335439));
#10391=CARTESIAN_POINT('Ctrl Pts',(2.05400574576737,2.69764649362973,57.0740998128503));
#10392=CARTESIAN_POINT('Ctrl Pts',(2.11420488743103,2.65072582143083,57.0696017921567));
#10393=CARTESIAN_POINT('Ctrl Pts',(2.17268507085529,2.60189251226536,57.0651037714631));
#10394=CARTESIAN_POINT('Ctrl Pts',(2.25205603393367,2.53561456045648,57.0589989302419));
#10395=CARTESIAN_POINT('Ctrl Pts',(2.32852388960276,2.46559093453856,57.0528940890206));
#10396=CARTESIAN_POINT('Ctrl Pts',(2.4017153185982,2.39210547236336,57.0467892477993));
#10397=CARTESIAN_POINT('Ctrl Pts',(2.47481128838866,2.31871585288304,57.0406923687575));
#10398=CARTESIAN_POINT('Ctrl Pts',(2.54463902820995,2.24187367379535,57.0345954897156));
#10399=CARTESIAN_POINT('Ctrl Pts',(2.61085820328083,2.16190298229619,57.0284986106738));
#10400=CARTESIAN_POINT('Ctrl Pts',(2.67700989861407,2.08201378382797,57.0224079445725));
#10401=CARTESIAN_POINT('Ctrl Pts',(2.73956007066472,1.9990027400187,57.0163172784712));
#10402=CARTESIAN_POINT('Ctrl Pts',(2.79820580868445,1.91323007365675,57.0102266123699));
#10403=CARTESIAN_POINT('Ctrl Pts',(2.85681044147336,1.82751752599,57.0041402152614));
#10404=CARTESIAN_POINT('Ctrl Pts',(2.91151584199323,1.73904755671792,56.998053818153));
#10405=CARTESIAN_POINT('Ctrl Pts',(2.96206043373232,1.64821207659011,56.9919674210445));
#10406=CARTESIAN_POINT('Ctrl Pts',(3.01258667454523,1.55740957556319,56.9858832336883));
#10407=CARTESIAN_POINT('Ctrl Pts',(3.05895490152958,1.46424364355644,56.9797990463321));
#10408=CARTESIAN_POINT('Ctrl Pts',(3.10094822659828,1.36913299516773,56.9737148589758));
#10409=CARTESIAN_POINT('Ctrl Pts',(3.14293715023512,1.27403231557856,56.9676313093194));
#10410=CARTESIAN_POINT('Ctrl Pts',(3.18055191132357,1.17698771577332,56.961547759663));
#10411=CARTESIAN_POINT('Ctrl Pts',(3.2136231241003,1.0784393718461,56.9554642100066));
#10412=CARTESIAN_POINT('Ctrl Pts',(3.24669941113849,0.979875907213559,56.9493797269245));
#10413=CARTESIAN_POINT('Ctrl Pts',(3.27523062887567,0.879808645090815,56.9432952438423));
#10414=CARTESIAN_POINT('Ctrl Pts',(3.29909705297031,0.778693583884322,56.9372107607602));
#10415=CARTESIAN_POINT('Ctrl Pts',(3.32298808303049,0.677474274395736,56.931120004657));
#10416=CARTESIAN_POINT('Ctrl Pts',(3.34220461692821,0.575205425093327,56.9250292485538));
#10417=CARTESIAN_POINT('Ctrl Pts',(3.35667795364865,0.472353869454985,56.9189384924505));
#10418=CARTESIAN_POINT('Ctrl Pts',(3.3711591223764,0.369446657394704,56.9128444404352));
#10419=CARTESIAN_POINT('Ctrl Pts',(3.38089194118954,0.265956536251279,56.9067503884198));
#10420=CARTESIAN_POINT('Ctrl Pts',(3.38585974227279,0.162354144254032,56.9006563364044));
#10421=CARTESIAN_POINT('Ctrl Pts',(3.39083550437345,0.0585857270007194,
56.8945525185282));
#10422=CARTESIAN_POINT('Ctrl Pts',(3.39103099444868,-0.0452948930979188,
56.888448700652));
#10423=CARTESIAN_POINT('Ctrl Pts',(3.38648168568396,-0.148818194543216,
56.8823448827758));
#10424=CARTESIAN_POINT('Ctrl Pts',(3.38312922957903,-0.225106119123088,
56.8778468848247));
#10425=CARTESIAN_POINT('Ctrl Pts',(3.37720123175873,-0.301200046176631,
56.8733488868736));
#10426=CARTESIAN_POINT('Ctrl Pts',(3.36872971970812,-0.376915292944285,
56.8688508889225));
#10427=CARTESIAN_POINT('Ctrl Pts',(3.35723188668417,-0.479678679161534,
56.862746048479));
#10428=CARTESIAN_POINT('Ctrl Pts',(3.34100838685991,-0.58208686381503,56.8566412080356));
#10429=CARTESIAN_POINT('Ctrl Pts',(3.32009002990701,-0.683671891927732,
56.8505363675921));
#10430=CARTESIAN_POINT('Ctrl Pts',(3.2991989555468,-0.785124428614343,56.8444394893359));
#10431=CARTESIAN_POINT('Ctrl Pts',(3.2736252831753,-0.885755528207205,56.8383426110798));
#10432=CARTESIAN_POINT('Ctrl Pts',(3.24345155588875,-0.98510256679336,56.8322457328236));
#10433=CARTESIAN_POINT('Ctrl Pts',(3.21330857676029,-1.08434836702668,56.8261550675147));
#10434=CARTESIAN_POINT('Ctrl Pts',(3.17857498795036,-1.18231230166627,56.8200644022057));
#10435=CARTESIAN_POINT('Ctrl Pts',(3.139384150489,-1.27854300598708,56.8139737368968));
#10436=CARTESIAN_POINT('Ctrl Pts',(3.10022078222212,-1.37470626138096,56.8078873405875));
#10437=CARTESIAN_POINT('Ctrl Pts',(3.05660653873389,-1.46913830779342,56.8018009442782));
#10438=CARTESIAN_POINT('Ctrl Pts',(3.00872401291701,-1.56140477666638,56.7957145479689));
#10439=CARTESIAN_POINT('Ctrl Pts',(2.96085887155836,-1.65363774683502,56.7896303614157));
#10440=CARTESIAN_POINT('Ctrl Pts',(2.90872872446253,-1.7437063233682,56.7835461748625));
#10441=CARTESIAN_POINT('Ctrl Pts',(2.8525631728965,-1.83119862580078,56.7774619883092));
#10442=CARTESIAN_POINT('Ctrl Pts',(2.79640350821829,-1.91868175789041,56.7713784394587));
#10443=CARTESIAN_POINT('Ctrl Pts',(2.73620951100475,-2.0035887933858,56.7652948906082));
#10444=CARTESIAN_POINT('Ctrl Pts',(2.67225488715546,-2.08553563397362,56.7592113417577));
#10445=CARTESIAN_POINT('Ctrl Pts',(2.60829045048589,-2.16749504800135,56.7531268594833));
#10446=CARTESIAN_POINT('Ctrl Pts',(2.54056450364021,-2.24649302792661,56.7470423772089));
#10447=CARTESIAN_POINT('Ctrl Pts',(2.46939134461489,-2.32217816922843,56.7409578949345));
#10448=CARTESIAN_POINT('Ctrl Pts',(2.39814480697646,-2.39794134093913,56.734867139637));
#10449=CARTESIAN_POINT('Ctrl Pts',(2.3234442529993,-2.47038454153069,56.7287763843395));
#10450=CARTESIAN_POINT('Ctrl Pts',(2.24564116425911,-2.53919294735256,56.722685629042));
#10451=CARTESIAN_POINT('Ctrl Pts',(2.16779597365636,-2.60803858771219,56.7165915778324));
#10452=CARTESIAN_POINT('Ctrl Pts',(2.08684523675812,-2.67324524731672,56.7104975266229));
#10453=CARTESIAN_POINT('Ctrl Pts',(2.0031723119033,-2.73453940387115,56.7044034754133));
#10454=CARTESIAN_POINT('Ctrl Pts',(1.91936529910049,-2.79593178583949,56.6982996583347));
#10455=CARTESIAN_POINT('Ctrl Pts',(1.83282774027427,-2.85339890383266,56.6921958412561));
#10456=CARTESIAN_POINT('Ctrl Pts',(1.74397082505208,-2.90671134168276,56.6860920241775));
#10457=CARTESIAN_POINT('Ctrl Pts',(1.67849066294818,-2.94599817787158,56.6815940182456));
#10458=CARTESIAN_POINT('Ctrl Pts',(1.61175155109226,-2.98302976614351,56.6770960123138));
#10459=CARTESIAN_POINT('Ctrl Pts',(1.54392519925981,-3.01773094254451,56.6725980063819));
#10460=CARTESIAN_POINT('Ctrl Pts',(1.45186906274478,-3.06482851075654,56.6664931660518));
#10461=CARTESIAN_POINT('Ctrl Pts',(1.35750235757375,-3.10778852350133,56.6603883257217));
#10462=CARTESIAN_POINT('Ctrl Pts',(1.26123239426683,-3.14637853891612,56.6542834853916));
#10463=CARTESIAN_POINT('Ctrl Pts',(1.16508799032235,-3.18491822359883,56.6481866072527));
#10464=CARTESIAN_POINT('Ctrl Pts',(1.0670456566205,-3.21909908462528,56.6420897291139));
#10465=CARTESIAN_POINT('Ctrl Pts',(0.967536795021359,-3.24873477107316,
56.635992850975));
#10466=CARTESIAN_POINT('Ctrl Pts',(0.868129336742945,-3.27834025762759,
56.6299021857872));
#10467=CARTESIAN_POINT('Ctrl Pts',(0.767258729715019,-3.30340965881391,
56.6238115205995));
#10468=CARTESIAN_POINT('Ctrl Pts',(0.665375017554338,-3.32380522120574,
56.6177208554117));
#10469=CARTESIAN_POINT('Ctrl Pts',(0.563562716651571,-3.34418648815491,
56.6116344592288));
#10470=CARTESIAN_POINT('Ctrl Pts',(0.460739140447227,-3.35990034734694,
56.6055480630459));
#10471=CARTESIAN_POINT('Ctrl Pts',(0.357367314247439,-3.37085948464299,
56.599461666863));
#10472=CARTESIAN_POINT('Ctrl Pts',(0.254033018770817,-3.38181464305655,
56.5933774804393));
#10473=CARTESIAN_POINT('Ctrl Pts',(0.150151293299678,-3.38801846562094,
56.5872932940157));
#10474=CARTESIAN_POINT('Ctrl Pts',(0.0461923375375434,-3.38943525243555,
56.581209107592));
#10475=CARTESIAN_POINT('Ctrl Pts',(-0.0577557219079818,-3.39085189075157,
56.5751255588741));
#10476=CARTESIAN_POINT('Ctrl Pts',(-0.161780568384527,-3.38748248532737,
56.5690420101562));
#10477=CARTESIAN_POINT('Ctrl Pts',(-0.265410845296043,-3.37934344891123,
56.5629584614383));
#10478=CARTESIAN_POINT('Ctrl Pts',(-0.369057022577222,-3.37120316369317,
56.5568739792994));
#10479=CARTESIAN_POINT('Ctrl Pts',(-0.472308084088825,-3.35829182695691,
56.5507894971605));
#10480=CARTESIAN_POINT('Ctrl Pts',(-0.574697550708619,-3.3406777437684,
56.5447050150216));
#10481=CARTESIAN_POINT('Ctrl Pts',(-0.677192579494404,-3.3230455006965,
56.5386142598633));
#10482=CARTESIAN_POINT('Ctrl Pts',(-0.778823817675819,-3.30070090139576,
56.532523504705));
#10483=CARTESIAN_POINT('Ctrl Pts',(-0.879134786017541,-3.27376344449532,
56.5264327495467));
#10484=CARTESIAN_POINT('Ctrl Pts',(-0.979500035955152,-3.24681141084248,
56.5203386984785));
#10485=CARTESIAN_POINT('Ctrl Pts',(-1.07854318584358,-3.21526169858401,
56.5142446474103));
#10486=CARTESIAN_POINT('Ctrl Pts',(-1.175824621046,-3.17928317754837,56.5081505963421));
#10487=CARTESIAN_POINT('Ctrl Pts',(-1.273261952141,-3.14324700004786,56.5020467794072));
#10488=CARTESIAN_POINT('Ctrl Pts',(-1.3689315354293,-3.10276800306601,56.4959429624723));
#10489=CARTESIAN_POINT('Ctrl Pts',(-1.46241519191532,-3.05806260056188,
56.4898391455374));
#10490=CARTESIAN_POINT('Ctrl Pts',(-1.53130489936172,-3.02511842384106,
56.4853411383053));
#10491=CARTESIAN_POINT('Ctrl Pts',(-1.59900801369582,-2.9898801018946,56.4808431310733));
#10492=CARTESIAN_POINT('Ctrl Pts',(-1.66536712062625,-2.95244939262928,
56.4763451238412));
#10493=CARTESIAN_POINT('Ctrl Pts',(-1.75543184228785,-2.90164722594083,
56.470240283253));
#10494=CARTESIAN_POINT('Ctrl Pts',(-1.84332007246911,-2.84663542959565,
56.4641354426648));
#10495=CARTESIAN_POINT('Ctrl Pts',(-1.92861324830859,-2.78762551303947,
56.4580306020766));
#10496=CARTESIAN_POINT('Ctrl Pts',(-2.01379518123969,-2.72869255967145,
56.4519337236755));
#10497=CARTESIAN_POINT('Ctrl Pts',(-2.09638844032221,-2.66577209419138,
56.4458368452744));
#10498=CARTESIAN_POINT('Ctrl Pts',(-2.17599961693015,-2.59912114562208,
56.4397399668732));
#10499=CARTESIAN_POINT('Ctrl Pts',(-2.25552966676952,-2.53253811686392,
56.4336493014194));
#10500=CARTESIAN_POINT('Ctrl Pts',(-2.33208335126618,-2.46223243742888,
56.4275586359655));
#10501=CARTESIAN_POINT('Ctrl Pts',(-2.40529751288698,-2.38850349319395,
56.4214679705117));
#10502=CARTESIAN_POINT('Ctrl Pts',(-2.47846035806661,-2.3148262262158,56.4153815740581));
#10503=CARTESIAN_POINT('Ctrl Pts',(-2.54828803501001,-2.23773076824747,
56.4092951776045));
#10504=CARTESIAN_POINT('Ctrl Pts',(-2.61445229577363,-2.15755515702936,
56.4032087811509));
#10505=CARTESIAN_POINT('Ctrl Pts',(-2.68059253462078,-2.07740865475638,
56.3971245944538));
#10506=CARTESIAN_POINT('Ctrl Pts',(-2.74307172920056,-1.99418455104031,
56.3910404077568));
#10507=CARTESIAN_POINT('Ctrl Pts',(-2.80160072466742,-1.90825533984396,
56.3849562210597));
#10508=CARTESIAN_POINT('Ctrl Pts',(-2.86012358552046,-1.8223351351669,56.378872672066));
#10509=CARTESIAN_POINT('Ctrl Pts',(-2.91469683016211,-1.73371073995053,
56.3727891230723));
#10510=CARTESIAN_POINT('Ctrl Pts',(-2.9650741320207,-1.6427843602012,56.3667055740786));
#10511=CARTESIAN_POINT('Ctrl Pts',(-3.01545916346851,-1.55184402925683,
56.3606210916618));
#10512=CARTESIAN_POINT('Ctrl Pts',(-3.06164676598381,-1.45860138574944,
56.354536609245));
#10513=CARTESIAN_POINT('Ctrl Pts',(-3.10343658625327,-1.36348319300411,
56.3484521268283));
#10514=CARTESIAN_POINT('Ctrl Pts',(-3.14526949127501,-1.26826693465939,
56.3423613713906));
#10515=CARTESIAN_POINT('Ctrl Pts',(-3.18269538743489,-1.17117165741252,
56.3362706159529));
#10516=CARTESIAN_POINT('Ctrl Pts',(-3.21556213755194,-1.07264402391585,
56.3301798605151));
#10517=CARTESIAN_POINT('Ctrl Pts',(-3.24844667296481,-0.974063073827136,
56.3240858091663));
#10518=CARTESIAN_POINT('Ctrl Pts',(-3.27676703159179,-0.874048634611226,
56.3179917578175));
#10519=CARTESIAN_POINT('Ctrl Pts',(-3.30042155918176,-0.773060537207965,
56.3118977064687));
#10520=CARTESIAN_POINT('Ctrl Pts',(-3.32411399372917,-0.671910603915307,
56.3057938892539));
#10521=CARTESIAN_POINT('Ctrl Pts',(-3.34312558302879,-0.569784315802146,
56.2996900720391));
#10522=CARTESIAN_POINT('Ctrl Pts',(-3.35740615336754,-0.467149851578451,
56.2935862548243));
#10523=CARTESIAN_POINT('Ctrl Pts',(-3.36792974336041,-0.391516806468435,
56.2890882503164));
#10524=CARTESIAN_POINT('Ctrl Pts',(-3.37588525623752,-0.315607954960892,
56.2845902458085));
#10525=CARTESIAN_POINT('Ctrl Pts',(-3.3812707318465,-0.239610726926493,
56.2800922413006));
#10526=CARTESIAN_POINT('Ctrl Pts',(-3.38688785552139,-0.160344593382771,
56.2754007619502));
#10527=CARTESIAN_POINT('Ctrl Pts',(-3.38971799424802,-0.0808786711404675,
56.2707092825999));
#10528=CARTESIAN_POINT('Ctrl Pts',(-3.3897497300894,-0.00135272275167798,
56.2660178032496));
#10529=CARTESIAN_POINT('Ctrl Pts',(-3.3897497300897,-0.00135272198827972,
56.2660178032046));
#10530=CARTESIAN_POINT('Ctrl Pts',(-3.38976803835472,0.0445254680142906,
56.2633113082128));
#10531=CARTESIAN_POINT('Ctrl Pts',(-3.38885478857705,0.0904400107489448,
56.2606048132211));
#10532=CARTESIAN_POINT('Ctrl Pts',(-3.38700661857411,0.136349654327209,
56.2578983182294));
#10533=CARTESIAN_POINT('Origin',(0.,0.,0.));
#10534=CARTESIAN_POINT('',(-3.38700661857411,0.136349654327209,55.0079919592607));
#10535=CARTESIAN_POINT('',(-3.38700661431188,0.136349760203538,55.352502545304));
#10536=CARTESIAN_POINT('',(-3.38700661857411,0.136349654327212,0.));
#10537=CARTESIAN_POINT('Ctrl Pts',(-3.38700661431188,0.136349760203538,
55.352502545304));
#10538=CARTESIAN_POINT('Ctrl Pts',(-3.38880281242614,0.0917311639953066,
55.3553323773583));
#10539=CARTESIAN_POINT('Ctrl Pts',(-3.38971764573037,0.04706943732554,55.3581464239571));
#10540=CARTESIAN_POINT('Ctrl Pts',(-3.38981775511018,-0.0948718230840635,
55.3670241442622));
#10541=CARTESIAN_POINT('Ctrl Pts',(-3.38570021853797,-0.192098489435276,
55.3730055851047));
#10542=CARTESIAN_POINT('Ctrl Pts',(-3.37361926428369,-0.333272692528037,
55.3815389378329));
#10543=CARTESIAN_POINT('Ctrl Pts',(-3.36896296292172,-0.377447295195299,
55.3841876439945));
#10544=CARTESIAN_POINT('Ctrl Pts',(-3.35913793120111,-0.455844430543228,
55.3888523496557));
#10545=CARTESIAN_POINT('Ctrl Pts',(-3.35431085657523,-0.490102635728252,
55.3908784690254));
#10546=CARTESIAN_POINT('Ctrl Pts',(-3.34297290915396,-0.562526140321877,
55.3951379255789));
#10547=CARTESIAN_POINT('Ctrl Pts',(-3.3363309162693,-0.600666066013674,
55.3973669167801));
#10548=CARTESIAN_POINT('Ctrl Pts',(-3.31620064344492,-0.705591685659972,
55.4034655097463));
#10549=CARTESIAN_POINT('Ctrl Pts',(-3.3013497900379,-0.772098925274634,
55.4072930631311));
#10550=CARTESIAN_POINT('Ctrl Pts',(-3.24996096974156,-0.973487097817526,
55.4188137828708));
#10551=CARTESIAN_POINT('Ctrl Pts',(-3.20708058215176,-1.10659915118776,
55.4263266836567));
#10552=CARTESIAN_POINT('Ctrl Pts',(-3.06884593201819,-1.45938166653565,
55.4465108615667));
#10553=CARTESIAN_POINT('Ctrl Pts',(-2.95827328279954,-1.67218528840312,
55.4589658256642));
#10554=CARTESIAN_POINT('Ctrl Pts',(-2.80533079094595,-1.90314465635302,
55.474592369687));
#10555=CARTESIAN_POINT('Ctrl Pts',(-2.78388574653216,-1.93437853868915,
55.4767553418103));
#10556=CARTESIAN_POINT('Ctrl Pts',(-2.74942070224973,-1.98281513807268,
55.4801993479608));
#10557=CARTESIAN_POINT('Ctrl Pts',(-2.73675170902076,-2.00026500711701,
55.4814588430929));
#10558=CARTESIAN_POINT('Ctrl Pts',(-2.71183028863784,-2.03391099798975,
55.4839264865651));
#10559=CARTESIAN_POINT('Ctrl Pts',(-2.69959728825885,-2.0501199648902,55.4851334390427));
#10560=CARTESIAN_POINT('Ctrl Pts',(-2.66786323386809,-2.09139170281684,
55.4882515406727));
#10561=CARTESIAN_POINT('Ctrl Pts',(-2.64815451449506,-2.11629180375309,
55.4901758566423));
#10562=CARTESIAN_POINT('Ctrl Pts',(-2.5504389884697,-2.23624364747822,55.4996433378818));
#10563=CARTESIAN_POINT('Ctrl Pts',(-2.46765475187571,-2.32727299493945,
55.5074396122191));
#10564=CARTESIAN_POINT('Ctrl Pts',(-2.18047788780646,-2.61046643725383,
55.533283838457));
#10565=CARTESIAN_POINT('Ctrl Pts',(-1.95714454417599,-2.78184294702616,
55.551470872835));
#10566=CARTESIAN_POINT('Ctrl Pts',(-1.66255431199399,-2.95466559960069,
55.5723520284109));
#10567=CARTESIAN_POINT('Ctrl Pts',(-1.6090442926027,-2.98414356620845,55.5760391877437));
#10568=CARTESIAN_POINT('Ctrl Pts',(-1.52157296811918,-3.02929297571206,
55.5819012363272));
#10569=CARTESIAN_POINT('Ctrl Pts',(-1.48809988070516,-3.04587575920181,
55.5841067719575));
#10570=CARTESIAN_POINT('Ctrl Pts',(-1.42272979940289,-3.0769255844328,55.5883435730693));
#10571=CARTESIAN_POINT('Ctrl Pts',(-1.39086938580202,-3.09145817034851,
55.5903768468966));
#10572=CARTESIAN_POINT('Ctrl Pts',(-1.31453504042211,-3.12485775517422,
55.59517660708));
#10573=CARTESIAN_POINT('Ctrl Pts',(-1.26987119058267,-3.14327311089009,
55.5979279373855));
#10574=CARTESIAN_POINT('Ctrl Pts',(-1.09803808267832,-3.20986089594365,
55.6083151015919));
#10575=CARTESIAN_POINT('Ctrl Pts',(-0.968400955818843,-3.25132268966853,
55.6157378193699));
#10576=CARTESIAN_POINT('Ctrl Pts',(-0.697786346824847,-3.32024431414935,
55.6307362414596));
#10577=CARTESIAN_POINT('Ctrl Pts',(-0.556858385623788,-3.34676516665912,
55.6382836507556));
#10578=CARTESIAN_POINT('Ctrl Pts',(-0.278703994817397,-3.38104985318099,
55.6532280102531));
#10579=CARTESIAN_POINT('Ctrl Pts',(-0.141853269206001,-3.38954941346553,
55.6606053537901));
#10580=CARTESIAN_POINT('Ctrl Pts',(0.0343109744158353,-3.3898028743182,
55.6705286109024));
#10581=CARTESIAN_POINT('Ctrl Pts',(0.0734953391494766,-3.38917968422495,
55.672763226355));
#10582=CARTESIAN_POINT('Ctrl Pts',(0.134476779517066,-3.38715184635258,
55.6762954324407));
#10583=CARTESIAN_POINT('Ctrl Pts',(0.156287090053255,-3.38621557553222,
55.6775696230163));
#10584=CARTESIAN_POINT('Ctrl Pts',(0.198211625919492,-3.3840099538928,55.6800424057753));
#10585=CARTESIAN_POINT('Ctrl Pts',(0.218326150781844,-3.38277176774475,
55.6812394022601));
#10586=CARTESIAN_POINT('Ctrl Pts',(0.269280404435321,-3.37917885782386,
55.6842967597014));
#10587=CARTESIAN_POINT('Ctrl Pts',(0.300100799070864,-3.37658126702778,
55.6861693245666));
#10588=CARTESIAN_POINT('Ctrl Pts',(0.440105225867371,-3.36284958651597,
55.6947687799499));
#10589=CARTESIAN_POINT('Ctrl Pts',(0.548737075808639,-3.34683934463749,
55.7016976787149));
#10590=CARTESIAN_POINT('Ctrl Pts',(0.808585014055161,-3.29555164432306,
55.7186220205351));
#10591=CARTESIAN_POINT('Ctrl Pts',(0.958537651659366,-3.25510018163623,
55.7286744849725));
#10592=CARTESIAN_POINT('Ctrl Pts',(1.25736348858366,-3.15203930367955,55.7488581084028));
#10593=CARTESIAN_POINT('Ctrl Pts',(1.40561565967696,-3.08878139120974,55.7589506057311));
#10594=CARTESIAN_POINT('Ctrl Pts',(1.594071059493,-2.9919775640794,55.7717910396497));
#10595=CARTESIAN_POINT('Ctrl Pts',(1.63878865496302,-2.96772041259873,55.7748401040756));
#10596=CARTESIAN_POINT('Ctrl Pts',(1.7133985679064,-2.92504721228157,55.7799336968657));
#10597=CARTESIAN_POINT('Ctrl Pts',(1.74358044913255,-2.90715723699086,55.7819960444295));
#10598=CARTESIAN_POINT('Ctrl Pts',(1.8045874397261,-2.86970409864575,55.7861705128455));
#10599=CARTESIAN_POINT('Ctrl Pts',(1.83538517950259,-2.85010505656818,55.7882809955759));
#10600=CARTESIAN_POINT('Ctrl Pts',(1.91317657744602,-2.79881624116049,55.7936239139676));
#10601=CARTESIAN_POINT('Ctrl Pts',(1.9597038582622,-2.76643783023996,55.7968309384294));
#10602=CARTESIAN_POINT('Ctrl Pts',(2.13445581969581,-2.63820532358989,55.8089519765371));
#10603=CARTESIAN_POINT('Ctrl Pts',(2.25664964967774,-2.53447584893079,55.8175768828203));
#10604=CARTESIAN_POINT('Ctrl Pts',(2.54308768766548,-2.25411903199912,55.8389312186935));
#10605=CARTESIAN_POINT('Ctrl Pts',(2.69666924870136,-2.06792076541547,55.8514610143064));
#10606=CARTESIAN_POINT('Ctrl Pts',(2.84994352990845,-1.83565852459641,55.8671639727908));
#10607=CARTESIAN_POINT('Ctrl Pts',(2.87013951976179,-1.80391774631296,55.8693122946878));
#10608=CARTESIAN_POINT('Ctrl Pts',(2.90104523711558,-1.75351197349775,55.8727382585398));
#10609=CARTESIAN_POINT('Ctrl Pts',(2.91211316116165,-1.73506904523594,55.8739947342902));
#10610=CARTESIAN_POINT('Ctrl Pts',(2.93330578501534,-1.69898088908525,55.8764615298813));
#10611=CARTESIAN_POINT('Ctrl Pts',(2.94344847611743,-1.68134763994268,55.877670738164));
#10612=CARTESIAN_POINT('Ctrl Pts',(2.96910635766999,-1.63579723103008,55.8808023440801));
#10613=CARTESIAN_POINT('Ctrl Pts',(2.98438658993576,-1.6077504985349,55.882738123091));
#10614=CARTESIAN_POINT('Ctrl Pts',(3.05816346487137,-1.46765708426681,55.8924291476583));
#10615=CARTESIAN_POINT('Ctrl Pts',(3.11075323487543,-1.35262336918258,55.9004516674915));
#10616=CARTESIAN_POINT('Ctrl Pts',(3.26245885446327,-0.964826534104013,
55.9271509510384));
#10617=CARTESIAN_POINT('Ctrl Pts',(3.33304080208288,-0.682218090902137,
55.9459394379256));
#10618=CARTESIAN_POINT('Ctrl Pts',(3.37308522068366,-0.340079481245563,
55.9668837423022));
#10619=CARTESIAN_POINT('Ctrl Pts',(3.37810371588516,-0.28596109934416,55.9701496393307));
#10620=CARTESIAN_POINT('Ctrl Pts',(3.38428441609053,-0.195766326280985,
55.9755172405826));
#10621=CARTESIAN_POINT('Ctrl Pts',(3.38617557696697,-0.159751601037691,
55.9776406480183));
#10622=CARTESIAN_POINT('Ctrl Pts',(3.38880006037581,-0.0878880758427056,
55.9818401505056));
#10623=CARTESIAN_POINT('Ctrl Pts',(3.38954004312717,-0.0520442220928807,
55.9839161807035));
#10624=CARTESIAN_POINT('Ctrl Pts',(3.38996541981011,0.0369932491460334,
55.9890306157176));
#10625=CARTESIAN_POINT('Ctrl Pts',(3.38896766102692,0.0901813160466013,
55.99204805566));
#10626=CARTESIAN_POINT('Ctrl Pts',(3.38407446071835,0.205805093592326,55.9985396919981));
#10627=CARTESIAN_POINT('Ctrl Pts',(3.37970182287387,0.268201167569212,56.0019996490059));
#10628=CARTESIAN_POINT('Ctrl Pts',(3.36075269775636,0.46165923984409,56.012637151543));
#10629=CARTESIAN_POINT('Ctrl Pts',(3.34025515711655,0.592018612691681,56.0196716343036));
#10630=CARTESIAN_POINT('Ctrl Pts',(3.26610644093321,0.932719486350201,56.0381979578883));
#10631=CARTESIAN_POINT('Ctrl Pts',(3.19978173144393,1.13964588842961,56.0495836336144));
#10632=CARTESIAN_POINT('Ctrl Pts',(3.10001099804948,1.37172204303961,56.0638682740228));
#10633=CARTESIAN_POINT('Ctrl Pts',(3.08533521774873,1.40442014063747,56.065918459289));
#10634=CARTESIAN_POINT('Ctrl Pts',(3.06118341709256,1.45602474071922,56.0692235435943));
#10635=CARTESIAN_POINT('Ctrl Pts',(3.05204377953239,1.47508666695356,56.0704597045032));
#10636=CARTESIAN_POINT('Ctrl Pts',(3.03364057957295,1.51256565650118,56.072922975289));
#10637=CARTESIAN_POINT('Ctrl Pts',(3.02438616826005,1.53098604634607,56.074149563588));
#10638=CARTESIAN_POINT('Ctrl Pts',(2.99973962677736,1.5789480177251,56.0773829200129));
#10639=CARTESIAN_POINT('Ctrl Pts',(2.98407929569765,1.60834860898335,56.0794046962201));
#10640=CARTESIAN_POINT('Ctrl Pts',(2.88570846707277,1.78664559434733,56.0918888753432));
#10641=CARTESIAN_POINT('Ctrl Pts',(2.79231127632899,1.9293533093108,56.1028317612555));
#10642=CARTESIAN_POINT('Ctrl Pts',(2.54428152318409,2.25237380889502,56.1290482364958));
#10643=CARTESIAN_POINT('Ctrl Pts',(2.3806355117399,2.42469821129782,56.1442309296979));
#10644=CARTESIAN_POINT('Ctrl Pts',(2.15665389132087,2.61582603308636,56.1621803429106));
#10645=CARTESIAN_POINT('Ctrl Pts',(2.11203506676749,2.65198233670601,56.1656384560089));
#10646=CARTESIAN_POINT('Ctrl Pts',(2.03746995525649,2.70932907650006,56.1712315788607));
#10647=CARTESIAN_POINT('Ctrl Pts',(2.00806163105059,2.73119689977044,56.1733922464689));
#10648=CARTESIAN_POINT('Ctrl Pts',(1.9495621717022,2.7732409146765,56.1776044600269));
#10649=CARTESIAN_POINT('Ctrl Pts',(1.92049821387228,2.79344672040605,56.1796569491292));
#10650=CARTESIAN_POINT('Ctrl Pts',(1.84910307177839,2.84144089939737,56.1846054641413));
#10651=CARTESIAN_POINT('Ctrl Pts',(1.80645484846148,2.86874359420123,56.1874836230846));
#10652=CARTESIAN_POINT('Ctrl Pts',(1.62063315210809,2.98191572269229,56.199717988057));
#10653=CARTESIAN_POINT('Ctrl Pts',(1.47183097478437,3.05810310006835,56.2087373051968));
#10654=CARTESIAN_POINT('Ctrl Pts',(1.09951054676106,3.21523339141517,56.2302870631734));
#10655=CARTESIAN_POINT('Ctrl Pts',(0.871963317456202,3.28425123106222,56.2426242454246));
#10656=CARTESIAN_POINT('Ctrl Pts',(0.596626617109975,3.33711143644126,56.2583497419202));
#10657=CARTESIAN_POINT('Ctrl Pts',(0.553997151889645,3.34445254991414,56.2608076347832));
#10658=CARTESIAN_POINT('Ctrl Pts',(0.488858755129172,3.35439037750868,56.2646141438897));
#10659=CARTESIAN_POINT('Ctrl Pts',(0.466443546566341,3.35758068308,56.265933143475));
#10660=CARTESIAN_POINT('Ctrl Pts',(0.424352783082365,3.36314175720591,56.2684297835563));
#10661=CARTESIAN_POINT('Ctrl Pts',(0.404685716125779,3.3655649094346,56.2696046924258));
#10662=CARTESIAN_POINT('Ctrl Pts',(0.356269047383536,3.37109976620516,56.2725163626944));
#10663=CARTESIAN_POINT('Ctrl Pts',(0.327499133904528,3.37401622150589,56.2742630150445));
#10664=CARTESIAN_POINT('Ctrl Pts',(0.212666046209488,3.38417454836853,56.2812910947432));
#10665=CARTESIAN_POINT('Ctrl Pts',(0.126382319766553,3.38849369004091,56.2866973963907));
#10666=CARTESIAN_POINT('Ctrl Pts',(-0.140661911396912,3.3916478568469,56.3036415191862));
#10667=CARTESIAN_POINT('Ctrl Pts',(-0.321238670000045,3.37932941651606,
56.3153823977885));
#10668=CARTESIAN_POINT('Ctrl Pts',(-0.661177567651374,3.32863545646693,
56.3373372513491));
#10669=CARTESIAN_POINT('Ctrl Pts',(-0.820453630608091,3.29299820261443,
56.3475615430667));
#10670=CARTESIAN_POINT('Ctrl Pts',(-1.02532952170021,3.23136159150946,56.3605289390248));
#10671=CARTESIAN_POINT('Ctrl Pts',(-1.07375993274099,3.21559300717031,56.363581725251));
#10672=CARTESIAN_POINT('Ctrl Pts',(-1.15493389451528,3.18712476341028,56.3686796321921));
#10673=CARTESIAN_POINT('Ctrl Pts',(-1.1878676328728,3.17499719397437,56.3707426428394));
#10674=CARTESIAN_POINT('Ctrl Pts',(-1.25464724890001,3.14922159101854,56.3749169555051));
#10675=CARTESIAN_POINT('Ctrl Pts',(-1.28847299948785,3.13553405772326,56.3770266437697));
#10676=CARTESIAN_POINT('Ctrl Pts',(-1.37418542652807,3.09922933999873,56.382364404));
#10677=CARTESIAN_POINT('Ctrl Pts',(-1.42573962937739,3.07585355763925,56.3855671677636));
#10678=CARTESIAN_POINT('Ctrl Pts',(-1.53790080187587,3.02157096074304,56.3925357426453));
#10679=CARTESIAN_POINT('Ctrl Pts',(-1.59821183464366,2.99010862688449,56.3962831727273));
#10680=CARTESIAN_POINT('Ctrl Pts',(-1.79203410399074,2.88145665785104,56.4083901330433));
#10681=CARTESIAN_POINT('Ctrl Pts',(-1.92123351698479,2.79697035123722,56.4165542558339));
#10682=CARTESIAN_POINT('Ctrl Pts',(-2.18494660965102,2.59760080893612,56.4341125404148));
#10683=CARTESIAN_POINT('Ctrl Pts',(-2.31712704142991,2.48040959806604,56.4434885552329));
#10684=CARTESIAN_POINT('Ctrl Pts',(-2.46656255072167,2.3255074879639,56.4556168562031));
#10685=CARTESIAN_POINT('Ctrl Pts',(-2.49306499252338,2.29707260863191,56.457833941026));
#10686=CARTESIAN_POINT('Ctrl Pts',(-2.53363548422156,2.25201466146652,56.4613445710169));
#10687=CARTESIAN_POINT('Ctrl Pts',(-2.54804296401896,2.2357002930477,56.4626151774843));
#10688=CARTESIAN_POINT('Ctrl Pts',(-2.57550923013788,2.20398839499421,56.4650865620563));
#10689=CARTESIAN_POINT('Ctrl Pts',(-2.58858926817689,2.18861101273915,56.4662858404909));
#10690=CARTESIAN_POINT('Ctrl Pts',(-2.62148235162637,2.14923333011438,56.4693573025594));
#10691=CARTESIAN_POINT('Ctrl Pts',(-2.6411034158455,2.12507558089545,56.4712419134249));
#10692=CARTESIAN_POINT('Ctrl Pts',(-2.73013829121127,2.01231662123332,56.480026685157));
#10693=CARTESIAN_POINT('Ctrl Pts',(-2.79543984358782,1.92056896396365,56.4871392471992));
#10694=CARTESIAN_POINT('Ctrl Pts',(-3.01349154466822,1.57946741330266,56.5130253054));
#10695=CARTESIAN_POINT('Ctrl Pts',(-3.13844384182353,1.31379997801054,56.532040347514));
#10696=CARTESIAN_POINT('Ctrl Pts',(-3.24638103177779,0.977309656638154,
56.5536435438288));
#10697=CARTESIAN_POINT('Ctrl Pts',(-3.26343828280017,0.918746566271449,
56.5573247124549));
#10698=CARTESIAN_POINT('Ctrl Pts',(-3.2883759937193,0.823639586993963,56.5631797327621));
#10699=CARTESIAN_POINT('Ctrl Pts',(-3.29724799814706,0.787371989111304,
56.5653840963834));
#10700=CARTESIAN_POINT('Ctrl Pts',(-3.31327841594486,0.716810886868806,
56.5696201612203));
#10701=CARTESIAN_POINT('Ctrl Pts',(-3.32050793272171,0.682538578430042,
56.5716538443982));
#10702=CARTESIAN_POINT('Ctrl Pts',(-3.33382775125312,0.614163780496667,
56.5756664991972));
#10703=CARTESIAN_POINT('Ctrl Pts',(-3.3399290527832,0.580067814420547,56.5776455854605));
#10704=CARTESIAN_POINT('Ctrl Pts',(-3.35634839301707,0.479440074265641,
56.5834271050173));
#10705=CARTESIAN_POINT('Ctrl Pts',(-3.36520852940889,0.412685912169786,
56.5871861054862));
#10706=CARTESIAN_POINT('Ctrl Pts',(-3.37921317984871,0.276083387277213,
56.5947562725798));
#10707=CARTESIAN_POINT('Ctrl Pts',(-3.38419211761487,0.206263517159003,
56.5985610392712));
#10708=CARTESIAN_POINT('Ctrl Pts',(-3.3870066172248,0.136349687844955,56.6023307114865));
#10709=CARTESIAN_POINT('',(-3.38974984859561,-0.00101313674349031,55.0160178032937));
#10710=CARTESIAN_POINT('Ctrl Pts',(-3.38700661857411,0.136349654327209,
56.2578983182294));
#10711=CARTESIAN_POINT('Ctrl Pts',(-3.38288267634243,0.238790835438136,
56.2518591394859));
#10712=CARTESIAN_POINT('Ctrl Pts',(-3.37410030439886,0.341207785170065,
56.2458199607423));
#10713=CARTESIAN_POINT('Ctrl Pts',(-3.36065963653686,0.443138657591452,
56.2397807819988));
#10714=CARTESIAN_POINT('Ctrl Pts',(-3.34723386195637,0.544956582859223,
56.2337482951242));
#10715=CARTESIAN_POINT('Ctrl Pts',(-3.32916010725762,0.646289071186269,
56.2277158082497));
#10716=CARTESIAN_POINT('Ctrl Pts',(-3.3064905050191,0.746676370804987,56.2216833213752));
#10717=CARTESIAN_POINT('Ctrl Pts',(-3.28383903063338,0.846983395252976,
56.2156556584068));
#10718=CARTESIAN_POINT('Ctrl Pts',(-3.25659911068481,0.946346309143612,
56.2096279954385));
#10719=CARTESIAN_POINT('Ctrl Pts',(-3.22487430571405,1.04431354240254,56.2036003324701));
#10720=CARTESIAN_POINT('Ctrl Pts',(-3.19316270701911,1.14223999425065,56.1975751786734));
#10721=CARTESIAN_POINT('Ctrl Pts',(-3.15697006634594,1.23877150473748,56.1915500248766));
#10722=CARTESIAN_POINT('Ctrl Pts',(-3.11645011480498,1.3334705637666,56.1855248710799));
#10723=CARTESIAN_POINT('Ctrl Pts',(-3.07593603154595,1.42815590805135,56.1795005898731));
#10724=CARTESIAN_POINT('Ctrl Pts',(-3.03109605495282,1.52100892696445,56.1734763086662));
#10725=CARTESIAN_POINT('Ctrl Pts',(-2.98213209040148,1.61161200600446,56.1674520274594));
#10726=CARTESIAN_POINT('Ctrl Pts',(-2.93316192542893,1.702226558324,56.1614269833837));
#10727=CARTESIAN_POINT('Ctrl Pts',(-2.88006694368194,1.79059022110328,56.1554019393081));
#10728=CARTESIAN_POINT('Ctrl Pts',(-2.82309453404155,1.8763108256269,56.1493768952325));
#10729=CARTESIAN_POINT('Ctrl Pts',(-2.76606525586127,1.96211699447279,56.1433458370974));
#10730=CARTESIAN_POINT('Ctrl Pts',(-2.70515106505316,2.04527447374013,56.1373147789623));
#10731=CARTESIAN_POINT('Ctrl Pts',(-2.64064202260133,2.12542108086185,56.1312837208272));
#10732=CARTESIAN_POINT('Ctrl Pts',(-2.57609806547028,2.20561106629106,56.1252493984604));
#10733=CARTESIAN_POINT('Ctrl Pts',(-2.50795567258216,2.28278660859193,56.1192150760937));
#10734=CARTESIAN_POINT('Ctrl Pts',(-2.4365430563558,2.35662109746653,56.1131807537269));
#10735=CARTESIAN_POINT('Ctrl Pts',(-2.36501906131461,2.43057074243397,56.1071370199184));
#10736=CARTESIAN_POINT('Ctrl Pts',(-2.29021497689596,2.50116863066805,56.1010932861099));
#10737=CARTESIAN_POINT('Ctrl Pts',(-2.21249345498554,2.56812728931923,56.0950495523015));
#10738=CARTESIAN_POINT('Ctrl Pts',(-2.1644396452842,2.60952661554948,56.091312821121));
#10739=CARTESIAN_POINT('Ctrl Pts',(-2.11527120872906,2.64953558429001,56.0875760899405));
#10740=CARTESIAN_POINT('Ctrl Pts',(-2.06507922825687,2.68809464928637,56.08383935876));
#10741=CARTESIAN_POINT('Ctrl Pts',(-1.98307867243234,2.75109006672217,56.0777345182878));
#10742=CARTESIAN_POINT('Ctrl Pts',(-1.89805620863826,2.8104349818159,56.0716296778156));
#10743=CARTESIAN_POINT('Ctrl Pts',(-1.81037029782322,2.86582700930455,56.0655248373433));
#10744=CARTESIAN_POINT('Ctrl Pts',(-1.72279875064673,2.92114679219027,56.0594279590598));
#10745=CARTESIAN_POINT('Ctrl Pts',(-1.63257102091373,2.97252371094682,56.0533310807763));
#10746=CARTESIAN_POINT('Ctrl Pts',(-1.54007761224668,3.01969634413074,56.0472342024928));
#10747=CARTESIAN_POINT('Ctrl Pts',(-1.44767845784912,3.06682090662352,56.0411435371581));
#10748=CARTESIAN_POINT('Ctrl Pts',(-1.35301859437778,3.10974951017623,56.0350528718234));
#10749=CARTESIAN_POINT('Ctrl Pts',(-1.25651566281468,3.14826514950717,56.0289622064886));
#10750=CARTESIAN_POINT('Ctrl Pts',(-1.16008037102177,3.18675379288108,56.0228758101558));
#10751=CARTESIAN_POINT('Ctrl Pts',(-1.0618049757545,3.22083546515498,56.016789413823));
#10752=CARTESIAN_POINT('Ctrl Pts',(-0.962129022608679,3.25034041391884,
56.0107030174902));
#10753=CARTESIAN_POINT('Ctrl Pts',(-0.862489258313608,3.27983465046823,
56.004618830915));
#10754=CARTESIAN_POINT('Ctrl Pts',(-0.761450355998017,3.30475534496944,
55.9985346443398));
#10755=CARTESIAN_POINT('Ctrl Pts',(-0.659468267529887,3.32498220545932,
55.9924504577645));
#10756=CARTESIAN_POINT('Ctrl Pts',(-0.55749686814948,3.34520694590352,55.9863669088934));
#10757=CARTESIAN_POINT('Ctrl Pts',(-0.454582898256851,3.36073874762659,
55.9802833600223));
#10758=CARTESIAN_POINT('Ctrl Pts',(-0.351192888352274,3.37150835942472,
55.9741998111513));
#10759=CARTESIAN_POINT('Ctrl Pts',(-0.247787014920056,3.38227962364589,
55.9681153288578));
#10760=CARTESIAN_POINT('Ctrl Pts',(-0.143905381295408,3.38828720196697,
55.9620308465644));
#10761=CARTESIAN_POINT('Ctrl Pts',(-0.0400191221791434,3.38951376046182,
55.955946364271));
#10762=CARTESIAN_POINT('Ctrl Pts',(0.0639742422930276,3.39074158352222,
55.949855608957));
#10763=CARTESIAN_POINT('Ctrl Pts',(0.167971813812484,3.38717853820811,55.943764853643));
#10764=CARTESIAN_POINT('Ctrl Pts',(0.27150301771893,3.37885944867044,55.937674098329));
#10765=CARTESIAN_POINT('Ctrl Pts',(0.375090245811289,3.37053585739609,55.9315800471042));
#10766=CARTESIAN_POINT('Ctrl Pts',(0.478210179753243,3.35745114909732,55.9254859958795));
#10767=CARTESIAN_POINT('Ctrl Pts',(0.580399886191446,3.33969175742447,55.9193919446547));
#10768=CARTESIAN_POINT('Ctrl Pts',(0.682753354140988,3.32190390589082,55.9132881275634));
#10769=CARTESIAN_POINT('Ctrl Pts',(0.784173199516818,3.29942649913459,55.9071843104721));
#10770=CARTESIAN_POINT('Ctrl Pts',(0.884208956675721,3.272396611573,55.9010804933807));
#10771=CARTESIAN_POINT('Ctrl Pts',(0.95792699265596,3.25247783172469,55.8965824876602));
#10772=CARTESIAN_POINT('Ctrl Pts',(1.0308936847203,3.23008790258919,55.8920844819397));
#10773=CARTESIAN_POINT('Ctrl Pts',(1.10293578871009,3.20529838056965,55.8875864762192));
#10774=CARTESIAN_POINT('Ctrl Pts',(1.20071368887821,3.17165323037269,55.8814816357171));
#10775=CARTESIAN_POINT('Ctrl Pts',(1.29711374109057,3.13347380728671,55.875376795215));
#10776=CARTESIAN_POINT('Ctrl Pts',(1.39168599073097,3.09089229280206,55.8692719547129));
#10777=CARTESIAN_POINT('Ctrl Pts',(1.48613489528964,3.04836631490878,55.863175076399));
#10778=CARTESIAN_POINT('Ctrl Pts',(1.57876035039731,3.00144983409531,55.8570781980851));
#10779=CARTESIAN_POINT('Ctrl Pts',(1.66912889298272,2.95032435523796,55.8509813197712));
#10780=CARTESIAN_POINT('Ctrl Pts',(1.75940534662468,2.89925097516627,55.8448906544055));
#10781=CARTESIAN_POINT('Ctrl Pts',(1.84742909133248,2.84397733559493,55.8387999890399));
#10782=CARTESIAN_POINT('Ctrl Pts',(1.93278874106862,2.78473207775872,55.8327093236743));
#10783=CARTESIAN_POINT('Ctrl Pts',(2.0180885614691,2.72552834544925,55.8266229273101));
#10784=CARTESIAN_POINT('Ctrl Pts',(2.10072765029589,2.66235877362975,55.8205365309458));
#10785=CARTESIAN_POINT('Ctrl Pts',(2.18032195116577,2.59549634015629,55.8144501345816));
#10786=CARTESIAN_POINT('Ctrl Pts',(2.25988735413482,2.52865818208887,55.8083659479746));
#10787=CARTESIAN_POINT('Ctrl Pts',(2.33640983951913,2.45813010165325,55.8022817613675));
#10788=CARTESIAN_POINT('Ctrl Pts',(2.40953755496922,2.38422604500768,55.7961975747605));
#10789=CARTESIAN_POINT('Ctrl Pts',(2.48265760565956,2.31032973449277,55.7901140258573));
#10790=CARTESIAN_POINT('Ctrl Pts',(2.55238329355677,2.23305845513715,55.7840304769541));
#10791=CARTESIAN_POINT('Ctrl Pts',(2.61839950318521,2.15276313239972,55.777946928051));
#10792=CARTESIAN_POINT('Ctrl Pts',(2.68442584193768,2.07245548963835,55.7718624457252));
#10793=CARTESIAN_POINT('Ctrl Pts',(2.74674130029062,1.98912321165813,55.7657779633995));
#10794=CARTESIAN_POINT('Ctrl Pts',(2.8050715264326,1.90314970354333,55.7596934810737));
#10795=CARTESIAN_POINT('Ctrl Pts',(2.86346189026644,1.81708755787849,55.7536027257272));
#10796=CARTESIAN_POINT('Ctrl Pts',(2.91785857652049,1.72837909830563,55.7475119703806));
#10797=CARTESIAN_POINT('Ctrl Pts',(2.96803104666488,1.63743603494408,55.741421215034));
#10798=CARTESIAN_POINT('Ctrl Pts',(3.01823066680662,1.54644375925707,55.7353271637765));
#10799=CARTESIAN_POINT('Ctrl Pts',(3.06420132857478,1.45321485426518,55.7292331125191));
#10800=CARTESIAN_POINT('Ctrl Pts',(3.10575975542555,1.35818312612072,55.7231390612616));
#10801=CARTESIAN_POINT('Ctrl Pts',(3.14738478067409,1.26299910730234,55.7170352441376));
#10802=CARTESIAN_POINT('Ctrl Pts',(3.18458329376295,1.16600689329911,55.7109314270136));
#10803=CARTESIAN_POINT('Ctrl Pts',(3.2172211345348,1.0676578262733,55.7048276098895));
#10804=CARTESIAN_POINT('Ctrl Pts',(3.24127250782663,0.995182746182175,55.7003296044859));
#10805=CARTESIAN_POINT('Ctrl Pts',(3.26284826270117,0.921971182530229,55.6958315990823));
#10806=CARTESIAN_POINT('Ctrl Pts',(3.28191251605947,0.848207108807883,55.6913335936787));
#10807=CARTESIAN_POINT('Ctrl Pts',(3.30778714609861,0.74809208820494,55.6852287531929));
#10808=CARTESIAN_POINT('Ctrl Pts',(3.32911973321287,0.646625053760209,55.6791239127071));
#10809=CARTESIAN_POINT('Ctrl Pts',(3.34577231801947,0.544254222284597,55.6730190722213));
#10810=CARTESIAN_POINT('Ctrl Pts',(3.36240318382819,0.442016907130759,55.666922193924));
#10811=CARTESIAN_POINT('Ctrl Pts',(3.37436611445069,0.338878556663255,55.6608253156266));
#10812=CARTESIAN_POINT('Ctrl Pts',(3.3815733877642,0.235300840765542,55.6547284373292));
#10813=CARTESIAN_POINT('Ctrl Pts',(3.38877331659493,0.131828674458836,55.6486377719802));
#10814=CARTESIAN_POINT('Ctrl Pts',(3.39122719565924,0.027918457042437,55.6425471066313));
#10815=CARTESIAN_POINT('Ctrl Pts',(3.38889879706883,-0.0759605537462734,
55.6364564412824));
#10816=CARTESIAN_POINT('Ctrl Pts',(3.38657203047373,-0.17976675481124,55.630370044935));
#10817=CARTESIAN_POINT('Ctrl Pts',(3.37946966156913,-0.283541366856671,
55.6242836485877));
#10818=CARTESIAN_POINT('Ctrl Pts',(3.36760751900137,-0.386813469860425,
55.6181972522404));
#10819=CARTESIAN_POINT('Ctrl Pts',(3.35574968316203,-0.490048078381245,
55.6121130656503));
#10820=CARTESIAN_POINT('Ctrl Pts',(3.33913555703853,-0.592780116503111,
55.6060288790603));
#10821=CARTESIAN_POINT('Ctrl Pts',(3.31783290521502,-0.694542925651456,
55.5999446924703));
#10822=CARTESIAN_POINT('Ctrl Pts',(3.29653248619384,-0.796295068698662,
55.5938611435842));
#10823=CARTESIAN_POINT('Ctrl Pts',(3.2705446062986,-0.897077766664336,55.5877775946982));
#10824=CARTESIAN_POINT('Ctrl Pts',(3.23998813934696,-0.996434603670006,
55.5816940458121));
#10825=CARTESIAN_POINT('Ctrl Pts',(3.20942698399791,-1.09580668538112,55.5756095635035));
#10826=CARTESIAN_POINT('Ctrl Pts',(3.17429597448661,-1.19375206311132,55.5695250811949));
#10827=CARTESIAN_POINT('Ctrl Pts',(3.13476356205984,-1.28983040454236,55.5634405988864));
#10828=CARTESIAN_POINT('Ctrl Pts',(3.09519039223853,-1.38600780147312,55.557349843557));
#10829=CARTESIAN_POINT('Ctrl Pts',(3.05120692044458,-1.48031392231843,55.5512590882276));
#10830=CARTESIAN_POINT('Ctrl Pts',(3.0030293756567,-1.57232936480972,55.5451683328982));
#10831=CARTESIAN_POINT('Ctrl Pts',(2.9548257603921,-1.66439459992664,55.5390742816579));
#10832=CARTESIAN_POINT('Ctrl Pts',(2.90242376668504,-1.75416631857476,55.5329802304176));
#10833=CARTESIAN_POINT('Ctrl Pts',(2.84608412482369,-1.84125235014828,55.5268861791773));
#10834=CARTESIAN_POINT('Ctrl Pts',(2.78965419730395,-1.92847793922409,55.5207823620703));
#10835=CARTESIAN_POINT('Ctrl Pts',(2.72927426508139,-2.01300889616574,55.5146785449634));
#10836=CARTESIAN_POINT('Ctrl Pts',(2.66524677925035,-2.09448434422309,55.5085747278565));
#10837=CARTESIAN_POINT('Ctrl Pts',(2.61806384715454,-2.15452497338836,55.5040767222837));
#10838=CARTESIAN_POINT('Ctrl Pts',(2.5689009892064,-2.2129069919269,55.4995787167109));
#10839=CARTESIAN_POINT('Ctrl Pts',(2.51789186088322,-2.26949898422494,55.495080711138));
#10840=CARTESIAN_POINT('Ctrl Pts',(2.44866060121859,-2.34630748973206,55.4889758706512));
#10841=CARTESIAN_POINT('Ctrl Pts',(2.37579610082697,-2.42007335539983,55.4828710301644));
#10842=CARTESIAN_POINT('Ctrl Pts',(2.29959610820991,-2.49043425964346,55.4767661896776));
#10843=CARTESIAN_POINT('Ctrl Pts',(2.22349549881186,-2.56070339625146,55.4706693113792));
#10844=CARTESIAN_POINT('Ctrl Pts',(2.14406835733114,-2.62757611300103,55.4645724330808));
#10845=CARTESIAN_POINT('Ctrl Pts',(2.06165136586444,-2.69072456935475,55.4584755547824));
#10846=CARTESIAN_POINT('Ctrl Pts',(1.97931836041439,-2.7538086750544,55.4523848894325));
#10847=CARTESIAN_POINT('Ctrl Pts',(1.89400190108035,-2.81317580885546,55.4462942240826));
#10848=CARTESIAN_POINT('Ctrl Pts',(1.8060734048445,-2.86853689514592,55.4402035587327));
#10849=CARTESIAN_POINT('Ctrl Pts',(1.71820653847519,-2.92385917835768,55.4341171623844));
#10850=CARTESIAN_POINT('Ctrl Pts',(1.6277316364979,-2.97518077093345,55.4280307660361));
#10851=CARTESIAN_POINT('Ctrl Pts',(1.53505021852719,-3.02225509993773,55.4219443696878));
#10852=CARTESIAN_POINT('Ctrl Pts',(1.44240244993301,-3.06931233790202,55.4158601830968));
#10853=CARTESIAN_POINT('Ctrl Pts',(1.34755013807224,-3.11212518388724,55.4097759965059));
#10854=CARTESIAN_POINT('Ctrl Pts',(1.25091989776188,-3.15049273477712,55.4036918099149));
#10855=CARTESIAN_POINT('Ctrl Pts',(1.15429978559087,-3.18885626423539,55.3976082610279));
#10856=CARTESIAN_POINT('Ctrl Pts',(1.05590251261699,-3.2227752675427,55.3915247121409));
#10857=CARTESIAN_POINT('Ctrl Pts',(0.956174343943407,-3.25209712131793,
55.3854411632539));
#10858=CARTESIAN_POINT('Ctrl Pts',(0.85643087359044,-3.28142347405882,55.3793566809445));
#10859=CARTESIAN_POINT('Ctrl Pts',(0.755356511711694,-3.3061511553531,55.373272198635));
#10860=CARTESIAN_POINT('Ctrl Pts',(0.65341145691597,-3.32617776591555,55.3671877163256));
#10861=CARTESIAN_POINT('Ctrl Pts',(0.551361298117504,-3.34622502364853,
55.3610969609954));
#10862=CARTESIAN_POINT('Ctrl Pts',(0.448439073729685,-3.36156144925758,
55.3550062056651));
#10863=CARTESIAN_POINT('Ctrl Pts',(0.345113880702074,-3.37213603993771,
55.3489154503349));
#10864=CARTESIAN_POINT('Ctrl Pts',(0.241732774966303,-3.38271635288155,
55.3428213990938));
#10865=CARTESIAN_POINT('Ctrl Pts',(0.13794869279289,-3.38852967418034,55.3367273478528));
#10866=CARTESIAN_POINT('Ctrl Pts',(0.0342325659969947,-3.38957714087248,
55.3306332966117));
#10867=CARTESIAN_POINT('Ctrl Pts',(-0.0696497684363739,-3.39062628615569,
55.324529479504));
#10868=CARTESIAN_POINT('Ctrl Pts',(-0.173463502829106,-3.38689433600581,
55.3184256623963));
#10869=CARTESIAN_POINT('Ctrl Pts',(-0.276740792540085,-3.37843448896738,
55.3123218452886));
#10870=CARTESIAN_POINT('Ctrl Pts',(-0.352847565651834,-3.37220028529186,
55.3078238397249));
#10871=CARTESIAN_POINT('Ctrl Pts',(-0.428663108147057,-3.36339970668902,
55.3033258341611));
#10872=CARTESIAN_POINT('Ctrl Pts',(-0.5040040791703,-3.35207174008548,55.2988278285974));
#10873=CARTESIAN_POINT('Ctrl Pts',(-0.606259312987569,-3.3366970527409,
55.292722988105));
#10874=CARTESIAN_POINT('Ctrl Pts',(-0.707980940545628,-3.3166135056809,
55.2866181476127));
#10875=CARTESIAN_POINT('Ctrl Pts',(-0.808702506194882,-3.29186957806261,
55.2805133071204));
#10876=CARTESIAN_POINT('Ctrl Pts',(-0.90929270656509,-3.26715792250975,
55.2744164288164));
#10877=CARTESIAN_POINT('Ctrl Pts',(-1.00888502671304,-3.23779807174814,
55.2683195505124));
#10878=CARTESIAN_POINT('Ctrl Pts',(-1.1070202940763,-3.20388999982884,55.2622226722084));
#10879=CARTESIAN_POINT('Ctrl Pts',(-1.20505555790891,-3.17001648151091,
55.2561320068529));
#10880=CARTESIAN_POINT('Ctrl Pts',(-1.30163631988751,-3.13160409751842,
55.2500413414974));
#10881=CARTESIAN_POINT('Ctrl Pts',(-1.39631657981158,-3.08880317784143,
55.2439506761418));
#10882=CARTESIAN_POINT('Ctrl Pts',(-1.49093047749865,-3.04603225771003,
55.2378642797878));
#10883=CARTESIAN_POINT('Ctrl Pts',(-1.58364613397871,-2.99887909435195,
55.2317778834338));
#10884=CARTESIAN_POINT('Ctrl Pts',(-1.67403639432774,-2.94754257186663,
55.2256914870798));
#10885=CARTESIAN_POINT('Ctrl Pts',(-1.76439383714003,-2.89622468787408,
55.2196073004831));
#10886=CARTESIAN_POINT('Ctrl Pts',(-1.85242719075477,-2.84072667424631,
55.2135231138865));
#10887=CARTESIAN_POINT('Ctrl Pts',(-1.93773354946284,-2.7812935396657,55.2074389272898));
#10888=CARTESIAN_POINT('Ctrl Pts',(-2.02303096692565,-2.72186663447104,
55.201355378397));
#10889=CARTESIAN_POINT('Ctrl Pts',(-2.10560160738799,-2.65850567278295,
55.1952718295043));
#10890=CARTESIAN_POINT('Ctrl Pts',(-2.18507199485081,-2.59149868605383,
55.1891882806116));
#10891=CARTESIAN_POINT('Ctrl Pts',(-2.26455457576358,-2.5244814181827,55.1831037982964));
#10892=CARTESIAN_POINT('Ctrl Pts',(-2.34093563196606,-2.45381728921244,
55.1770193159811));
#10893=CARTESIAN_POINT('Ctrl Pts',(-2.41387589250341,-2.37983365765149,
55.1709348336659));
#10894=CARTESIAN_POINT('Ctrl Pts',(-2.48689135348432,-2.30577374994526,
55.1648440783299));
#10895=CARTESIAN_POINT('Ctrl Pts',(-2.55645863416792,-2.22838781000726,
55.1587533229939));
#10896=CARTESIAN_POINT('Ctrl Pts',(-2.62227642408051,-2.14803897036612,
55.1526625676579));
#10897=CARTESIAN_POINT('Ctrl Pts',(-2.68812983019447,-2.06764665128794,
55.146568516411));
#10898=CARTESIAN_POINT('Ctrl Pts',(-2.75022944869206,-1.98428858138369,
55.1404744651642));
#10899=CARTESIAN_POINT('Ctrl Pts',(-2.80831644606139,-1.89835818571762,
55.1343804139173));
#10900=CARTESIAN_POINT('Ctrl Pts',(-2.86649652926843,-1.8122900844853,55.1282765968039));
#10901=CARTESIAN_POINT('Ctrl Pts',(-2.92065092356286,-1.72364178784119,
55.1221727796905));
#10902=CARTESIAN_POINT('Ctrl Pts',(-2.97056592221792,-1.63283286476528,
55.1160689625771));
#10903=CARTESIAN_POINT('Ctrl Pts',(-3.00734912437631,-1.56591424180047,
55.1115709570703));
#10904=CARTESIAN_POINT('Ctrl Pts',(-3.04183109545327,-1.49782283125494,
55.1070729515635));
#10905=CARTESIAN_POINT('Ctrl Pts',(-3.07394321690758,-1.42873306174663,
55.1025749460567));
#10906=CARTESIAN_POINT('Ctrl Pts',(-3.12107749964318,-1.32732285953447,
55.0959727580448));
#10907=CARTESIAN_POINT('Ctrl Pts',(-3.16324201953652,-1.22346548226534,
55.0893705700329));
#10908=CARTESIAN_POINT('Ctrl Pts',(-3.20019768663299,-1.11764924236938,
55.082768382021));
#10909=CARTESIAN_POINT('Ctrl Pts',(-3.23702807947291,-1.01219170390749,
55.0761885744519));
#10910=CARTESIAN_POINT('Ctrl Pts',(-3.2686847197901,-0.904788838507579,
55.0696087668829));
#10911=CARTESIAN_POINT('Ctrl Pts',(-3.29497673585062,-0.795948096739492,
55.0630289593138));
#10912=CARTESIAN_POINT('Ctrl Pts',(-3.3212116362351,-0.687343796046599,
55.0564634454435));
#10913=CARTESIAN_POINT('Ctrl Pts',(-3.34210505503976,-0.577308145988027,
55.0498979315732));
#10914=CARTESIAN_POINT('Ctrl Pts',(-3.35751524924152,-0.466365107625599,
55.0433324177029));
#10915=CARTESIAN_POINT('Ctrl Pts',(-3.37287660872133,-0.355773646430945,
55.0367877098679));
#10916=CARTESIAN_POINT('Ctrl Pts',(-3.38278933482319,-0.244280839478064,
55.0302430020329));
#10917=CARTESIAN_POINT('Ctrl Pts',(-3.38716249140841,-0.132420992655877,
55.0236982941979));
#10918=CARTESIAN_POINT('Ctrl Pts',(-3.3888731860247,-0.0886635753286188,
55.0211381305631));
#10919=CARTESIAN_POINT('Ctrl Pts',(-3.3897367464864,-0.0448501340533459,
55.0185779669284));
#10920=CARTESIAN_POINT('Ctrl Pts',(-3.38974984859561,-0.00101313674349148,
55.0160178032937));
#10921=CARTESIAN_POINT('Ctrl Pts',(-3.38974984859583,-0.00101313598912749,
55.0160178032496));
#10922=CARTESIAN_POINT('Ctrl Pts',(-3.38976353983086,0.0447949908273649,
55.01334252192));
#10923=CARTESIAN_POINT('Ctrl Pts',(-3.38884852420672,0.0905956214387927,
55.0106672405903));
#10924=CARTESIAN_POINT('Ctrl Pts',(-3.38700661857411,0.136349654327207,
55.0079919592607));
#10925=CARTESIAN_POINT('Origin',(0.,0.,0.));
#10926=CARTESIAN_POINT('',(-3.38700661857411,0.136349654327214,53.7581562375148));
#10927=CARTESIAN_POINT('',(-3.38700661852469,0.136349655555037,54.0981108245895));
#10928=CARTESIAN_POINT('',(-3.38700661857411,0.136349654327212,0.));
#10929=CARTESIAN_POINT('',(-3.38974995993599,-0.000521165956363422,54.1059382181378));
#10930=CARTESIAN_POINT('Ctrl Pts',(-3.38700661852469,0.136349655555037,
54.0981108245895));
#10931=CARTESIAN_POINT('Ctrl Pts',(-3.38713784720114,0.133089857106149,
54.0982944673588));
#10932=CARTESIAN_POINT('Ctrl Pts',(-3.38726437466028,0.129829749115,54.0984783058417));
#10933=CARTESIAN_POINT('Ctrl Pts',(-3.38836760212715,0.10030397733956,54.1001449274906));
#10934=CARTESIAN_POINT('Ctrl Pts',(-3.38904345575389,0.0740288444827477,
54.1016399154169));
#10935=CARTESIAN_POINT('Ctrl Pts',(-3.38964034157982,0.0316597707542363,
54.1040734266578));
#10936=CARTESIAN_POINT('Ctrl Pts',(-3.38975243379317,0.0155692120963263,
54.105002909413));
#10937=CARTESIAN_POINT('Ctrl Pts',(-3.38974995993599,-0.000521165956363422,
54.1059382181378));
#10938=CARTESIAN_POINT('Ctrl Pts',(-3.38974995973272,-0.000522486388896574,
54.1059382948925));
#10939=CARTESIAN_POINT('Ctrl Pts',(-3.38974880577691,-0.00800903866730812,
54.1063734767157));
#10940=CARTESIAN_POINT('Ctrl Pts',(-3.38972284979861,-0.0154955041731149,
54.1068099170362));
#10941=CARTESIAN_POINT('Ctrl Pts',(-3.38959716225012,-0.0340336658808944,
54.1078939026009));
#10942=CARTESIAN_POINT('Ctrl Pts',(-3.38946818111483,-0.0450849686866558,
54.1085429784608));
#10943=CARTESIAN_POINT('Ctrl Pts',(-3.38895074179065,-0.076326456836172,
54.1103864888572));
#10944=CARTESIAN_POINT('Ctrl Pts',(-3.38843591336309,-0.0965135311733807,
54.1115879235587));
#10945=CARTESIAN_POINT('Ctrl Pts',(-3.38664827058089,-0.148410506838658,
54.1147008318373));
#10946=CARTESIAN_POINT('Ctrl Pts',(-3.3851104633099,-0.180108805124303,
54.1166254674601));
#10947=CARTESIAN_POINT('Ctrl Pts',(-3.37493640676949,-0.342636920141599,
54.1265977433721));
#10948=CARTESIAN_POINT('Ctrl Pts',(-3.3591601978656,-0.472898229193909,
54.1349325326575));
#10949=CARTESIAN_POINT('Ctrl Pts',(-3.31169581089374,-0.735955193926571,
54.1520851067243));
#10950=CARTESIAN_POINT('Ctrl Pts',(-3.27945019515363,-0.868427938849285,
54.1608925568338));
#10951=CARTESIAN_POINT('Ctrl Pts',(-3.1929216021003,-1.14911426306114,54.1796275628981));
#10952=CARTESIAN_POINT('Ctrl Pts',(-3.13608446160491,-1.29622403395978,
54.1894887486311));
#10953=CARTESIAN_POINT('Ctrl Pts',(-3.04797467126933,-1.4841695627637,54.202059048543));
#10954=CARTESIAN_POINT('Ctrl Pts',(-3.02573333417236,-1.52900198653648,
54.2050565907763));
#10955=CARTESIAN_POINT('Ctrl Pts',(-2.98612508286627,-1.60458958345322,
54.210111289979));
#10956=CARTESIAN_POINT('Ctrl Pts',(-2.96925586114434,-1.63559484956421,
54.2121849584143));
#10957=CARTESIAN_POINT('Ctrl Pts',(-2.93381192753878,-1.69838373641629,
54.2163870317253));
#10958=CARTESIAN_POINT('Ctrl Pts',(-2.91519755166542,-1.73013962724154,
54.2185136934568));
#10959=CARTESIAN_POINT('Ctrl Pts',(-2.86579346193715,-1.81136051545903,
54.2239609838004));
#10960=CARTESIAN_POINT('Ctrl Pts',(-2.83423855765408,-1.86034712754012,
54.2272540888061));
#10961=CARTESIAN_POINT('Ctrl Pts',(-2.67311869122726,-2.09685083209188,
54.2432357359045));
#10962=CARTESIAN_POINT('Ctrl Pts',(-2.52613379266629,-2.27178448441025,
54.2552704524063));
#10963=CARTESIAN_POINT('Ctrl Pts',(-2.23571499774619,-2.55408347108543,
54.2767917177553));
#10964=CARTESIAN_POINT('Ctrl Pts',(-2.09927092886332,-2.66736052272165,
54.2862324075508));
#10965=CARTESIAN_POINT('Ctrl Pts',(-1.92713688883577,-2.78884926911087,
54.2981790584023));
#10966=CARTESIAN_POINT('Ctrl Pts',(-1.89936510527903,-2.80783704134662,
54.3001078847219));
#10967=CARTESIAN_POINT('Ctrl Pts',(-1.85407155270942,-2.83782513331666,
54.303263683091));
#10968=CARTESIAN_POINT('Ctrl Pts',(-1.83672290795452,-2.84908436711678,
54.3044747676869));
#10969=CARTESIAN_POINT('Ctrl Pts',(-1.80369647837574,-2.87009143663667,
54.3067868111644));
#10970=CARTESIAN_POINT('Ctrl Pts',(-1.78803997479763,-2.87987132601829,
54.3078855384055));
#10971=CARTESIAN_POINT('Ctrl Pts',(-1.74448566013589,-2.9065856075163,54.3109477343445));
#10972=CARTESIAN_POINT('Ctrl Pts',(-1.7164226706873,-2.92324531258167,54.3129271508577));
#10973=CARTESIAN_POINT('Ctrl Pts',(-1.57046898984507,-3.00706511142262,
54.3232375389886));
#10974=CARTESIAN_POINT('Ctrl Pts',(-1.44887217252678,-3.06750331888508,
54.331874494367));
#10975=CARTESIAN_POINT('Ctrl Pts',(-1.08780944721153,-3.22069878443769,
54.3570592495246));
#10976=CARTESIAN_POINT('Ctrl Pts',(-0.840974019556434,-3.29378615324854,
54.3736484844233));
#10977=CARTESIAN_POINT('Ctrl Pts',(-0.523109897505935,-3.34979615622988,
54.3934548207542));
#10978=CARTESIAN_POINT('Ctrl Pts',(-0.457658201182087,-3.35936424404907,
54.3974587073065));
#10979=CARTESIAN_POINT('Ctrl Pts',(-0.353893554028891,-3.37144382832758,
54.4036916061082));
#10980=CARTESIAN_POINT('Ctrl Pts',(-0.31574864856133,-3.37522993364654,
54.4059586768766));
#10981=CARTESIAN_POINT('Ctrl Pts',(-0.24298056056052,-3.38120812435767,
54.410239568183));
#10982=CARTESIAN_POINT('Ctrl Pts',(-0.208372156989474,-3.38351726861837,
54.4122567031306));
#10983=CARTESIAN_POINT('Ctrl Pts',(-0.12865618115829,-3.38760829510363,
54.4168623881268));
#10984=CARTESIAN_POINT('Ctrl Pts',(-0.0835358145798179,-3.38902115837409,
54.419439438951));
#10985=CARTESIAN_POINT('Ctrl Pts',(0.0635201227786067,-3.39068711676852,
54.4277534010708));
#10986=CARTESIAN_POINT('Ctrl Pts',(0.165444568737296,-3.38724437886605,
54.433380786759));
#10987=CARTESIAN_POINT('Ctrl Pts',(0.322278966059611,-3.3748494623226,54.441927826291));
#10988=CARTESIAN_POINT('Ctrl Pts',(0.377378235597982,-3.36913320449526,
54.4449095825132));
#10989=CARTESIAN_POINT('Ctrl Pts',(0.682306715048204,-3.32992377976773,
54.4613681608745));
#10990=CARTESIAN_POINT('Ctrl Pts',(0.927907043754976,-3.26999979278323,
54.4744086677195));
#10991=CARTESIAN_POINT('Ctrl Pts',(1.20926823591909,-3.16707130870517,54.4911431835702));
#10992=CARTESIAN_POINT('Ctrl Pts',(1.25361457885408,-3.1497810030207,54.4938384630331));
#10993=CARTESIAN_POINT('Ctrl Pts',(1.31925672331664,-3.12258183566324,54.4979352529181));
#10994=CARTESIAN_POINT('Ctrl Pts',(1.34083904836122,-3.1133753710381,54.4992998354579));
#10995=CARTESIAN_POINT('Ctrl Pts',(1.38028847470216,-3.0960609982444,54.5018296021112));
#10996=CARTESIAN_POINT('Ctrl Pts',(1.39818347898119,-3.08802086634257,54.5029909856056));
#10997=CARTESIAN_POINT('Ctrl Pts',(1.44090391316207,-3.06837935004555,54.5057961115482));
#10998=CARTESIAN_POINT('Ctrl Pts',(1.46565982623667,-3.05663165774957,54.5074480160356));
#10999=CARTESIAN_POINT('Ctrl Pts',(1.53727271824638,-3.02157843891935,54.512297997835));
#11000=CARTESIAN_POINT('Ctrl Pts',(1.5837342098592,-2.99748712117677,54.5155345968511));
#11001=CARTESIAN_POINT('Ctrl Pts',(1.82279279452032,-2.86642034419381,54.5325941538459));
#11002=CARTESIAN_POINT('Ctrl Pts',(2.00517936774663,-2.74193245144112,54.5469688649951));
#11003=CARTESIAN_POINT('Ctrl Pts',(2.29869609373423,-2.4965447123013,54.5713981010247));
#11004=CARTESIAN_POINT('Ctrl Pts',(2.4155735618601,-2.38364323040263,54.5815715723823));
#11005=CARTESIAN_POINT('Ctrl Pts',(2.55753489657486,-2.22529896696241,54.5944540617795));
#11006=CARTESIAN_POINT('Ctrl Pts',(2.59030760254701,-2.18706359480978,54.5974710702015));
#11007=CARTESIAN_POINT('Ctrl Pts',(2.64461718845796,-2.12076740422357,54.6025483245134));
#11008=CARTESIAN_POINT('Ctrl Pts',(2.66658824507123,-2.09307470655296,54.6046254465186));
#11009=CARTESIAN_POINT('Ctrl Pts',(2.70783106859896,-2.03938778901376,54.6085715967526));
#11010=CARTESIAN_POINT('Ctrl Pts',(2.72717155828645,-2.01345152556354,54.6104431306776));
#11011=CARTESIAN_POINT('Ctrl Pts',(2.77760456368372,-1.94375894268725,54.6153832920784));
#11012=CARTESIAN_POINT('Ctrl Pts',(2.80803474200271,-1.89953343415626,54.6184271631954));
#11013=CARTESIAN_POINT('Ctrl Pts',(2.99791245774716,-1.60903468323097,54.6378859481037));
#11014=CARTESIAN_POINT('Ctrl Pts',(3.12585818965196,-1.34368354630474,54.6530925818413));
#11015=CARTESIAN_POINT('Ctrl Pts',(3.25723869027443,-0.946761436681349,
54.6755087321998));
#11016=CARTESIAN_POINT('Ctrl Pts',(3.28986257115198,-0.826292746792135,
54.6822935886086));
#11017=CARTESIAN_POINT('Ctrl Pts',(3.3223905741613,-0.673157060422188,54.691191787781));
#11018=CARTESIAN_POINT('Ctrl Pts',(3.32856880262191,-0.641910528181548,
54.6930215753848));
#11019=CARTESIAN_POINT('Ctrl Pts',(3.33796669455495,-0.590589980391987,
54.6960567635597));
#11020=CARTESIAN_POINT('Ctrl Pts',(3.34144785640518,-0.57056496634148,54.6972485036451));
#11021=CARTESIAN_POINT('Ctrl Pts',(3.3482461056926,-0.529260660227407,54.6997240012835));
#11022=CARTESIAN_POINT('Ctrl Pts',(3.3515408487459,-0.507979050074281,54.7010087569635));
#11023=CARTESIAN_POINT('Ctrl Pts',(3.36005180360068,-0.449312529690876,
54.7045732481889));
#11024=CARTESIAN_POINT('Ctrl Pts',(3.36484653321403,-0.411870642975198,
54.7068735996792));
#11025=CARTESIAN_POINT('Ctrl Pts',(3.39054340421553,-0.180613164224188,
54.721206785352));
#11026=CARTESIAN_POINT('Ctrl Pts',(3.39531774969034,0.0146151083274236,
54.7338252575582));
#11027=CARTESIAN_POINT('Ctrl Pts',(3.37009123008838,0.422675504427868,54.7601239349573));
#11028=CARTESIAN_POINT('Ctrl Pts',(3.33670690008856,0.634492524859602,54.773715686223));
#11029=CARTESIAN_POINT('Ctrl Pts',(3.27048444522901,0.892811715667228,54.7899055750597));
#11030=CARTESIAN_POINT('Ctrl Pts',(3.25621133986964,0.943540904387663,54.7930684490225));
#11031=CARTESIAN_POINT('Ctrl Pts',(3.23027614745665,1.02810489802438,54.7983155171613));
#11032=CARTESIAN_POINT('Ctrl Pts',(3.21925099286312,1.062123749796,54.8004193780254));
#11033=CARTESIAN_POINT('Ctrl Pts',(3.19599757127383,1.13018240403059,54.8046164028191));
#11034=CARTESIAN_POINT('Ctrl Pts',(3.18375870078436,1.16421364986842,54.8067089029626));
#11035=CARTESIAN_POINT('Ctrl Pts',(3.15158110395465,1.24938119740011,54.8119339696722));
#11036=CARTESIAN_POINT('Ctrl Pts',(3.13094039559436,1.30024210781025,54.8150434473145));
#11037=CARTESIAN_POINT('Ctrl Pts',(2.9945574572102,1.61419910488277,54.834215131494));
#11038=CARTESIAN_POINT('Ctrl Pts',(2.84698723680335,1.86217098632353,54.8491332806216));
#11039=CARTESIAN_POINT('Ctrl Pts',(2.59115729411746,2.18920982655896,54.871376049095));
#11040=CARTESIAN_POINT('Ctrl Pts',(2.50679787605289,2.28532146109677,54.8783190943877));
#11041=CARTESIAN_POINT('Ctrl Pts',(2.39478347763971,2.39925858605941,54.8873986450716));
#11042=CARTESIAN_POINT('Ctrl Pts',(2.37202145863168,2.42176458598733,54.88923719627));
#11043=CARTESIAN_POINT('Ctrl Pts',(2.33426889581641,2.45804966250731,54.8922829875356));
#11044=CARTESIAN_POINT('Ctrl Pts',(2.31946623613915,2.47202260882605,54.8934763735748));
#11045=CARTESIAN_POINT('Ctrl Pts',(2.28878032926301,2.50047023948265,54.8959506358887));
#11046=CARTESIAN_POINT('Ctrl Pts',(2.27288378142486,2.51492864232572,54.8972324407925));
#11047=CARTESIAN_POINT('Ctrl Pts',(2.22885656753686,2.55421439294252,54.9007799885008));
#11048=CARTESIAN_POINT('Ctrl Pts',(2.2004502217732,2.57872668885708,54.903066043987));
#11049=CARTESIAN_POINT('Ctrl Pts',(1.98638557325339,2.75733401771856,54.9202356966448));
#11050=CARTESIAN_POINT('Ctrl Pts',(1.78516251673025,2.89167877040181,54.9360034257713));
#11051=CARTESIAN_POINT('Ctrl Pts',(1.42983663024125,3.07757940838737,54.9616605820086));
#11052=CARTESIAN_POINT('Ctrl Pts',(1.28320970882871,3.14154597608366,54.9717181023114));
#11053=CARTESIAN_POINT('Ctrl Pts',(1.07922710513936,3.21385762159498,54.9849025248142));
#11054=CARTESIAN_POINT('Ctrl Pts',(1.02538427509494,3.23143924841082,54.9883113785962));
#11055=CARTESIAN_POINT('Ctrl Pts',(0.93616002117095,3.25811927970467,54.9938466638021));
#11056=CARTESIAN_POINT('Ctrl Pts',(0.901028839199804,3.26800918160687,54.995997719879));
#11057=CARTESIAN_POINT('Ctrl Pts',(0.831819202934741,3.28629168828837,55.0001819539615));
#11058=CARTESIAN_POINT('Ctrl Pts',(0.797756683395567,3.29472618808492,55.0022162225077));
#11059=CARTESIAN_POINT('Ctrl Pts',(0.713978129941297,3.31409579507144,55.0071617323388));
#11060=CARTESIAN_POINT('Ctrl Pts',(0.664134252535824,3.32444307863524,55.0100544643011));
#11061=CARTESIAN_POINT('Ctrl Pts',(0.454624170950834,3.36303567616586,55.0220305446317));
#11062=CARTESIAN_POINT('Ctrl Pts',(0.293264970952798,3.38093109274095,55.0307997891587));
#11063=CARTESIAN_POINT('Ctrl Pts',(-0.0228479750814905,3.39317831493441,
55.0476804168612));
#11064=CARTESIAN_POINT('Ctrl Pts',(-0.177150706255401,3.38862753910714,
55.0557859318033));
#11065=CARTESIAN_POINT('Ctrl Pts',(-0.439572508580142,3.36291084421065,
55.0699916897318));
#11066=CARTESIAN_POINT('Ctrl Pts',(-0.547951202497927,3.34695962480425,
55.0759863434842));
#11067=CARTESIAN_POINT('Ctrl Pts',(-0.685686008744834,3.31981855805869,
55.0839760542949));
#11068=CARTESIAN_POINT('Ctrl Pts',(-0.715929645054314,3.31342800755006,
55.085753798977));
#11069=CARTESIAN_POINT('Ctrl Pts',(-0.765735602672148,3.30219018829066,
55.088726369199));
#11070=CARTESIAN_POINT('Ctrl Pts',(-0.785350445078205,3.29758028193596,
55.08990867058));
#11071=CARTESIAN_POINT('Ctrl Pts',(-0.826135171697292,3.28761046747775,
55.0923932576763));
#11072=CARTESIAN_POINT('Ctrl Pts',(-0.847296154261183,3.28222044933866,
55.0936969774007));
#11073=CARTESIAN_POINT('Ctrl Pts',(-0.906312991594718,3.26657924185801,
55.097371074524));
#11074=CARTESIAN_POINT('Ctrl Pts',(-0.944044118462808,3.25587524376736,
55.0997640738037));
#11075=CARTESIAN_POINT('Ctrl Pts',(-1.11363388109118,3.20456848173543,55.1106941666996));
#11076=CARTESIAN_POINT('Ctrl Pts',(-1.24311688582502,3.15659537264405,55.1195142622557));
#11077=CARTESIAN_POINT('Ctrl Pts',(-1.53407295516866,3.02811280572796,55.1399669935222));
#11078=CARTESIAN_POINT('Ctrl Pts',(-1.69279058480409,2.94233164856218,55.1515927918168));
#11079=CARTESIAN_POINT('Ctrl Pts',(-1.93337539575698,2.78636383652742,55.1695807582493));
#11080=CARTESIAN_POINT('Ctrl Pts',(-2.02002687427742,2.72419875000878,55.1761488222825));
#11081=CARTESIAN_POINT('Ctrl Pts',(-2.13888236041718,2.63013506578544,55.1852783433681));
#11082=CARTESIAN_POINT('Ctrl Pts',(-2.17359480176549,2.60152150533854,55.1879607375157));
#11083=CARTESIAN_POINT('Ctrl Pts',(-2.23396281006884,2.54970791407216,55.1926568608095));
#11084=CARTESIAN_POINT('Ctrl Pts',(-2.25985153606307,2.52679074102485,55.1946814066929));
#11085=CARTESIAN_POINT('Ctrl Pts',(-2.31405445044402,2.47730980619854,55.1989452426932));
#11086=CARTESIAN_POINT('Ctrl Pts',(-2.34227217060202,2.45064749230435,55.2011800539229));
#11087=CARTESIAN_POINT('Ctrl Pts',(-2.4178215658101,2.3767652303288,55.207210801943));
#11088=CARTESIAN_POINT('Ctrl Pts',(-2.46422537632135,2.32861937312651,55.2109671265601));
#11089=CARTESIAN_POINT('Ctrl Pts',(-2.70227790250621,2.06653872232165,55.2305992917445));
#11090=CARTESIAN_POINT('Ctrl Pts',(-2.86756756174876,1.83028406060423,55.2454174956946));
#11091=CARTESIAN_POINT('Ctrl Pts',(-3.05059734322658,1.48175497423973,55.266649775665));
#11092=CARTESIAN_POINT('Ctrl Pts',(-3.09562848939659,1.38521565185532,55.2724870155394));
#11093=CARTESIAN_POINT('Ctrl Pts',(-3.14768948445942,1.25833143351853,55.2802951126124));
#11094=CARTESIAN_POINT('Ctrl Pts',(-3.15895349862581,1.22978036261847,55.2820607422084));
#11095=CARTESIAN_POINT('Ctrl Pts',(-3.17695326808241,1.18227636129799,55.2850188315253));
#11096=CARTESIAN_POINT('Ctrl Pts',(-3.18391108312619,1.16340863942326,55.2861990285575));
#11097=CARTESIAN_POINT('Ctrl Pts',(-3.19809913188291,1.12385372406835,55.2886862049741));
#11098=CARTESIAN_POINT('Ctrl Pts',(-3.20529727230949,1.10315664768894,55.2899947260406));
#11099=CARTESIAN_POINT('Ctrl Pts',(-3.22493723041621,1.04486969813699,55.2936967859319));
#11100=CARTESIAN_POINT('Ctrl Pts',(-3.23692146017324,1.00713057643775,55.296113470759));
#11101=CARTESIAN_POINT('Ctrl Pts',(-3.29631979681536,0.808057398542282,
55.3089336589346));
#11102=CARTESIAN_POINT('Ctrl Pts',(-3.33233827125783,0.643579686550158,
55.3197609200745));
#11103=CARTESIAN_POINT('Ctrl Pts',(-3.37207139070138,0.364103150086197,
55.3379338239378));
#11104=CARTESIAN_POINT('Ctrl Pts',(-3.38241663982499,0.250367371407375,
55.3452712400108));
#11105=CARTESIAN_POINT('Ctrl Pts',(-3.38700661431188,0.136349760203539,
55.352502545304));
#11106=CARTESIAN_POINT('',(-3.38974886845295,0.00276971513483697,53.766017803298));
#11107=CARTESIAN_POINT('Ctrl Pts',(-3.38700661857411,0.136349654327207,
55.0079919592607));
#11108=CARTESIAN_POINT('Ctrl Pts',(-3.38271306911003,0.243003980102895,
55.0017557805359));
#11109=CARTESIAN_POINT('Ctrl Pts',(-3.37337953946629,0.349404568150216,
54.9955196018111));
#11110=CARTESIAN_POINT('Ctrl Pts',(-3.35906611853581,0.455060296889049,
54.9892834230863));
#11111=CARTESIAN_POINT('Ctrl Pts',(-3.34474203433446,0.560794737464861,
54.9830425985075));
#11112=CARTESIAN_POINT('Ctrl Pts',(-3.32543072307948,0.665782821158282,
54.9768017739288));
#11113=CARTESIAN_POINT('Ctrl Pts',(-3.30124349820878,0.76954299947065,54.97056094935));
#11114=CARTESIAN_POINT('Ctrl Pts',(-3.27701548930977,0.873478136178295,
54.9643096016142));
#11115=CARTESIAN_POINT('Ctrl Pts',(-3.24789523580502,0.976180845668962,
54.9580582538784));
#11116=CARTESIAN_POINT('Ctrl Pts',(-3.21404426870813,1.07718359683223,54.9518069061426));
#11117=CARTESIAN_POINT('Ctrl Pts',(-3.18016135519291,1.17828166805332,54.9455496587772));
#11118=CARTESIAN_POINT('Ctrl Pts',(-3.14153897217313,1.27767621427922,54.9392924114117));
#11119=CARTESIAN_POINT('Ctrl Pts',(-3.09838652197303,1.37492036967814,54.9330351640462));
#11120=CARTESIAN_POINT('Ctrl Pts',(-3.05515295714101,1.47234731710473,54.926766154792));
#11121=CARTESIAN_POINT('Ctrl Pts',(-3.00737249175788,1.56761544493229,54.9204971455379));
#11122=CARTESIAN_POINT('Ctrl Pts',(-2.95530035426293,1.66030264668626,54.9142281362837));
#11123=CARTESIAN_POINT('Ctrl Pts',(-2.93341033988125,1.6992663665756,54.9115927786945));
#11124=CARTESIAN_POINT('Ctrl Pts',(-2.91076243068349,1.73777434941002,54.9089574211053));
#11125=CARTESIAN_POINT('Ctrl Pts',(-2.88737778668006,1.77579688576327,54.9063220635161));
#11126=CARTESIAN_POINT('Ctrl Pts',(-2.83320695155512,1.86387659086898,54.9002172230302));
#11127=CARTESIAN_POINT('Ctrl Pts',(-2.77491178083767,1.94962221129783,54.8941123825444));
#11128=CARTESIAN_POINT('Ctrl Pts',(-2.71271945693791,2.0326234797548,54.8880075420585));
#11129=CARTESIAN_POINT('Ctrl Pts',(-2.65060824686941,2.11551649448426,54.8819106637611));
#11130=CARTESIAN_POINT('Ctrl Pts',(-2.5846102429144,2.19567193422446,54.8758137854636));
#11131=CARTESIAN_POINT('Ctrl Pts',(-2.51499716353766,2.27270638884515,54.8697169071662));
#11132=CARTESIAN_POINT('Ctrl Pts',(-2.44545502250916,2.34966234245685,54.8636262418172));
#11133=CARTESIAN_POINT('Ctrl Pts',(-2.3723054167313,2.423503320107,54.8575355764682));
#11134=CARTESIAN_POINT('Ctrl Pts',(-2.29586124756975,2.49387774247406,54.8514449111193));
#11135=CARTESIAN_POINT('Ctrl Pts',(-2.21947065880728,2.56420283878162,54.8453585147719));
#11136=CARTESIAN_POINT('Ctrl Pts',(-2.13979041221341,2.63106592315446,54.8392721184245));
#11137=CARTESIAN_POINT('Ctrl Pts',(-2.05717071359343,2.69415176217553,54.8331857220772));
#11138=CARTESIAN_POINT('Ctrl Pts',(-1.97458101129209,2.75721469693816,54.8271015354871));
#11139=CARTESIAN_POINT('Ctrl Pts',(-1.88905431727527,2.8165028530403,54.8210173488971));
#11140=CARTESIAN_POINT('Ctrl Pts',(-1.80097379098454,2.87174136486676,54.814933162307));
#11141=CARTESIAN_POINT('Ctrl Pts',(-1.71290249670896,2.92697408695967,54.808849613421));
#11142=CARTESIAN_POINT('Ctrl Pts',(-1.62227826440829,2.97815778192843,54.8027660645349));
#11143=CARTESIAN_POINT('Ctrl Pts',(-1.52951232516102,3.02506150510705,54.7966825156489));
#11144=CARTESIAN_POINT('Ctrl Pts',(-1.4367321524759,3.07197242490583,54.7905980333403));
#11145=CARTESIAN_POINT('Ctrl Pts',(-1.3418100012344,3.11460187542676,54.7845135510318));
#11146=CARTESIAN_POINT('Ctrl Pts',(-1.24517990421265,3.15276578080976,54.7784290687232));
#11147=CARTESIAN_POINT('Ctrl Pts',(-1.1484501828388,3.1909690326745,54.7723383133939));
#11148=CARTESIAN_POINT('Ctrl Pts',(-1.05000939732259,3.22469738820762,54.7662475580645));
#11149=CARTESIAN_POINT('Ctrl Pts',(-0.950309642682163,3.25381570552564,
54.7601568027352));
#11150=CARTESIAN_POINT('Ctrl Pts',(-0.850555937178876,3.28294977973644,
54.7540627514949));
#11151=CARTESIAN_POINT('Ctrl Pts',(-0.749542320676296,3.30746874575644,
54.7479687002547));
#11152=CARTESIAN_POINT('Ctrl Pts',(-0.647732138507999,3.32728840638197,
54.7418746490145));
#11153=CARTESIAN_POINT('Ctrl Pts',(-0.545758803024913,3.34713982849992,
54.7357708319076));
#11154=CARTESIAN_POINT('Ctrl Pts',(-0.442986774797963,3.36227683979656,
54.7296670148008));
#11155=CARTESIAN_POINT('Ctrl Pts',(-0.339885794689353,3.3726670023986,54.7235631976939));
#11156=CARTESIAN_POINT('Ctrl Pts',(-0.263908946927662,3.38032368811976,
54.7190651921211));
#11157=CARTESIAN_POINT('Ctrl Pts',(-0.187753578591885,3.38540370428563,
54.7145671865483));
#11158=CARTESIAN_POINT('Ctrl Pts',(-0.111607059801464,3.38791217812718,
54.7100691809754));
#11159=CARTESIAN_POINT('Ctrl Pts',(-0.00825851019702291,3.39131676099405,
54.7039643404726));
#11160=CARTESIAN_POINT('Ctrl Pts',(0.0954183339104613,3.38999373153248,
54.6978594999697));
#11161=CARTESIAN_POINT('Ctrl Pts',(0.198955952643701,3.38390626220757,54.6917546594668));
#11162=CARTESIAN_POINT('Ctrl Pts',(0.302358533283741,3.3778267324148,54.6856577811523));
#11163=CARTESIAN_POINT('Ctrl Pts',(0.405621826601226,3.36699514171919,54.6795609028378));
#11164=CARTESIAN_POINT('Ctrl Pts',(0.508276146323263,3.35142662482394,54.6734640245232));
#11165=CARTESIAN_POINT('Ctrl Pts',(0.610825857430051,3.33587397283334,54.6673733591572));
#11166=CARTESIAN_POINT('Ctrl Pts',(0.7127674087945,3.31559405745615,54.6612826937911));
#11167=CARTESIAN_POINT('Ctrl Pts',(0.813634945909873,3.29065392244372,54.655192028425));
#11168=CARTESIAN_POINT('Ctrl Pts',(0.914431784070129,3.26573126819404,54.6491056320606));
#11169=CARTESIAN_POINT('Ctrl Pts',(1.01415569145816,3.23615499222817,54.6430192356961));
#11170=CARTESIAN_POINT('Ctrl Pts',(1.1123505508037,3.20204330305302,54.6369328393316));
#11171=CARTESIAN_POINT('Ctrl Pts',(1.21050975903522,3.16794399863741,54.6308486527245));
#11172=CARTESIAN_POINT('Ctrl Pts',(1.30714061946752,3.12931269383448,54.6247644661173));
#11173=CARTESIAN_POINT('Ctrl Pts',(1.40180250672691,3.0863173515752,54.6186802795102));
#11174=CARTESIAN_POINT('Ctrl Pts',(1.49645447215617,3.04332651580206,54.6125967306071));
#11175=CARTESIAN_POINT('Ctrl Pts',(1.58913748587239,2.99597272889506,54.606513181704));
#11176=CARTESIAN_POINT('Ctrl Pts',(1.67943207110619,2.9444715962359,54.6004296328009));
#11177=CARTESIAN_POINT('Ctrl Pts',(1.7697405105878,2.89296256155855,54.5943451504753));
#11178=CARTESIAN_POINT('Ctrl Pts',(1.85765942238197,2.83730512851825,54.5882606681498));
#11179=CARTESIAN_POINT('Ctrl Pts',(1.94279584416735,2.77775977550005,54.5821761858242));
#11180=CARTESIAN_POINT('Ctrl Pts',(2.02802004047452,2.71815303201257,54.576085430478));
#11181=CARTESIAN_POINT('Ctrl Pts',(2.11045566726323,2.65465060912955,54.5699946751318));
#11182=CARTESIAN_POINT('Ctrl Pts',(2.1897406136349,2.58755504434164,54.5639039197857));
#11183=CARTESIAN_POINT('Ctrl Pts',(2.26906846373453,2.52042317190655,54.5578098685287));
#11184=CARTESIAN_POINT('Ctrl Pts',(2.34524192418938,2.44969457519158,54.5517158172718));
#11185=CARTESIAN_POINT('Ctrl Pts',(2.41793517031265,2.37570927822938,54.5456217660148));
#11186=CARTESIAN_POINT('Ctrl Pts',(2.49074490914241,2.30160541801759,54.5395179488916));
#11187=CARTESIAN_POINT('Ctrl Pts',(2.56006300777758,2.22423475072808,54.5334141317683));
#11188=CARTESIAN_POINT('Ctrl Pts',(2.62560328529656,2.14397118701253,54.527310314645));
#11189=CARTESIAN_POINT('Ctrl Pts',(2.67390101710397,2.08482361820466,54.5228123092416));
#11190=CARTESIAN_POINT('Ctrl Pts',(2.72014806194289,2.0241057699486,54.5183143038382));
#11191=CARTESIAN_POINT('Ctrl Pts',(2.76424533668976,1.96197675345273,54.5138162984348));
#11192=CARTESIAN_POINT('Ctrl Pts',(2.82409560438845,1.87765321440233,54.5077114579645));
#11193=CARTESIAN_POINT('Ctrl Pts',(2.88018373319809,1.79044793869892,54.5016066174942));
#11194=CARTESIAN_POINT('Ctrl Pts',(2.93222110601276,1.70073056300913,54.4955017770239));
#11195=CARTESIAN_POINT('Ctrl Pts',(2.98419060950876,1.61113020047412,54.4894048987419));
#11196=CARTESIAN_POINT('Ctrl Pts',(3.03211964795986,1.51902461827581,54.48330802046));
#11197=CARTESIAN_POINT('Ctrl Pts',(3.07576175020044,1.42481392416833,54.477211142178));
#11198=CARTESIAN_POINT('Ctrl Pts',(3.1193593794969,1.33069923430259,54.4711204768444));
#11199=CARTESIAN_POINT('Ctrl Pts',(3.15867858115272,1.23448408403791,54.4650298115108));
#11200=CARTESIAN_POINT('Ctrl Pts',(3.19351829436629,1.13659401988918,54.4589391461772));
#11201=CARTESIAN_POINT('Ctrl Pts',(3.22833358811568,1.03877256775513,54.452852749845));
#11202=CARTESIAN_POINT('Ctrl Pts',(3.25867549433964,0.93927893765865,54.4467663535128));
#11203=CARTESIAN_POINT('Ctrl Pts',(3.28439099945326,0.838558778625809,54.4406799571806));
#11204=CARTESIAN_POINT('Ctrl Pts',(3.31009716816831,0.737875187552442,54.4345957706055));
#11205=CARTESIAN_POINT('Ctrl Pts',(3.33118016863909,0.635966366107156,54.4285115840305));
#11206=CARTESIAN_POINT('Ctrl Pts',(3.34753703262397,0.533292487956728,54.4224273974555));
#11207=CARTESIAN_POINT('Ctrl Pts',(3.36389218219153,0.430629371397037,54.4163438485843));
#11208=CARTESIAN_POINT('Ctrl Pts',(3.37552211319775,0.327201779484954,54.4102602997131));
#11209=CARTESIAN_POINT('Ctrl Pts',(3.38237526160712,0.223478527308951,54.4041767508419));
#11210=CARTESIAN_POINT('Ctrl Pts',(3.38922946152187,0.119739360468459,54.3980922685479));
#11211=CARTESIAN_POINT('Ctrl Pts',(3.3913053945124,0.015704869540343,54.392007786254));
#11212=CARTESIAN_POINT('Ctrl Pts',(3.38860355077158,-0.0881534922635265,
54.3859233039601));
#11213=CARTESIAN_POINT('Ctrl Pts',(3.38589892146543,-0.192118930670961,
54.3798325486451));
#11214=CARTESIAN_POINT('Ctrl Pts',(3.37840668973926,-0.295907449474564,
54.37374179333));
#11215=CARTESIAN_POINT('Ctrl Pts',(3.36617944540213,-0.399050126991812,
54.367651038015));
#11216=CARTESIAN_POINT('Ctrl Pts',(3.35394558449486,-0.502248618455593,
54.3615569867889));
#11217=CARTESIAN_POINT('Ctrl Pts',(3.33697167683054,-0.604800150975558,
54.3554629355627));
#11218=CARTESIAN_POINT('Ctrl Pts',(3.31536159593447,-0.706245389863055,
54.3493688843366));
#11219=CARTESIAN_POINT('Ctrl Pts',(3.29371688435196,-0.807853197242361,
54.3432650672435));
#11220=CARTESIAN_POINT('Ctrl Pts',(3.26742126667447,-0.90835075610087,54.3371612501503));
#11221=CARTESIAN_POINT('Ctrl Pts',(3.23662874963644,-1.00729310507264,54.3310574330571));
#11222=CARTESIAN_POINT('Ctrl Pts',(3.21393722469607,-1.08020539011184,54.3265594273362));
#11223=CARTESIAN_POINT('Ctrl Pts',(3.18880472242233,-1.15227344406592,54.3220614216151));
#11224=CARTESIAN_POINT('Ctrl Pts',(3.16130929773415,-1.22332685189184,54.3175634158941));
#11225=CARTESIAN_POINT('Ctrl Pts',(3.12399160808946,-1.31976286084666,54.3114585754191));
#11226=CARTESIAN_POINT('Ctrl Pts',(3.08219497809912,-1.41465058412122,54.3053537349439));
#11227=CARTESIAN_POINT('Ctrl Pts',(3.03606850574177,-1.50754538603087,54.2992488944689));
#11228=CARTESIAN_POINT('Ctrl Pts',(2.99000219346137,-1.60031903064957,54.2931520161824));
#11229=CARTESIAN_POINT('Ctrl Pts',(2.93961745443416,-1.69110454202663,54.2870551378959));
#11230=CARTESIAN_POINT('Ctrl Pts',(2.8851120512839,-1.77947562895265,54.2809582596094));
#11231=CARTESIAN_POINT('Ctrl Pts',(2.83066219119295,-1.86775666241169,54.2748675942716));
#11232=CARTESIAN_POINT('Ctrl Pts',(2.77210024035554,-1.95362780237237,54.2687769289338));
#11233=CARTESIAN_POINT('Ctrl Pts',(2.70967022941156,-2.03668660091353,54.262686263596));
#11234=CARTESIAN_POINT('Ctrl Pts',(2.64728397622073,-2.11968718279976,54.25659986726));
#11235=CARTESIAN_POINT('Ctrl Pts',(2.5810353103908,-2.19987900273196,54.250513470924));
#11236=CARTESIAN_POINT('Ctrl Pts',(2.51121153426146,-2.27688859909575,54.244427074588));
#11237=CARTESIAN_POINT('Ctrl Pts',(2.44141310870103,-2.35387023597084,54.2383428880095));
#11238=CARTESIAN_POINT('Ctrl Pts',(2.36804243931463,-2.4276716294355,54.2322587014309));
#11239=CARTESIAN_POINT('Ctrl Pts',(2.29142654994989,-2.49795304773424,54.2261745148524));
#11240=CARTESIAN_POINT('Ctrl Pts',(2.21481869095487,-2.56822709960051,54.220090965978));
#11241=CARTESIAN_POINT('Ctrl Pts',(2.13496660323843,-2.63498162123575,54.2140074171035));
#11242=CARTESIAN_POINT('Ctrl Pts',(2.05223287463767,-2.69791498953477,54.2079238682291));
#11243=CARTESIAN_POINT('Ctrl Pts',(1.96948645188116,-2.76085801394373,54.2018393859323));
#11244=CARTESIAN_POINT('Ctrl Pts',(1.88385784983554,-2.81997846151331,54.1957549036354));
#11245=CARTESIAN_POINT('Ctrl Pts',(1.79574057163204,-2.87501667158551,54.1896704213386));
#11246=CARTESIAN_POINT('Ctrl Pts',(1.70753244568139,-2.93011162532359,54.183579666021));
#11247=CARTESIAN_POINT('Ctrl Pts',(1.61683088271967,-2.98111571003608,54.1774889107035));
#11248=CARTESIAN_POINT('Ctrl Pts',(1.52405601427245,-3.02781411712476,54.171398155386));
#11249=CARTESIAN_POINT('Ctrl Pts',(1.43123094225041,-3.07453779427863,54.1653041041577));
#11250=CARTESIAN_POINT('Ctrl Pts',(1.3363307199609,-3.1169509783585,54.1592100529293));
#11251=CARTESIAN_POINT('Ctrl Pts',(1.23979577237874,-3.15488692432737,54.153116001701));
#11252=CARTESIAN_POINT('Ctrl Pts',(1.14310612517395,-3.19288366358066,54.147012184606));
#11253=CARTESIAN_POINT('Ctrl Pts',(1.04477692425027,-3.22638869459226,54.1409083675111));
#11254=CARTESIAN_POINT('Ctrl Pts',(0.945264261161252,-3.2552850165648,54.1348045504161));
#11255=CARTESIAN_POINT('Ctrl Pts',(0.871931702601138,-3.27657920322853,
54.1303065447286));
#11256=CARTESIAN_POINT('Ctrl Pts',(0.797956780170471,-3.29537169747829,
54.125808539041));
#11257=CARTESIAN_POINT('Ctrl Pts',(0.723524692469719,-3.3116335971672,54.1213105333535));
#11258=CARTESIAN_POINT('Ctrl Pts',(0.622503025979026,-3.33370477987382,
54.1152056927601));
#11259=CARTESIAN_POINT('Ctrl Pts',(0.520302028742421,-3.35118605235059,
54.1091008521669));
#11260=CARTESIAN_POINT('Ctrl Pts',(0.417374812849767,-3.36395649913887,
54.1029960115735));
#11261=CARTESIAN_POINT('Ctrl Pts',(0.314581838931188,-3.37671029017705,
54.0968991331683));
#11262=CARTESIAN_POINT('Ctrl Pts',(0.21106494988949,-3.38476541843064,54.0908022547631));
#11263=CARTESIAN_POINT('Ctrl Pts',(0.107288801997741,-3.38805167839363,
54.0847053763579));
#11264=CARTESIAN_POINT('Ctrl Pts',(0.00361840590228503,-3.39133458953417,
54.078614710901));
#11265=CARTESIAN_POINT('Ctrl Pts',(-0.100310298885308,-3.38985828274735,
54.072524045444));
#11266=CARTESIAN_POINT('Ctrl Pts',(-0.204027020455333,-3.38360429681488,
54.0664333799871));
#11267=CARTESIAN_POINT('Ctrl Pts',(-0.307671046049174,-3.37735469435699,
54.060346983532));
#11268=CARTESIAN_POINT('Ctrl Pts',(-0.411102958675252,-3.36633409778358,
54.0542605870769));
#11269=CARTESIAN_POINT('Ctrl Pts',(-0.513852773378347,-3.35057612803998,
54.0481741906218));
#11270=CARTESIAN_POINT('Ctrl Pts',(-0.616565283220748,-3.33482387946354,
54.0420900039242));
#11271=CARTESIAN_POINT('Ctrl Pts',(-0.718595765519508,-3.31433774092562,
54.0360058172266));
#11272=CARTESIAN_POINT('Ctrl Pts',(-0.819480457211773,-3.28920307107177,
54.0299216305289));
#11273=CARTESIAN_POINT('Ctrl Pts',(-0.920354574836653,-3.26407103566809,
54.0238380815356));
#11274=CARTESIAN_POINT('Ctrl Pts',(-1.02008272615848,-3.23429154118383,
54.0177545325423));
#11275=CARTESIAN_POINT('Ctrl Pts',(-1.11821331572462,-3.20000063172434,
54.0116709835489));
#11276=CARTESIAN_POINT('Ctrl Pts',(-1.21635896184113,-3.16570446087991,
54.0055865011335));
#11277=CARTESIAN_POINT('Ctrl Pts',(-1.31290615587972,-3.12689564073215,
53.999502018718));
#11278=CARTESIAN_POINT('Ctrl Pts',(-1.40742124877484,-3.08375914931712,
53.9934175363026));
#11279=CARTESIAN_POINT('Ctrl Pts',(-1.50203378545856,-3.04057818476007,
53.9873267808677));
#11280=CARTESIAN_POINT('Ctrl Pts',(-1.59460964780646,-2.99306081653175,
53.9812360254328));
#11281=CARTESIAN_POINT('Ctrl Pts',(-1.68473790812533,-2.941438974962,53.9751452699978));
#11282=CARTESIAN_POINT('Ctrl Pts',(-1.77491493984307,-2.88978919909709,
53.9690512186526));
#11283=CARTESIAN_POINT('Ctrl Pts',(-1.86264137067453,-2.83403075481871,
53.9629571673074));
#11284=CARTESIAN_POINT('Ctrl Pts',(-1.94753516753801,-2.77443901243165,
53.9568631159621));
#11285=CARTESIAN_POINT('Ctrl Pts',(-2.03256500876364,-2.71475177283652,
53.9507592987523));
#11286=CARTESIAN_POINT('Ctrl Pts',(-2.11475281020638,-2.65121922559731,
53.9446554815424));
#11287=CARTESIAN_POINT('Ctrl Pts',(-2.19374938756521,-2.58415724890287,
53.9385516643325));
#11288=CARTESIAN_POINT('Ctrl Pts',(-2.25196328040394,-2.534738161958,53.934053659826));
#11289=CARTESIAN_POINT('Ctrl Pts',(-2.30844489606716,-2.48340327098839,
53.9295556553194));
#11290=CARTESIAN_POINT('Ctrl Pts',(-2.36306796596053,-2.43029110411719,
53.9250576508129));
#11291=CARTESIAN_POINT('Ctrl Pts',(-2.43614074560596,-2.35923955623008,
53.9190403820509));
#11292=CARTESIAN_POINT('Ctrl Pts',(-2.50614531578541,-2.28475379901223,
53.913023113289));
#11293=CARTESIAN_POINT('Ctrl Pts',(-2.57273549547598,-2.20713323857396,
53.907005844527));
#11294=CARTESIAN_POINT('Ctrl Pts',(-2.63922143882549,-2.12963418078441,
53.9009979948428));
#11295=CARTESIAN_POINT('Ctrl Pts',(-2.70230333681151,-2.04901041047589,
53.8949901451586));
#11296=CARTESIAN_POINT('Ctrl Pts',(-2.76167070345194,-1.96559914229613,
53.8889822954743));
#11297=CARTESIAN_POINT('Ctrl Pts',(-2.82098532482678,-1.8822619813194,53.8829797834974));
#11298=CARTESIAN_POINT('Ctrl Pts',(-2.87659171419398,-1.7961425973199,53.8769772715205));
#11299=CARTESIAN_POINT('Ctrl Pts',(-2.92821901061884,-1.70761192557046,
53.8709747595436));
#11300=CARTESIAN_POINT('Ctrl Pts',(-2.97981472197077,-1.61913541601653,
53.8649759198446));
#11301=CARTESIAN_POINT('Ctrl Pts',(-3.0274359546713,-1.5282509288324,53.8589770801455));
#11302=CARTESIAN_POINT('Ctrl Pts',(-3.0708552501005,-1.43535817670371,53.8529782404465));
#11303=CARTESIAN_POINT('Ctrl Pts',(-3.11425999142334,-1.34249656213682,
53.8469814115528));
#11304=CARTESIAN_POINT('Ctrl Pts',(-3.15346540869544,-1.24762841971144,
53.8409845826591));
#11305=CARTESIAN_POINT('Ctrl Pts',(-3.18829058916242,-1.15117686806083,
53.8349877537654));
#11306=CARTESIAN_POINT('Ctrl Pts',(-3.22312809554013,-1.05469117866279,
53.8289888023737));
#11307=CARTESIAN_POINT('Ctrl Pts',(-3.25358211035393,-0.956621372797933,
53.8229898509819));
#11308=CARTESIAN_POINT('Ctrl Pts',(-3.27952057482157,-0.857408806708909,
53.8169908995902));
#11309=CARTESIAN_POINT('Ctrl Pts',(-3.30546295820986,-0.758181251059746,
53.8109910418451));
#11310=CARTESIAN_POINT('Ctrl Pts',(-3.3268883330814,-0.657811021334741,
53.8049911841));
#11311=CARTESIAN_POINT('Ctrl Pts',(-3.34371548730905,-0.556751113541406,
53.7989913263549));
#11312=CARTESIAN_POINT('Ctrl Pts',(-3.36056098266848,-0.455581053249218,
53.7929849289311));
#11313=CARTESIAN_POINT('Ctrl Pts',(-3.3727981863967,-0.353720250879779,
53.7869785315074));
#11314=CARTESIAN_POINT('Ctrl Pts',(-3.38039766334347,-0.251628098911874,
53.7809721340836));
#11315=CARTESIAN_POINT('Ctrl Pts',(-3.38670455492597,-0.166900671169774,
53.7759873571551));
#11316=CARTESIAN_POINT('Ctrl Pts',(-3.3898181440983,-0.082014108835823,
53.7710025802265));
#11317=CARTESIAN_POINT('Ctrl Pts',(-3.38974886845295,0.00276971513482787,
53.766017803298));
#11318=CARTESIAN_POINT('Ctrl Pts',(-3.38974886845228,0.00276971595823088,
53.7660178032496));
#11319=CARTESIAN_POINT('Ctrl Pts',(-3.3897124498917,0.0473409919946466,
53.763397281338));
#11320=CARTESIAN_POINT('Ctrl Pts',(-3.38879693886487,0.0918770320527466,
53.7607767594264));
#11321=CARTESIAN_POINT('Ctrl Pts',(-3.38700661857411,0.136349654327203,
53.7581562375148));
#11322=CARTESIAN_POINT('Origin',(0.,0.,0.));
#11323=CARTESIAN_POINT('',(-3.38743469189442,0.136371088936278,52.5078428482942));
#11324=CARTESIAN_POINT('',(-3.3870066183502,0.136349659889395,52.8536715661706));
#11325=CARTESIAN_POINT('',(-3.38700661857411,0.136349654327212,0.));
#11326=CARTESIAN_POINT('Ctrl Pts',(-3.3870066183502,0.136349659889395,52.8536715661706));
#11327=CARTESIAN_POINT('Ctrl Pts',(-3.38885798329129,0.090360654023626,
52.8562620823228));
#11328=CARTESIAN_POINT('Ctrl Pts',(-3.38977266289487,0.0443345664023467,
52.8588265392501));
#11329=CARTESIAN_POINT('Ctrl Pts',(-3.38962280610553,-0.254445741724597,
52.8753257019146));
#11330=CARTESIAN_POINT('Ctrl Pts',(-3.3612305356205,-0.50637572230606,52.8884778259417));
#11331=CARTESIAN_POINT('Ctrl Pts',(-3.27688841398311,-0.876665695222036,
52.9088225462481));
#11332=CARTESIAN_POINT('Ctrl Pts',(-3.24174102107433,-0.998824148034817,
52.9157237313064));
#11333=CARTESIAN_POINT('Ctrl Pts',(-3.18915375802687,-1.14923855903693,
52.9247744573728));
#11334=CARTESIAN_POINT('Ctrl Pts',(-3.17804464081704,-1.17961140085019,
52.9266313154987));
#11335=CARTESIAN_POINT('Ctrl Pts',(-3.15993345097052,-1.22701445647214,
52.9295822425549));
#11336=CARTESIAN_POINT('Ctrl Pts',(-3.15322400662735,-1.24415522370565,
52.9306602736426));
#11337=CARTESIAN_POINT('Ctrl Pts',(-3.13865471048719,-1.28050078342945,
52.9329712903503));
#11338=CARTESIAN_POINT('Ctrl Pts',(-3.13075750988737,-1.2996895806954,52.9342065064485));
#11339=CARTESIAN_POINT('Ctrl Pts',(-3.10946731904312,-1.35010082885317,
52.9374892526451));
#11340=CARTESIAN_POINT('Ctrl Pts',(-3.09578051594554,-1.38119588156737,
52.9395525888828));
#11341=CARTESIAN_POINT('Ctrl Pts',(-3.00851727444757,-1.57163354422528,
52.9524048891755));
#11342=CARTESIAN_POINT('Ctrl Pts',(-2.9231296558358,-1.72525696214465,52.9636985676011));
#11343=CARTESIAN_POINT('Ctrl Pts',(-2.69980866555869,-2.06249284571376,
52.9897377104267));
#11344=CARTESIAN_POINT('Ctrl Pts',(-2.55433591656216,-2.24014269858376,
53.0043896339951));
#11345=CARTESIAN_POINT('Ctrl Pts',(-2.35082654683572,-2.44282686540813,
53.0219095429194));
#11346=CARTESIAN_POINT('Ctrl Pts',(-2.30856082778187,-2.48280810181074,
53.0254145565268));
#11347=CARTESIAN_POINT('Ctrl Pts',(-2.23791751802748,-2.54626857259377,
53.031062758679));
#11348=CARTESIAN_POINT('Ctrl Pts',(-2.2101508069525,-2.57040697745637,53.0332326016579));
#11349=CARTESIAN_POINT('Ctrl Pts',(-2.15497811275992,-2.61681501248026,
53.0374491577784));
#11350=CARTESIAN_POINT('Ctrl Pts',(-2.12760633045955,-2.63911782888246,
53.0394970426046));
#11351=CARTESIAN_POINT('Ctrl Pts',(-2.06056113415274,-2.69202580007891,
53.044411405192));
#11352=CARTESIAN_POINT('Ctrl Pts',(-2.02054737518682,-2.72218731236242,
53.0472606428668));
#11353=CARTESIAN_POINT('Ctrl Pts',(-1.85128611980178,-2.84398361657381,
53.0589926042189));
#11354=CARTESIAN_POINT('Ctrl Pts',(-1.71635952028096,-2.92739135329188,
53.0675755975238));
#11355=CARTESIAN_POINT('Ctrl Pts',(-1.39292525994255,-3.0972508890093,53.0870878916235));
#11356=CARTESIAN_POINT('Ctrl Pts',(-1.20135985671553,-3.17646472593229,
53.0978835547358));
#11357=CARTESIAN_POINT('Ctrl Pts',(-0.937176706167467,-3.25836887632998,
53.1130638783348));
#11358=CARTESIAN_POINT('Ctrl Pts',(-0.869953025628567,-3.27695718339984,
53.1169533846755));
#11359=CARTESIAN_POINT('Ctrl Pts',(-0.775403481268927,-3.29998721937711,
53.1225202139044));
#11360=CARTESIAN_POINT('Ctrl Pts',(-0.748520558821123,-3.30618860241921,
53.1241137448057));
#11361=CARTESIAN_POINT('Ctrl Pts',(-0.702376320504877,-3.31624159008216,
53.1268719367306));
#11362=CARTESIAN_POINT('Ctrl Pts',(-0.683152160469688,-3.3202550936674,
53.128027914092));
#11363=CARTESIAN_POINT('Ctrl Pts',(-0.640995870128654,-3.32867459540301,
53.1305790841751));
#11364=CARTESIAN_POINT('Ctrl Pts',(-0.618052515149012,-3.33301084428786,
53.1319776609449));
#11365=CARTESIAN_POINT('Ctrl Pts',(-0.54881970116538,-3.34535630569313,
53.136224632438));
#11366=CARTESIAN_POINT('Ctrl Pts',(-0.502408386572499,-3.35264033715182,
53.1391074229554));
#11367=CARTESIAN_POINT('Ctrl Pts',(-0.226705302833743,-3.39005757404586,
53.1563864938663));
#11368=CARTESIAN_POINT('Ctrl Pts',(0.0050255618206228,-3.39762513213806,
53.1714903160061));
#11369=CARTESIAN_POINT('Ctrl Pts',(0.401305076754971,-3.37000181387177,
53.196880230899));
#11370=CARTESIAN_POINT('Ctrl Pts',(0.565838787195996,-3.3463108943855,53.2073004596762));
#11371=CARTESIAN_POINT('Ctrl Pts',(0.777804374637566,-3.29970099556454,
53.2204556983712));
#11372=CARTESIAN_POINT('Ctrl Pts',(0.827364991889574,-3.28762435433156,
53.2235133426087));
#11373=CARTESIAN_POINT('Ctrl Pts',(0.910547954114985,-3.26535448506558,
53.2286168824168));
#11374=CARTESIAN_POINT('Ctrl Pts',(0.944317431691197,-3.25574910196942,
53.230680760338));
#11375=CARTESIAN_POINT('Ctrl Pts',(1.01284941787929,-3.23509984260165,53.2348548808183));
#11376=CARTESIAN_POINT('Ctrl Pts',(1.04759514365871,-3.22401605124798,53.2369635412927));
#11377=CARTESIAN_POINT('Ctrl Pts',(1.13569381875675,-3.19433814031534,53.2422946214143));
#11378=CARTESIAN_POINT('Ctrl Pts',(1.1887741018071,-3.1749666529573,53.245491866065));
#11379=CARTESIAN_POINT('Ctrl Pts',(1.41178798794155,-3.08720080825328,53.2588960860065));
#11380=CARTESIAN_POINT('Ctrl Pts',(1.57651739515791,-3.00641903721444,53.26870476174));
#11381=CARTESIAN_POINT('Ctrl Pts',(1.92504928497801,-2.79893975976317,53.2902628690432));
#11382=CARTESIAN_POINT('Ctrl Pts',(2.10448949170084,-2.666642059985,53.3019240501951));
#11383=CARTESIAN_POINT('Ctrl Pts',(2.29579079117951,-2.49419074111917,53.3164999363096));
#11384=CARTESIAN_POINT('Ctrl Pts',(2.32155267502854,-2.4702299049804,53.3185138071492));
#11385=CARTESIAN_POINT('Ctrl Pts',(2.3620902765292,-2.43133208245837,53.3217741676592));
#11386=CARTESIAN_POINT('Ctrl Pts',(2.37710875644105,-2.41665059102843,53.3230027877577));
#11387=CARTESIAN_POINT('Ctrl Pts',(2.40668067456327,-2.38719984390909,53.3254658686477));
#11388=CARTESIAN_POINT('Ctrl Pts',(2.42123690728599,-2.37243477168986,53.3267000386163));
#11389=CARTESIAN_POINT('Ctrl Pts',(2.45922896035533,-2.33318382467216,53.3299768281626));
#11390=CARTESIAN_POINT('Ctrl Pts',(2.48243408742767,-2.30847886103826,53.3320351572997));
#11391=CARTESIAN_POINT('Ctrl Pts',(2.53372104529874,-2.2522094334881,53.3367059232514));
#11392=CARTESIAN_POINT('Ctrl Pts',(2.56159092738067,-2.2204597041786,53.3393294895995));
#11393=CARTESIAN_POINT('Ctrl Pts',(2.6506195517551,-2.11512989733755,53.3479729135561));
#11394=CARTESIAN_POINT('Ctrl Pts',(2.70925611841536,-2.03948230091072,53.3540862939258));
#11395=CARTESIAN_POINT('Ctrl Pts',(2.9156333825492,-1.74860052015084,53.3769999900173));
#11396=CARTESIAN_POINT('Ctrl Pts',(3.04159073019534,-1.51897523051815,53.3938516392515));
#11397=CARTESIAN_POINT('Ctrl Pts',(3.16298865604935,-1.22051071625204,53.413551782908));
#11398=CARTESIAN_POINT('Ctrl Pts',(3.18449008889452,-1.16325716686628,53.4172430416015));
#11399=CARTESIAN_POINT('Ctrl Pts',(3.21661719117919,-1.07012850821992,53.4231098999423));
#11400=CARTESIAN_POINT('Ctrl Pts',(3.22821787227389,-1.03460655006405,53.4253162380643));
#11401=CARTESIAN_POINT('Ctrl Pts',(3.24954597043363,-0.965443800308088,
53.4295535471454));
#11402=CARTESIAN_POINT('Ctrl Pts',(3.2593440758806,-0.931829959601022,53.4315865444558));
#11403=CARTESIAN_POINT('Ctrl Pts',(3.28140793265502,-0.851526186780927,
53.4363840131463));
#11404=CARTESIAN_POINT('Ctrl Pts',(3.29320075221251,-0.804713613622579,
53.4391333699168));
#11405=CARTESIAN_POINT('Ctrl Pts',(3.33429680626021,-0.625503486553928,
53.4494971391396));
#11406=CARTESIAN_POINT('Ctrl Pts',(3.35664823094535,-0.491637535292613,
53.4568997854144));
#11407=CARTESIAN_POINT('Ctrl Pts',(3.38594981301633,-0.214792454780028,
53.4718536075304));
#11408=CARTESIAN_POINT('Ctrl Pts',(3.39199186502904,-0.0719958942982847,
53.4793767791466));
#11409=CARTESIAN_POINT('Ctrl Pts',(3.38613296549362,0.20862635739138,53.4943414166087));
#11410=CARTESIAN_POINT('Ctrl Pts',(3.37484426580657,0.346180651397624,53.5017648360333));
#11411=CARTESIAN_POINT('Ctrl Pts',(3.34962880555744,0.521468955304257,53.5117400661906));
#11412=CARTESIAN_POINT('Ctrl Pts',(3.34337196287359,0.560184479288933,53.5139762506026));
#11413=CARTESIAN_POINT('Ctrl Pts',(3.33258790360751,0.62027393360538,53.517510387474));
#11414=CARTESIAN_POINT('Ctrl Pts',(3.32852315444243,0.64172848019871,53.5187848983954));
#11415=CARTESIAN_POINT('Ctrl Pts',(3.32030952213742,0.682902459952344,53.5212578106338));
#11416=CARTESIAN_POINT('Ctrl Pts',(3.31619160074067,0.702626703030152,53.5224546077159));
#11417=CARTESIAN_POINT('Ctrl Pts',(3.30531120535703,0.752514769831181,53.5255107260587));
#11418=CARTESIAN_POINT('Ctrl Pts',(3.29831156883901,0.782624617058191,53.5273822316073));
#11419=CARTESIAN_POINT('Ctrl Pts',(3.26464852653738,0.918949018263562,53.5359657875073));
#11420=CARTESIAN_POINT('Ctrl Pts',(3.23326114171657,1.02392174267986,53.5428789673085));
#11421=CARTESIAN_POINT('Ctrl Pts',(3.14555808507566,1.27266038465735,53.5597311700279));
#11422=CARTESIAN_POINT('Ctrl Pts',(3.08439317204763,1.41446811678783,53.5697265280043));
#11423=CARTESIAN_POINT('Ctrl Pts',(2.93961036044075,1.69568657637012,53.5899274326136));
#11424=CARTESIAN_POINT('Ctrl Pts',(2.85519664450187,1.83426429852382,53.6000900035199));
#11425=CARTESIAN_POINT('Ctrl Pts',(2.73165818452038,2.00774479450128,53.6129980068788));
#11426=CARTESIAN_POINT('Ctrl Pts',(2.70120316788931,2.04853544265164,53.6160490993045));
#11427=CARTESIAN_POINT('Ctrl Pts',(2.64821995555896,2.11626257858412,53.6211450430547));
#11428=CARTESIAN_POINT('Ctrl Pts',(2.62617174886801,2.14356206270229,53.6232077521041));
#11429=CARTESIAN_POINT('Ctrl Pts',(2.58033553382868,2.19854619657751,53.6273821356807));
#11430=CARTESIAN_POINT('Ctrl Pts',(2.55651629028332,2.22619887976334,53.6294921853701));
#11431=CARTESIAN_POINT('Ctrl Pts',(2.4946069398356,2.29576748384065,53.6348322910165));
#11432=CARTESIAN_POINT('Ctrl Pts',(2.45590381723638,2.3371241036674,53.6380369919694));
#11433=CARTESIAN_POINT('Ctrl Pts',(2.30411993784524,2.49137788343762,53.6501392043006));
#11434=CARTESIAN_POINT('Ctrl Pts',(2.18414084450859,2.59720382163998,53.6587487917959));
#11435=CARTESIAN_POINT('Ctrl Pts',(1.86536944513923,2.84060146606205,53.6801182829856));
#11436=CARTESIAN_POINT('Ctrl Pts',(1.65853954576827,2.9661152993283,53.6926755684377));
#11437=CARTESIAN_POINT('Ctrl Pts',(1.40620340821925,3.08454290767146,53.7084066274108));
#11438=CARTESIAN_POINT('Ctrl Pts',(1.37197524368227,3.09991881551319,53.7105495486316));
#11439=CARTESIAN_POINT('Ctrl Pts',(1.31775493481248,3.12320168593756,53.7139688610426));
#11440=CARTESIAN_POINT('Ctrl Pts',(1.29792984466635,3.13149244033557,53.7152242227484));
#11441=CARTESIAN_POINT('Ctrl Pts',(1.25917405728812,3.14726867674767,53.7176907248316));
#11442=CARTESIAN_POINT('Ctrl Pts',(1.24025238214931,3.1547731118327,53.7189007849583));
#11443=CARTESIAN_POINT('Ctrl Pts',(1.19140707186828,3.17363809059535,53.7220374696585));
#11444=CARTESIAN_POINT('Ctrl Pts',(1.16138842798264,3.18474587665938,53.7239775563707));
#11445=CARTESIAN_POINT('Ctrl Pts',(1.01079097960334,3.23805912851354,53.7337565137636));
#11446=CARTESIAN_POINT('Ctrl Pts',(0.888059672820282,3.27384632969777,53.7418683450188));
#11447=CARTESIAN_POINT('Ctrl Pts',(0.483561204869113,3.36737225583087,53.7684938398514));
#11448=CARTESIAN_POINT('Ctrl Pts',(0.196352309392905,3.39625175660232,53.787107687746));
#11449=CARTESIAN_POINT('Ctrl Pts',(-0.145920713740234,3.3870521458296,53.8079352164141));
#11450=CARTESIAN_POINT('Ctrl Pts',(-0.200722974356862,3.38424672584363,
53.8112337773401));
#11451=CARTESIAN_POINT('Ctrl Pts',(-0.291491544816678,3.37738733451354,
53.8166396593038));
#11452=CARTESIAN_POINT('Ctrl Pts',(-0.327502701276744,3.37408575150571,
53.8187693411268));
#11453=CARTESIAN_POINT('Ctrl Pts',(-0.399009248509365,3.36637423260744,
53.8229703357184));
#11454=CARTESIAN_POINT('Ctrl Pts',(-0.434501321906444,3.36197748305969,
53.82504176409));
#11455=CARTESIAN_POINT('Ctrl Pts',(-0.522113281326584,3.34971349433156,
53.8301246383504));
#11456=CARTESIAN_POINT('Ctrl Pts',(-0.574132686689068,3.34119063346354,
53.8331157161812));
#11457=CARTESIAN_POINT('Ctrl Pts',(-0.836960791282227,3.29180891568344,
53.8481235844396));
#11458=CARTESIAN_POINT('Ctrl Pts',(-1.04374769815246,3.23219913396659,53.8595485025921));
#11459=CARTESIAN_POINT('Ctrl Pts',(-1.42404672304241,3.08223187924565,53.8812546604134));
#11460=CARTESIAN_POINT('Ctrl Pts',(-1.59810771360037,2.99567998575996,53.8915139594138));
#11461=CARTESIAN_POINT('Ctrl Pts',(-1.79606439957106,2.87506280281147,53.9045920959586));
#11462=CARTESIAN_POINT('Ctrl Pts',(-1.8280066086371,2.85485989831206,53.9067499878424));
#11463=CARTESIAN_POINT('Ctrl Pts',(-1.87761648768503,2.8223085543644,53.9101877376386));
#11464=CARTESIAN_POINT('Ctrl Pts',(-1.89551640211223,2.81031791192903,53.9114461861937));
#11465=CARTESIAN_POINT('Ctrl Pts',(-1.93007366748487,2.7866886422809,53.9139135270737));
#11466=CARTESIAN_POINT('Ctrl Pts',(-1.94674280044033,2.77506943107268,53.9151212526667));
#11467=CARTESIAN_POINT('Ctrl Pts',(-1.98924410726643,2.7448725595004,53.9182439921702));
#11468=CARTESIAN_POINT('Ctrl Pts',(-2.01492065489445,2.7260799844922,53.9201722465617));
#11469=CARTESIAN_POINT('Ctrl Pts',(-2.13944206965429,2.63222290170996,53.9297149221311));
#11470=CARTESIAN_POINT('Ctrl Pts',(-2.23437044782411,2.55213503843991,53.9375871708117));
#11471=CARTESIAN_POINT('Ctrl Pts',(-2.53296903998981,2.27076533082989,53.9638827342647));
#11472=CARTESIAN_POINT('Ctrl Pts',(-2.71559968869029,2.04887199185127,53.9824370793653));
#11473=CARTESIAN_POINT('Ctrl Pts',(-2.89879238953796,1.7580408283262,54.003390690979));
#11474=CARTESIAN_POINT('Ctrl Pts',(-2.92816929547138,1.70866323326224,54.0068504527771));
#11475=CARTESIAN_POINT('Ctrl Pts',(-2.9742104486785,1.62659781187271,54.0124455118186));
#11476=CARTESIAN_POINT('Ctrl Pts',(-2.99162343331729,1.59434551587221,54.014606501733));
#11477=CARTESIAN_POINT('Ctrl Pts',(-3.0248168476347,1.53040538362912,54.0188188610676));
#11478=CARTESIAN_POINT('Ctrl Pts',(-3.04063072914205,1.49874030639207,54.0208711817759));
#11479=CARTESIAN_POINT('Ctrl Pts',(-3.07784726944555,1.42120469938868,54.0258184597566));
#11480=CARTESIAN_POINT('Ctrl Pts',(-3.09872438510022,1.37509060441782,54.0286955728289));
#11481=CARTESIAN_POINT('Ctrl Pts',(-3.18385868700254,1.17524741255232,54.0409104488996));
#11482=CARTESIAN_POINT('Ctrl Pts',(-3.23776973060225,1.01735812739505,54.0499128157608));
#11483=CARTESIAN_POINT('Ctrl Pts',(-3.34130616867213,0.62070800530699,54.0717742388552));
#11484=CARTESIAN_POINT('Ctrl Pts',(-3.37722260790877,0.379390304076916,
54.0844189787722));
#11485=CARTESIAN_POINT('Ctrl Pts',(-3.38700661852469,0.136349655555036,
54.0981108245895));
#11486=CARTESIAN_POINT('',(-3.38974892034748,-0.00270545801625161,52.5160178032496));
#11487=CARTESIAN_POINT('Ctrl Pts',(-3.38700661857411,0.136349654327203,
53.7581562375148));
#11488=CARTESIAN_POINT('Ctrl Pts',(-3.38089832230461,0.288083371549333,
53.7492154215617));
#11489=CARTESIAN_POINT('Ctrl Pts',(-3.3646031929328,0.439076737459294,53.7402746056086));
#11490=CARTESIAN_POINT('Ctrl Pts',(-3.33832120308359,0.588231763459373,
53.7313337896555));
#11491=CARTESIAN_POINT('Ctrl Pts',(-3.33584314013142,0.6022952170328,53.7304907825277));
#11492=CARTESIAN_POINT('Ctrl Pts',(-3.33327632582759,0.616342345712101,
53.7296477753999));
#11493=CARTESIAN_POINT('Ctrl Pts',(-3.33062094849041,0.630372239218109,
53.7288047682721));
#11494=CARTESIAN_POINT('Ctrl Pts',(-3.31139138984876,0.731973113840281,
53.7226999278141));
#11495=CARTESIAN_POINT('Ctrl Pts',(-3.28747651147585,0.832862740521183,
53.7165950873561));
#11496=CARTESIAN_POINT('Ctrl Pts',(-3.25894239268673,0.932576829890859,
53.7104902468981));
#11497=CARTESIAN_POINT('Ctrl Pts',(-3.23044548929775,1.03216086794328,53.7043933686303));
#11498=CARTESIAN_POINT('Ctrl Pts',(-3.19734143965255,1.13057200949136,53.6982964903625));
#11499=CARTESIAN_POINT('Ctrl Pts',(-3.15974750580198,1.22735518986076,53.6921996120947));
#11500=CARTESIAN_POINT('Ctrl Pts',(-3.12219188159578,1.32403974449882,53.6861089467771));
#11501=CARTESIAN_POINT('Ctrl Pts',(-3.08015562554104,1.41909924075953,53.6800182814594));
#11502=CARTESIAN_POINT('Ctrl Pts',(-3.03380582163393,1.51209368066932,53.6739276161418));
#11503=CARTESIAN_POINT('Ctrl Pts',(-2.98748850473577,1.60502293991064,53.6678412198282));
#11504=CARTESIAN_POINT('Ctrl Pts',(-2.93686384247436,1.69588963992659,53.6617548235146));
#11505=CARTESIAN_POINT('Ctrl Pts',(-2.88214672577944,1.78427445018384,53.655668427201));
#11506=CARTESIAN_POINT('Ctrl Pts',(-2.82744947496616,1.87262717099111,53.6495842406461));
#11507=CARTESIAN_POINT('Ctrl Pts',(-2.76866294749466,1.95849943013418,53.6435000540913));
#11508=CARTESIAN_POINT('Ctrl Pts',(-2.70604720913747,2.04149787274425,53.6374158675365));
#11509=CARTESIAN_POINT('Ctrl Pts',(-2.64343803376025,2.12448761599007,53.631332318687));
#11510=CARTESIAN_POINT('Ctrl Pts',(-2.57700070295938,2.20460380069758,53.6252487698376));
#11511=CARTESIAN_POINT('Ctrl Pts',(-2.50703716190101,2.2814841071871,53.6191652209882));
#11512=CARTESIAN_POINT('Ctrl Pts',(-2.43706288608055,2.35837620970335,53.6130807387176));
#11513=CARTESIAN_POINT('Ctrl Pts',(-2.36356161262207,2.43203113159341,53.606996256447));
#11514=CARTESIAN_POINT('Ctrl Pts',(-2.2868732924771,2.50212222056696,53.6009117741764));
#11515=CARTESIAN_POINT('Ctrl Pts',(-2.21010590771101,2.57228557250551,53.5948210188868));
#11516=CARTESIAN_POINT('Ctrl Pts',(-2.1301452304708,2.63887746531716,53.5887302635973));
#11517=CARTESIAN_POINT('Ctrl Pts',(-2.04736552501942,2.70161053252721,53.5826395083078));
#11518=CARTESIAN_POINT('Ctrl Pts',(-1.96454102472262,2.76437754668154,53.5765454571084));
#11519=CARTESIAN_POINT('Ctrl Pts',(-1.87889480957758,2.82328133367252,53.5704514059091));
#11520=CARTESIAN_POINT('Ctrl Pts',(-1.79082980884284,2.87807811885986,53.5643573547097));
#11521=CARTESIAN_POINT('Ctrl Pts',(-1.70262368180194,2.93296271722858,53.5582535376451));
#11522=CARTESIAN_POINT('Ctrl Pts',(-1.61199139918918,2.98372695783321,53.5521497205805));
#11523=CARTESIAN_POINT('Ctrl Pts',(-1.51936030942531,3.0301731489542,53.5460459035158));
#11524=CARTESIAN_POINT('Ctrl Pts',(-1.45109889423784,3.06440013196897,53.5415478975878));
#11525=CARTESIAN_POINT('Ctrl Pts',(-1.38175253004824,3.09628319019804,53.5370498916597));
#11526=CARTESIAN_POINT('Ctrl Pts',(-1.31149811501989,3.12576034858709,53.5325518857317));
#11527=CARTESIAN_POINT('Ctrl Pts',(-1.21614651747083,3.16576771527668,53.5264470444794));
#11528=CARTESIAN_POINT('Ctrl Pts',(-1.11880358129998,3.20147477068205,53.5203422032271));
#11529=CARTESIAN_POINT('Ctrl Pts',(-1.01989301568441,3.2326805129889,53.5142373619747));
#11530=CARTESIAN_POINT('Ctrl Pts',(-0.921111453306506,3.26384555548005,
53.508140482908));
#11531=CARTESIAN_POINT('Ctrl Pts',(-0.82076673036726,3.29052082920096,53.5020436038414));
#11532=CARTESIAN_POINT('Ctrl Pts',(-0.719303095967168,3.31255311182056,
53.4959467247747));
#11533=CARTESIAN_POINT('Ctrl Pts',(-0.617942856788223,3.33456294272386,
53.4898560586548));
#11534=CARTESIAN_POINT('Ctrl Pts',(-0.515466388872144,3.35193910107061,
53.4837653925349));
#11535=CARTESIAN_POINT('Ctrl Pts',(-0.412332857848781,3.36457823164186,
53.477674726415));
#11536=CARTESIAN_POINT('Ctrl Pts',(-0.309271614037571,3.37720850333371,
53.4715883292973));
#11537=CARTESIAN_POINT('Ctrl Pts',(-0.205554645802275,3.385108298159,53.4655019321796));
#11538=CARTESIAN_POINT('Ctrl Pts',(-0.101650252254103,3.38822553687276,
53.4594155350619));
#11539=CARTESIAN_POINT('Ctrl Pts',(0.00221641724162593,3.39134164382613,
53.4533313477022));
#11540=CARTESIAN_POINT('Ctrl Pts',(0.10626995023665,3.3896786329916,53.4472471603425));
#11541=CARTESIAN_POINT('Ctrl Pts',(0.210038793604787,3.38323643390187,53.4411629729828));
#11542=CARTESIAN_POINT('Ctrl Pts',(0.313796760586779,3.37679491004223,53.4350794233287));
#11543=CARTESIAN_POINT('Ctrl Pts',(0.417269670903458,3.36557522059296,53.4289958736746));
#11544=CARTESIAN_POINT('Ctrl Pts',(0.519988755373871,3.34962934617918,53.4229123240205));
#11545=CARTESIAN_POINT('Ctrl Pts',(0.622723600387313,3.33368102513494,53.4168278409464));
#11546=CARTESIAN_POINT('Ctrl Pts',(0.724703967579495,3.31300514393209,53.4107433578723));
#11547=CARTESIAN_POINT('Ctrl Pts',(0.825469872181442,3.28770505864208,53.4046588747982));
#11548=CARTESIAN_POINT('Ctrl Pts',(0.926339664943076,3.26237888933774,53.3985681187119));
#11549=CARTESIAN_POINT('Ctrl Pts',(1.02599207958538,3.23241909955356,53.3924773626257));
#11550=CARTESIAN_POINT('Ctrl Pts',(1.12398097072417,3.1979793370111,53.3863866065394));
#11551=CARTESIAN_POINT('Ctrl Pts',(1.22202288685473,3.16352093798746,53.3802925545459));
#11552=CARTESIAN_POINT('Ctrl Pts',(1.3183990902397,3.12457789727113,53.3741985025524));
#11553=CARTESIAN_POINT('Ctrl Pts',(1.41268398227067,3.08135181839657,53.3681044505589));
#11554=CARTESIAN_POINT('Ctrl Pts',(1.50711996792513,3.03805646877518,53.3620006327124));
#11555=CARTESIAN_POINT('Ctrl Pts',(1.59945756773846,2.99046456621031,53.3558968148659));
#11556=CARTESIAN_POINT('Ctrl Pts',(1.68929614980463,2.93882350282477,53.3497929970194));
#11557=CARTESIAN_POINT('Ctrl Pts',(1.75549959287608,2.90076840309629,53.3452949990765));
#11558=CARTESIAN_POINT('Ctrl Pts',(1.8203464993356,2.86051538189802,53.3407970011337));
#11559=CARTESIAN_POINT('Ctrl Pts',(1.8836875944295,2.81817779941089,53.3362990031909));
#11560=CARTESIAN_POINT('Ctrl Pts',(1.96965632723492,2.76071576293887,53.3301941642592));
#11561=CARTESIAN_POINT('Ctrl Pts',(2.05313672094171,2.69922058348168,53.3240893253275));
#11562=CARTESIAN_POINT('Ctrl Pts',(2.13372739052763,2.6339347914123,53.3179844863958));
#11563=CARTESIAN_POINT('Ctrl Pts',(2.21421295037924,2.56873414781351,53.3118876096513));
#11564=CARTESIAN_POINT('Ctrl Pts',(2.2918159498874,2.49975298727891,53.3057907329068));
#11565=CARTESIAN_POINT('Ctrl Pts',(2.36616352571386,2.42727732904202,53.2996938561623));
#11566=CARTESIAN_POINT('Ctrl Pts',(2.44043533858205,2.35487552620941,53.2936031923631));
#11567=CARTESIAN_POINT('Ctrl Pts',(2.51145802035402,2.27898660371923,53.2875125285638));
#11568=CARTESIAN_POINT('Ctrl Pts',(2.57889207269775,2.19993653087463,53.2814218647646));
#11569=CARTESIAN_POINT('Ctrl Pts',(2.64627886002463,2.12094186479998,53.2753354699558));
#11570=CARTESIAN_POINT('Ctrl Pts',(2.71008174346828,2.03879077863847,53.2692490751471));
#11571=CARTESIAN_POINT('Ctrl Pts',(2.7699989549438,1.95384514537623,53.2631626803383));
#11572=CARTESIAN_POINT('Ctrl Pts',(2.82989441264589,1.86893035280257,53.2570784952795));
#11573=CARTESIAN_POINT('Ctrl Pts',(2.8859067563119,1.78122337841738,53.2509943102206));
#11574=CARTESIAN_POINT('Ctrl Pts',(2.93777580264318,1.69111749914198,53.2449101251618));
#11575=CARTESIAN_POINT('Ctrl Pts',(2.98963941248285,1.60102106403206,53.2388265777978));
#11576=CARTESIAN_POINT('Ctrl Pts',(3.03736037549326,1.50852659430234,53.2327430304337));
#11577=CARTESIAN_POINT('Ctrl Pts',(3.08072345920221,1.41405375796721,53.2266594830697));
#11578=CARTESIAN_POINT('Ctrl Pts',(3.12409319635748,1.31956642612366,53.2205750022722));
#11579=CARTESIAN_POINT('Ctrl Pts',(3.16310354751013,1.22310051286622,53.2144905214746));
#11580=CARTESIAN_POINT('Ctrl Pts',(3.19758697752962,1.12509669968097,53.208406040677));
#11581=CARTESIAN_POINT('Ctrl Pts',(3.23210595966656,1.02699184541382,53.2023152868325));
#11582=CARTESIAN_POINT('Ctrl Pts',(3.26208855823222,0.927346328604415,53.196224532988));
#11583=CARTESIAN_POINT('Ctrl Pts',(3.28741681995202,0.826617030066845,53.1901337791435));
#11584=CARTESIAN_POINT('Ctrl Pts',(3.31275878769398,0.725833223327642,53.1840397293757));
#11585=CARTESIAN_POINT('Ctrl Pts',(3.33344131661272,0.623964885329891,53.1779456796079));
#11586=CARTESIAN_POINT('Ctrl Pts',(3.34939778702454,0.521478213135649,53.1718516298401));
#11587=CARTESIAN_POINT('Ctrl Pts',(3.36537982816956,0.41882730290603,53.1657478141707));
#11588=CARTESIAN_POINT('Ctrl Pts',(3.37662063571285,0.31555650399105,53.1596439985013));
#11589=CARTESIAN_POINT('Ctrl Pts',(3.3831055540886,0.21213644758713,53.1535401828318));
#11590=CARTESIAN_POINT('Ctrl Pts',(3.38788441682756,0.13592419241689,53.1490421621047));
#11591=CARTESIAN_POINT('Ctrl Pts',(3.39008168558463,0.0596309572089956,
53.1445441413775));
#11592=CARTESIAN_POINT('Ctrl Pts',(3.38970956783697,-0.0165562137738431,
53.1400461206503));
#11593=CARTESIAN_POINT('Ctrl Pts',(3.38920451911107,-0.119959595837954,
53.1339412797724));
#11594=CARTESIAN_POINT('Ctrl Pts',(3.38396282606339,-0.22351230565078,53.1278364388946));
#11595=CARTESIAN_POINT('Ctrl Pts',(3.37396536250715,-0.326745765239541,
53.1217315980167));
#11596=CARTESIAN_POINT('Ctrl Pts',(3.36398093808233,-0.429844583212729,
53.1156347193406));
#11597=CARTESIAN_POINT('Ctrl Pts',(3.34925311562263,-0.532624557058128,
53.1095378406646));
#11598=CARTESIAN_POINT('Ctrl Pts',(3.32981477593396,-0.634616908435232,
53.1034409619885));
#11599=CARTESIAN_POINT('Ctrl Pts',(3.31039624468753,-0.736505325544588,
53.0973502962746));
#11600=CARTESIAN_POINT('Ctrl Pts',(3.28627682136983,-0.837607298772716,
53.0912596305607));
#11601=CARTESIAN_POINT('Ctrl Pts',(3.25754111386167,-0.937459841273676,
53.0851689648468));
#11602=CARTESIAN_POINT('Ctrl Pts',(3.22882554756865,-1.0372423958845,53.0790825681564));
#11603=CARTESIAN_POINT('Ctrl Pts',(3.1955002493585,-1.13577685192026,53.0729961714659));
#11604=CARTESIAN_POINT('Ctrl Pts',(3.15770058716458,-1.23261188714066,53.0669097747754));
#11605=CARTESIAN_POINT('Ctrl Pts',(3.11991464878697,-1.32941176473906,53.0608255878558));
#11606=CARTESIAN_POINT('Ctrl Pts',(3.07765773035409,-1.42451305029741,53.0547414009361));
#11607=CARTESIAN_POINT('Ctrl Pts',(3.03111433296921,-1.51748178340586,53.0486572140165));
#11608=CARTESIAN_POINT('Ctrl Pts',(2.98457581405908,-1.61044077193951,53.0425736648146));
#11609=CARTESIAN_POINT('Ctrl Pts',(2.93375190095082,-1.70126727054694,53.0364901156127));
#11610=CARTESIAN_POINT('Ctrl Pts',(2.87887390359773,-1.78955025346704,53.0304065664109));
#11611=CARTESIAN_POINT('Ctrl Pts',(2.8239874862283,-1.87784678178231,53.0243220838006));
#11612=CARTESIAN_POINT('Ctrl Pts',(2.76504597433088,-1.96359865620777,53.0182376011903));
#11613=CARTESIAN_POINT('Ctrl Pts',(2.70232451638145,-2.04642304293706,53.01215311858));
#11614=CARTESIAN_POINT('Ctrl Pts',(2.63953839368367,-2.12933282018978,53.0060623629725));
#11615=CARTESIAN_POINT('Ctrl Pts',(2.57296480093383,-2.20930874125264,52.9999716073649));
#11616=CARTESIAN_POINT('Ctrl Pts',(2.50291974928054,-2.28600039176756,52.9938808517573));
#11617=CARTESIAN_POINT('Ctrl Pts',(2.43283679406054,-2.36273354253157,52.9877868002515));
#11618=CARTESIAN_POINT('Ctrl Pts',(2.35927894036816,-2.43617858074976,52.9816927487457));
#11619=CARTESIAN_POINT('Ctrl Pts',(2.28259828726525,-2.50602276954416,52.9755986972399));
#11620=CARTESIAN_POINT('Ctrl Pts',(2.20579475183068,-2.57597888509483,52.9694948798906));
#11621=CARTESIAN_POINT('Ctrl Pts',(2.1258587493692,-2.6423223514547,52.9633910625413));
#11622=CARTESIAN_POINT('Ctrl Pts',(2.04317474257019,-2.70478132828206,52.9572872451919));
#11623=CARTESIAN_POINT('Ctrl Pts',(1.98224355205528,-2.75080836499406,52.9527892428312));
#11624=CARTESIAN_POINT('Ctrl Pts',(1.91982073489687,-2.79472681761542,52.9482912404704));
#11625=CARTESIAN_POINT('Ctrl Pts',(1.85606903414094,-2.83644368937638,52.9437932381097));
#11626=CARTESIAN_POINT('Ctrl Pts',(1.76954300026846,-2.89306328408904,52.9376883922779));
#11627=CARTESIAN_POINT('Ctrl Pts',(1.68027951834246,-2.94581447430127,52.9315835464462));
#11628=CARTESIAN_POINT('Ctrl Pts',(1.58865887313047,-2.99442282373813,52.9254787006145));
#11629=CARTESIAN_POINT('Ctrl Pts',(1.49715772291929,-3.04296777638552,52.9193818169462));
#11630=CARTESIAN_POINT('Ctrl Pts',(1.40330589574736,-3.08738043194736,52.913284933278));
#11631=CARTESIAN_POINT('Ctrl Pts',(1.30751253226124,-3.12742962198669,52.9071880496098));
#11632=CARTESIAN_POINT('Ctrl Pts',(1.21181678545712,-3.16743800054486,52.9010973788725));
#11633=CARTESIAN_POINT('Ctrl Pts',(1.1141838288362,-3.20309159190741,52.8950067081353));
#11634=CARTESIAN_POINT('Ctrl Pts',(1.0150465067861,-3.23420556730109,52.888916037398));
#11635=CARTESIAN_POINT('Ctrl Pts',(0.915978670843065,-3.26529773467149,
52.8828296356584));
#11636=CARTESIAN_POINT('Ctrl Pts',(0.81540897278163,-3.29185648606345,52.8767432339189));
#11637=CARTESIAN_POINT('Ctrl Pts',(0.713788528613445,-3.31374576558309,
52.8706568321793));
#11638=CARTESIAN_POINT('Ctrl Pts',(0.612204979229959,-3.33562709788047,
52.8645726401967));
#11639=CARTESIAN_POINT('Ctrl Pts',(0.50957185915237,-3.35284223795687,52.858488448214));
#11640=CARTESIAN_POINT('Ctrl Pts',(0.406352906602684,-3.3653056886107,52.8524042562314));
#11641=CARTESIAN_POINT('Ctrl Pts',(0.30314477287223,-3.37776783291704,52.8463207019589));
#11642=CARTESIAN_POINT('Ctrl Pts',(0.199351352903832,-3.38547922705865,
52.8402371476864));
#11643=CARTESIAN_POINT('Ctrl Pts',(0.0954430767543992,-3.38840606799121,
52.834153593414));
#11644=CARTESIAN_POINT('Ctrl Pts',(-0.00848114221444304,-3.39133335799384,
52.8280691057316));
#11645=CARTESIAN_POINT('Ctrl Pts',(-0.112519825311717,-3.38947462424989,
52.8219846180493));
#11646=CARTESIAN_POINT('Ctrl Pts',(-0.216201874215394,-3.38284818046654,
52.815900130367));
#11647=CARTESIAN_POINT('Ctrl Pts',(-0.319990816950072,-3.37621490497057,
52.8098093697164));
#11648=CARTESIAN_POINT('Ctrl Pts',(-0.423421964109565,-3.36480413073154,
52.8037186090659));
#11649=CARTESIAN_POINT('Ctrl Pts',(-0.52602871677517,-3.34868613811863,
52.7976278484153));
#11650=CARTESIAN_POINT('Ctrl Pts',(-0.628690992966425,-3.33255942358681,
52.7915337918754));
#11651=CARTESIAN_POINT('Ctrl Pts',(-0.730527567488587,-3.31172050241758,
52.7854397353355));
#11652=CARTESIAN_POINT('Ctrl Pts',(-0.831083360381304,-3.28629053958979,
52.7793456787956));
#11653=CARTESIAN_POINT('Ctrl Pts',(-0.93180029479501,-3.26081982502835,
52.7732418564778));
#11654=CARTESIAN_POINT('Ctrl Pts',(-1.0312319385576,-3.23074349611941,52.76713803416));
#11655=CARTESIAN_POINT('Ctrl Pts',(-1.12893947007988,-3.19623227181564,
52.7610342118422));
#11656=CARTESIAN_POINT('Ctrl Pts',(-1.20094087720445,-3.17080069379142,
52.7565362597511));
#11657=CARTESIAN_POINT('Ctrl Pts',(-1.2720063947445,-3.14296185816959,52.7520383076601));
#11658=CARTESIAN_POINT('Ctrl Pts',(-1.34196868650031,-3.11280020350691,
52.7475403555691));
#11659=CARTESIAN_POINT('Ctrl Pts',(-1.43692472241457,-3.07186342039838,
52.7414355283889));
#11660=CARTESIAN_POINT('Ctrl Pts',(-1.53016425998354,-3.02650945017575,
52.7353307012087));
#11661=CARTESIAN_POINT('Ctrl Pts',(-1.62124861941892,-2.97690409259893,
52.7292258740285));
#11662=CARTESIAN_POINT('Ctrl Pts',(-1.71221418254363,-2.92736343255642,
52.7231290090381));
#11663=CARTESIAN_POINT('Ctrl Pts',(-1.80102978379207,-2.87358261158481,
52.7170321440476));
#11664=CARTESIAN_POINT('Ctrl Pts',(-1.88727691443995,-2.81577536581348,
52.7109352790571));
#11665=CARTESIAN_POINT('Ctrl Pts',(-1.97343615605219,-2.75802702777677,
52.7048446269989));
#11666=CARTESIAN_POINT('Ctrl Pts',(-2.05703177887024,-2.69626066085924,
52.6987539749407));
#11667=CARTESIAN_POINT('Ctrl Pts',(-2.13767084953855,-2.63073533475588,
52.6926633228826));
#11668=CARTESIAN_POINT('Ctrl Pts',(-2.21825340047877,-2.56525593519387,
52.6865769397476));
#11669=CARTESIAN_POINT('Ctrl Pts',(-2.29588318959422,-2.4960230844489,52.6804905566126));
#11670=CARTESIAN_POINT('Ctrl Pts',(-2.37019788498121,-2.42333799717055,
52.6744041734776));
#11671=CARTESIAN_POINT('Ctrl Pts',(-2.44448559989363,-2.35067929872606,
52.6683200000469));
#11672=CARTESIAN_POINT('Ctrl Pts',(-2.51546030812431,-2.27457115324918,
52.6622358266163));
#11673=CARTESIAN_POINT('Ctrl Pts',(-2.5827948851974,-2.19535319333773,52.6561516531856));
#11674=CARTESIAN_POINT('Ctrl Pts',(-2.650122405451,-2.11614353565178,52.6500681173904));
#11675=CARTESIAN_POINT('Ctrl Pts',(-2.71381027655406,-2.03382503718923,
52.6439845815952));
#11676=CARTESIAN_POINT('Ctrl Pts',(-2.77357079996188,-1.94877142838734,
52.6379010458));
#11677=CARTESIAN_POINT('Ctrl Pts',(-2.83334049350506,-1.86370476827562,
52.6318165764981));
#11678=CARTESIAN_POINT('Ctrl Pts',(-2.88918139640564,-1.77590251354845,
52.6257321071963));
#11679=CARTESIAN_POINT('Ctrl Pts',(-2.94084891135973,-1.68576770139136,
52.6196476378944));
#11680=CARTESIAN_POINT('Ctrl Pts',(-2.992569696728,-1.59553995813859,52.6135568953627));
#11681=CARTESIAN_POINT('Ctrl Pts',(-3.04010828853447,-1.50297522617446,
52.6074661528309));
#11682=CARTESIAN_POINT('Ctrl Pts',(-3.08326591619373,-1.40850145634928,
52.6013754102991));
#11683=CARTESIAN_POINT('Ctrl Pts',(-3.12644689862605,-1.31397656199353,
52.5952813717588));
#11684=CARTESIAN_POINT('Ctrl Pts',(-3.16524203502955,-1.21754096830853,
52.5891873332185));
#11685=CARTESIAN_POINT('Ctrl Pts',(-3.19950135126218,-1.1196410879257,52.5830932946782));
#11686=CARTESIAN_POINT('Ctrl Pts',(-3.23381557061824,-1.0215843156429,52.5769894899841));
#11687=CARTESIAN_POINT('Ctrl Pts',(-3.26357932707888,-0.922058978611061,
52.5708856852901));
#11688=CARTESIAN_POINT('Ctrl Pts',(-3.28869294748947,-0.82152526414774,
52.564781880596));
#11689=CARTESIAN_POINT('Ctrl Pts',(-3.30720017078735,-0.7474379811468,52.5602837447401));
#11690=CARTESIAN_POINT('Ctrl Pts',(-3.3231830594563,-0.672803339565695,
52.5557856088842));
#11691=CARTESIAN_POINT('Ctrl Pts',(-3.33661973224267,-0.597807514931707,
52.5512874730284));
#11692=CARTESIAN_POINT('Ctrl Pts',(-3.36382438323819,-0.445966708228573,
52.5421802916573));
#11693=CARTESIAN_POINT('Ctrl Pts',(-3.38066933541319,-0.292218649893261,
52.5330731102862));
#11694=CARTESIAN_POINT('Ctrl Pts',(-3.38695150873708,-0.137711800378893,
52.5239659289151));
#11695=CARTESIAN_POINT('Ctrl Pts',(-3.38877905928926,-0.0927641264471587,
52.5213165536932));
#11696=CARTESIAN_POINT('Ctrl Pts',(-3.3897129670525,-0.0477524120291606,
52.5186671784714));
#11697=CARTESIAN_POINT('Ctrl Pts',(-3.38974892034748,-0.00270545801625161,
52.5160178032496));
#11698=CARTESIAN_POINT('Ctrl Pts',(-3.39152367512854,-0.00269060468911869,
52.5160168468642));
#11699=CARTESIAN_POINT('Ctrl Pts',(-3.39112041704622,0.0436611229947171,
52.5132921806742));
#11700=CARTESIAN_POINT('Ctrl Pts',(-3.38975319490166,0.090027953380886,
52.5105675144842));
#11701=CARTESIAN_POINT('Ctrl Pts',(-3.38743469189442,0.136371088936278,
52.5078428482942));
#11702=CARTESIAN_POINT('Origin',(0.,0.,0.));
#11703=CARTESIAN_POINT('',(-3.38700661857411,0.136349654327209,51.2580969930732));
#11704=CARTESIAN_POINT('',(-3.38700661379996,0.136349772919874,51.6005689639805));
#11705=CARTESIAN_POINT('',(-3.38700661857411,0.136349654327212,0.));
#11706=CARTESIAN_POINT('',(-3.38974867768107,0.00293645210927518,51.6091549103211));
#11707=CARTESIAN_POINT('Ctrl Pts',(-3.38700661379996,0.136349772919874,
51.6005689639805));
#11708=CARTESIAN_POINT('Ctrl Pts',(-3.38879548487887,0.0919131886429986,
51.6034319494006));
#11709=CARTESIAN_POINT('Ctrl Pts',(-3.38971017523789,0.0474336314538165,
51.6062961227749));
#11710=CARTESIAN_POINT('Ctrl Pts',(-3.38974872771026,0.00293691789115749,
51.6091549678441));
#11711=CARTESIAN_POINT('Ctrl Pts',(-3.3897487281089,0.00293645774800871,
51.6091549974076));
#11712=CARTESIAN_POINT('Ctrl Pts',(-3.38987105787604,-0.138276938860297,
51.6182277397316));
#11713=CARTESIAN_POINT('Ctrl Pts',(-3.38116912748961,-0.279373005641703,
51.627220309697));
#11714=CARTESIAN_POINT('Ctrl Pts',(-3.35498934500473,-0.489277272767235,
51.6403570728065));
#11715=CARTESIAN_POINT('Ctrl Pts',(-3.34412219774405,-0.558742803692446,
51.6446660030182));
#11716=CARTESIAN_POINT('Ctrl Pts',(-3.32233360665932,-0.674348489415988,
51.6517704980771));
#11717=CARTESIAN_POINT('Ctrl Pts',(-3.31259094933643,-0.720685797073671,
51.6546001506718));
#11718=CARTESIAN_POINT('Ctrl Pts',(-3.29399230171,-0.800771948080072,51.6594617774325));
#11719=CARTESIAN_POINT('Ctrl Pts',(-3.2855803465773,-0.834615430341658,
51.661507189113));
#11720=CARTESIAN_POINT('Ctrl Pts',(-3.26698882397763,-0.904771111174041,
51.6657304430639));
#11721=CARTESIAN_POINT('Ctrl Pts',(-3.25672250925341,-0.941055471628134,
51.6679052353609));
#11722=CARTESIAN_POINT('Ctrl Pts',(-3.22771751943565,-1.03740174388216,
51.6736594903687));
#11723=CARTESIAN_POINT('Ctrl Pts',(-3.20790823785293,-1.09712724215636,
51.6772048774853));
#11724=CARTESIAN_POINT('Ctrl Pts',(-3.09162758310946,-1.4175734352985,51.6961723481098));
#11725=CARTESIAN_POINT('Ctrl Pts',(-2.96503289569032,-1.66621028992737,
51.7105862441453));
#11726=CARTESIAN_POINT('Ctrl Pts',(-2.74119056567748,-1.99779507427186,
51.7320515705437));
#11727=CARTESIAN_POINT('Ctrl Pts',(-2.66746898058891,-2.0952123385526,51.7387002793221));
#11728=CARTESIAN_POINT('Ctrl Pts',(-2.56819260788787,-2.21264480834499,
51.7474422266867));
#11729=CARTESIAN_POINT('Ctrl Pts',(-2.54738534201585,-2.23656837253055,
51.7492639629333));
#11730=CARTESIAN_POINT('Ctrl Pts',(-2.51271320640104,-2.2753218130507,51.7522893685993));
#11731=CARTESIAN_POINT('Ctrl Pts',(-2.49904467132517,-2.2903258985071,51.7534795528178));
#11732=CARTESIAN_POINT('Ctrl Pts',(-2.47056773260371,-2.32102688021627,
51.7559561569881));
#11733=CARTESIAN_POINT('Ctrl Pts',(-2.45574283270985,-2.33670661075482,
51.7572436395464));
#11734=CARTESIAN_POINT('Ctrl Pts',(-2.41443092156084,-2.37957329127065,
51.7608237458737));
#11735=CARTESIAN_POINT('Ctrl Pts',(-2.38763612859452,-2.40645780837782,
51.7631372659178));
#11736=CARTESIAN_POINT('Ctrl Pts',(-2.18903673737211,-2.59913985968773,
51.7801861561247));
#11737=CARTESIAN_POINT('Ctrl Pts',(-2.00059975057804,-2.74681691735285,
51.7957827711509));
#11738=CARTESIAN_POINT('Ctrl Pts',(-1.66164816339618,-2.95893343004414,
51.8213726801498));
#11739=CARTESIAN_POINT('Ctrl Pts',(-1.51914391289128,-3.0345632536054,51.831519559208));
#11740=CARTESIAN_POINT('Ctrl Pts',(-1.31982432293415,-3.12277080624156,
51.8448001997358));
#11741=CARTESIAN_POINT('Ctrl Pts',(-1.26729142258515,-3.14445651569493,
51.8482210557487));
#11742=CARTESIAN_POINT('Ctrl Pts',(-1.18012874384436,-3.17789800519564,
51.8537704955256));
#11743=CARTESIAN_POINT('Ctrl Pts',(-1.14581154357527,-3.19043188999231,
51.8559239524696));
#11744=CARTESIAN_POINT('Ctrl Pts',(-1.0781699104516,-3.21390483573051,51.8601093696363));
#11745=CARTESIAN_POINT('Ctrl Pts',(-1.04486517558037,-3.22488628435555,
51.862142479027));
#11746=CARTESIAN_POINT('Ctrl Pts',(-0.962949469430438,-3.25049376513832,
51.8670789974797));
#11747=CARTESIAN_POINT('Ctrl Pts',(-0.914168151969811,-3.26454872292996,
51.8699640671037));
#11748=CARTESIAN_POINT('Ctrl Pts',(-0.712492115176322,-3.31778054074508,
51.8816915375638));
#11749=CARTESIAN_POINT('Ctrl Pts',(-0.557262906336512,-3.34735383324367,
51.8902385934743));
#11750=CARTESIAN_POINT('Ctrl Pts',(-0.243918895803178,-3.38463903569707,
51.9070900918788));
#11751=CARTESIAN_POINT('Ctrl Pts',(-0.0862073925304647,-3.39232132574715,
51.9153757928337));
#11752=CARTESIAN_POINT('Ctrl Pts',(0.181882681816868,-3.38666826602269,
51.9298176140896));
#11753=CARTESIAN_POINT('Ctrl Pts',(0.292114723578123,-3.37894481550556,
51.935862044089));
#11754=CARTESIAN_POINT('Ctrl Pts',(0.432523396443501,-3.36218504322535,
51.9439091654905));
#11755=CARTESIAN_POINT('Ctrl Pts',(0.46323098688419,-3.35809196749698,51.9456906663847));
#11756=CARTESIAN_POINT('Ctrl Pts',(0.513824118068741,-3.3506411856894,51.9486677754617));
#11757=CARTESIAN_POINT('Ctrl Pts',(0.533744310745238,-3.34752573918671,
51.9498507795762));
#11758=CARTESIAN_POINT('Ctrl Pts',(0.575157259635956,-3.34066985373146,
51.9523347141267));
#11759=CARTESIAN_POINT('Ctrl Pts',(0.596643535394793,-3.33689936618805,
51.9536370463206));
#11760=CARTESIAN_POINT('Ctrl Pts',(0.65654546626964,-3.3257905367248,51.9573030423094));
#11761=CARTESIAN_POINT('Ctrl Pts',(0.694871642469487,-3.31799453956417,
51.9596891766464));
#11762=CARTESIAN_POINT('Ctrl Pts',(0.959525996132115,-3.25937440210863,
51.9764093468088));
#11763=CARTESIAN_POINT('Ctrl Pts',(1.18024131676789,-3.18610021009077,51.9915450678248));
#11764=CARTESIAN_POINT('Ctrl Pts',(1.55387646790826,-3.01786223221083,52.0177892658091));
#11765=CARTESIAN_POINT('Ctrl Pts',(1.71003755733788,-2.93220237788336,52.0289828493556));
#11766=CARTESIAN_POINT('Ctrl Pts',(1.90158604219653,-2.80659878090064,52.042869699458));
#11767=CARTESIAN_POINT('Ctrl Pts',(1.94375952304615,-2.77755747623924,52.0459394768243));
#11768=CARTESIAN_POINT('Ctrl Pts',(2.0140289994769,-2.72678417667402,52.0510780116933));
#11769=CARTESIAN_POINT('Ctrl Pts',(2.04246979922072,-2.70554652845264,52.0531646428357));
#11770=CARTESIAN_POINT('Ctrl Pts',(2.09947172719957,-2.66157016984409,52.0573629060216));
#11771=CARTESIAN_POINT('Ctrl Pts',(2.12800960088497,-2.63880893397884,52.0594732872653));
#11772=CARTESIAN_POINT('Ctrl Pts',(2.19989804813751,-2.57954733420765,52.0648155652048));
#11773=CARTESIAN_POINT('Ctrl Pts',(2.24271194414063,-2.54241214585397,52.0680220632045));
#11774=CARTESIAN_POINT('Ctrl Pts',(2.49019708357747,-2.31663371880594,52.0867557271232));
#11775=CARTESIAN_POINT('Ctrl Pts',(2.67192516132004,-2.10444631676261,52.1012322733145));
#11776=CARTESIAN_POINT('Ctrl Pts',(2.87556365369532,-1.79713549656603,52.1209561951511));
#11777=CARTESIAN_POINT('Ctrl Pts',(2.92242166496743,-1.71988727619846,52.1258343055489));
#11778=CARTESIAN_POINT('Ctrl Pts',(2.99429611797371,-1.5899622129895,52.1340551747531));
#11779=CARTESIAN_POINT('Ctrl Pts',(3.02113878404768,-1.53834610481194,52.1373253574219));
#11780=CARTESIAN_POINT('Ctrl Pts',(3.05771914351488,-1.46335147061405,52.1421183023096));
#11781=CARTESIAN_POINT('Ctrl Pts',(3.06854492988605,-1.44051234551156,52.1435833770792));
#11782=CARTESIAN_POINT('Ctrl Pts',(3.08726264045479,-1.39985504342026,52.146204637741));
#11783=CARTESIAN_POINT('Ctrl Pts',(3.09525793954078,-1.38208646628821,52.1473548265244));
#11784=CARTESIAN_POINT('Ctrl Pts',(3.11321275499186,-1.34124673581127,52.1500092555031));
#11785=CARTESIAN_POINT('Ctrl Pts',(3.12306931595686,-1.31813293291421,52.15151903168));
#11786=CARTESIAN_POINT('Ctrl Pts',(3.15369329506298,-1.24404703755062,52.1563770912907));
#11787=CARTESIAN_POINT('Ctrl Pts',(3.17347576003551,-1.19267989577675,52.1597735038214));
#11788=CARTESIAN_POINT('Ctrl Pts',(3.26690727779489,-0.931268360590284,
52.1771214028011));
#11789=CARTESIAN_POINT('Ctrl Pts',(3.32099067256739,-0.714816893078074,
52.1916474391223));
#11790=CARTESIAN_POINT('Ctrl Pts',(3.37724086001234,-0.33345442658512,52.2162658669266));
#11791=CARTESIAN_POINT('Ctrl Pts',(3.38936579170606,-0.170759440167206,
52.2264812983484));
#11792=CARTESIAN_POINT('Ctrl Pts',(3.38985704326271,0.0425848775897024,
52.2394055452134));
#11793=CARTESIAN_POINT('Ctrl Pts',(3.38884945476204,0.0929732405482049,
52.2424250329519));
#11794=CARTESIAN_POINT('Ctrl Pts',(3.38522394881534,0.178644149332612,52.2475051475909));
#11795=CARTESIAN_POINT('Ctrl Pts',(3.3831766467966,0.213941188261571,52.2495826975655));
#11796=CARTESIAN_POINT('Ctrl Pts',(3.37787884403524,0.285809479566358,52.2537832812902));
#11797=CARTESIAN_POINT('Ctrl Pts',(3.3745856624859,0.322372923341972,52.2559047254914));
#11798=CARTESIAN_POINT('Ctrl Pts',(3.36458496562479,0.416303061115712,52.2613185614779));
#11799=CARTESIAN_POINT('Ctrl Pts',(3.35700403925316,0.473565887704233,52.264584111905));
#11800=CARTESIAN_POINT('Ctrl Pts',(3.3052905989075,0.79985990430415,52.283041720845));
#11801=CARTESIAN_POINT('Ctrl Pts',(3.23029727614805,1.06297081266451,52.2972392750651));
#11802=CARTESIAN_POINT('Ctrl Pts',(3.08872379539329,1.39955389326863,52.3167603660537));
#11803=CARTESIAN_POINT('Ctrl Pts',(3.04937543608565,1.48333187692974,52.3217521768385));
#11804=CARTESIAN_POINT('Ctrl Pts',(2.97936203090318,1.61780689506126,52.3301404461206));
#11805=CARTESIAN_POINT('Ctrl Pts',(2.95070752615989,1.66949738903029,52.3334605314602));
#11806=CARTESIAN_POINT('Ctrl Pts',(2.90781690297534,1.74231228803539,52.3383134502885));
#11807=CARTESIAN_POINT('Ctrl Pts',(2.89466975283893,1.76406864608762,52.3397865886549));
#11808=CARTESIAN_POINT('Ctrl Pts',(2.87101396405339,1.8022385065597,52.3424159466096));
#11809=CARTESIAN_POINT('Ctrl Pts',(2.86060648159784,1.81871254861502,52.3435659984875));
#11810=CARTESIAN_POINT('Ctrl Pts',(2.83652960922569,1.85610593422345,52.3462117221215));
#11811=CARTESIAN_POINT('Ctrl Pts',(2.82277048245854,1.87696461997163,52.3477127650335));
#11812=CARTESIAN_POINT('Ctrl Pts',(2.77721730143225,1.94438892006352,52.3526425717778));
#11813=CARTESIAN_POINT('Ctrl Pts',(2.74449314205261,1.99031174862924,52.3561227195155));
#11814=CARTESIAN_POINT('Ctrl Pts',(2.57743683899233,2.21278936472214,52.3735162069105));
#11815=CARTESIAN_POINT('Ctrl Pts',(2.42714402196589,2.37667578195511,52.3879932241919));
#11816=CARTESIAN_POINT('Ctrl Pts',(2.140731632253,2.63327709480896,52.41255038668));
#11817=CARTESIAN_POINT('Ctrl Pts',(2.01187126753199,2.73299574038936,52.4227522423883));
#11818=CARTESIAN_POINT('Ctrl Pts',(1.83437461242483,2.85096698845879,52.4356630076093));
#11819=CARTESIAN_POINT('Ctrl Pts',(1.7918005229941,2.87791491855263,52.4386817164428));
#11820=CARTESIAN_POINT('Ctrl Pts',(1.71835510809195,2.92214142648197,52.4437609514644));
#11821=CARTESIAN_POINT('Ctrl Pts',(1.6877861928792,2.93990351894607,52.4458383854721));
#11822=CARTESIAN_POINT('Ctrl Pts',(1.62491675438216,2.97512997878435,52.4500390839158));
#11823=CARTESIAN_POINT('Ctrl Pts',(1.5925991082126,2.99255427377152,52.4521607530354));
#11824=CARTESIAN_POINT('Ctrl Pts',(1.50871453160159,3.03603738002926,52.4575759155834));
#11825=CARTESIAN_POINT('Ctrl Pts',(1.45675205264521,3.06130960674944,52.4608425419491));
#11826=CARTESIAN_POINT('Ctrl Pts',(1.15614185747562,3.19812441646148,52.4792950249874));
#11827=CARTESIAN_POINT('Ctrl Pts',(0.895419301129158,3.28068494276031,52.4934874155788));
#11828=CARTESIAN_POINT('Ctrl Pts',(0.493959466364551,3.35632348972954,52.5153272777128));
#11829=CARTESIAN_POINT('Ctrl Pts',(0.358920374819451,3.37343629959095,52.5226924495569));
#11830=CARTESIAN_POINT('Ctrl Pts',(0.190916675886263,3.38452430683381,52.5322553231149));
#11831=CARTESIAN_POINT('Ctrl Pts',(0.158572621835733,3.38619381042795,52.5341147485072));
#11832=CARTESIAN_POINT('Ctrl Pts',(0.105795509761141,3.38816022922224,52.5371858608962));
#11833=CARTESIAN_POINT('Ctrl Pts',(0.0853740264588072,3.38873629529908,
52.5383832303929));
#11834=CARTESIAN_POINT('Ctrl Pts',(0.0435717885324079,3.38953738855444,
52.540854871851));
#11835=CARTESIAN_POINT('Ctrl Pts',(0.0221919479965969,3.38974477992475,
52.542129911089));
#11836=CARTESIAN_POINT('Ctrl Pts',(-0.0361875206390548,3.38975876814832,
52.5456387085442));
#11837=CARTESIAN_POINT('Ctrl Pts',(-0.0731833303047075,3.38916184372154,
52.5478920926298));
#11838=CARTESIAN_POINT('Ctrl Pts',(-0.316538787699377,3.38124908538498,
52.5628794440812));
#11839=CARTESIAN_POINT('Ctrl Pts',(-0.521859338970512,3.35569592859384,
52.5762760873013));
#11840=CARTESIAN_POINT('Ctrl Pts',(-0.920842547156187,3.26852116135418,
52.6025258227099));
#11841=CARTESIAN_POINT('Ctrl Pts',(-1.11389786101519,3.20787058003291,52.6153281811723));
#11842=CARTESIAN_POINT('Ctrl Pts',(-1.34984712358641,3.10985237075649,52.6308513326477));
#11843=CARTESIAN_POINT('Ctrl Pts',(-1.39877715367245,3.08815349085226,52.6340657641505));
#11844=CARTESIAN_POINT('Ctrl Pts',(-1.47964648362908,3.04997389471161,52.6393731063393));
#11845=CARTESIAN_POINT('Ctrl Pts',(-1.51187317492557,3.0341282313925,52.6414866958907));
#11846=CARTESIAN_POINT('Ctrl Pts',(-1.57589042752171,3.00137805996543,52.6456845056885));
#11847=CARTESIAN_POINT('Ctrl Pts',(-1.60767555491014,2.98447321182746,52.6477683678868));
#11848=CARTESIAN_POINT('Ctrl Pts',(-1.68645263251289,2.94095198307756,52.6529358224508));
#11849=CARTESIAN_POINT('Ctrl Pts',(-1.73308992255605,2.91371254872916,52.6559974383317));
#11850=CARTESIAN_POINT('Ctrl Pts',(-2.0274189979257,2.73223540059595,52.6753792958114));
#11851=CARTESIAN_POINT('Ctrl Pts',(-2.25495812588372,2.54768627066783,52.6905086998192));
#11852=CARTESIAN_POINT('Ctrl Pts',(-2.54257924458769,2.24531838466659,52.7128777053626));
#11853=CARTESIAN_POINT('Ctrl Pts',(-2.62397250391029,2.14963401706148,52.7197043680379));
#11854=CARTESIAN_POINT('Ctrl Pts',(-2.71914997230546,2.02426423880615,52.7286505082782));
#11855=CARTESIAN_POINT('Ctrl Pts',(-2.73807489114561,1.99859150779091,52.7304826618189));
#11856=CARTESIAN_POINT('Ctrl Pts',(-2.76846702437069,1.95612086719505,52.733520709445));
#11857=CARTESIAN_POINT('Ctrl Pts',(-2.78015081454608,1.93947929588414,52.7347128908033));
#11858=CARTESIAN_POINT('Ctrl Pts',(-2.80389203030473,1.90500859873086,52.7371880418936));
#11859=CARTESIAN_POINT('Ctrl Pts',(-2.81593055365271,1.88716807447398,52.738471990852));
#11860=CARTESIAN_POINT('Ctrl Pts',(-2.84857845315503,1.83777745739272,52.7420318516036));
#11861=CARTESIAN_POINT('Ctrl Pts',(-2.86883229941964,1.80599727907717,52.7443282963346));
#11862=CARTESIAN_POINT('Ctrl Pts',(-2.99142721624258,1.60636698104816,52.7587583953573));
#11863=CARTESIAN_POINT('Ctrl Pts',(-3.07952865630849,1.43022564660035,52.7714880063254));
#11864=CARTESIAN_POINT('Ctrl Pts',(-3.20427716363135,1.11503194436916,52.7932909347465));
#11865=CARTESIAN_POINT('Ctrl Pts',(-3.24829444849369,0.979426934267012,
52.8023896652377));
#11866=CARTESIAN_POINT('Ctrl Pts',(-3.30688705398011,0.750775642305356,
52.8171100024576));
#11867=CARTESIAN_POINT('Ctrl Pts',(-3.32635768508744,0.659176045620381,
52.82285006368));
#11868=CARTESIAN_POINT('Ctrl Pts',(-3.34922340952981,0.524372559918057,
52.8310667186017));
#11869=CARTESIAN_POINT('Ctrl Pts',(-3.35562237123423,0.481728953830529,
52.8336329966302));
#11870=CARTESIAN_POINT('Ctrl Pts',(-3.36566231985887,0.404853358648766,
52.8382024921641));
#11871=CARTESIAN_POINT('Ctrl Pts',(-3.36959871261343,0.370666612059013,
52.8402144915192));
#11872=CARTESIAN_POINT('Ctrl Pts',(-3.37698490169864,0.296612286757205,
52.844531814897));
#11873=CARTESIAN_POINT('Ctrl Pts',(-3.38025074163482,0.256731360692908,
52.8468312412225));
#11874=CARTESIAN_POINT('Ctrl Pts',(-3.38452747924999,0.190000076920932,
52.8506399303389));
#11875=CARTESIAN_POINT('Ctrl Pts',(-3.38592647032564,0.163181179021443,
52.8521601726888));
#11876=CARTESIAN_POINT('Ctrl Pts',(-3.3870066183502,0.136349659889395,52.8536715661706));
#11877=CARTESIAN_POINT('',(-3.38581326799137,0.000818680359414605,51.2660178032496));
#11878=CARTESIAN_POINT('Ctrl Pts',(-3.38743469189442,0.136371088936278,
52.5078428482942));
#11879=CARTESIAN_POINT('Ctrl Pts',(-3.34409159582951,1.00272967033552,52.4569067623586));
#11880=CARTESIAN_POINT('Ctrl Pts',(-2.48565222001799,2.96284343806158,52.3405530489097));
#11881=CARTESIAN_POINT('Ctrl Pts',(0.890051795839941,3.89117902226943,52.158781707947));
#11882=CARTESIAN_POINT('Ctrl Pts',(3.73656515455507,1.40411381468714,51.9625288254065));
#11883=CARTESIAN_POINT('Ctrl Pts',(3.23236205304029,-2.34203796083313,51.7662759428657));
#11884=CARTESIAN_POINT('Ctrl Pts',(-0.170370382920846,-3.98806386008981,
51.5700230603252));
#11885=CARTESIAN_POINT('Ctrl Pts',(-2.93186071344323,-2.34791161761635,
51.4032703471197));
#11886=CARTESIAN_POINT('Ctrl Pts',(-3.3833120129129,-0.613321193095971,
51.3019352614279));
#11887=CARTESIAN_POINT('Ctrl Pts',(-3.38470792471488,0.000818413090442893,
51.2660178032496));
#11888=CARTESIAN_POINT('Ctrl Pts',(-3.38974990090759,0.000819632226453476,
51.2660178032496));
#11889=CARTESIAN_POINT('Ctrl Pts',(-3.38973896871118,0.0460318755858765,
51.2633775331908));
#11890=CARTESIAN_POINT('Ctrl Pts',(-3.38882336922471,0.0912204861733642,
51.260737263132));
#11891=CARTESIAN_POINT('Ctrl Pts',(-3.38700661857411,0.136349654327206,
51.2580969930732));
#11892=CARTESIAN_POINT('Origin',(0.,0.,0.));
#11893=CARTESIAN_POINT('',(-3.38700661857411,0.136349654327212,28.));
#11894=CARTESIAN_POINT('Origin',(0.,0.,28.));
#11895=CARTESIAN_POINT('',(-3.38700661857411,0.136349654327212,50.));
#11896=CARTESIAN_POINT('',(-3.38700661857411,0.136349654327212,0.));
#11897=CARTESIAN_POINT('',(0.786086670334145,3.30023142332346,49.9983683068078));
#11898=CARTESIAN_POINT('Origin',(0.,0.,50.));
#11899=CARTESIAN_POINT('',(-3.38700661811317,0.13634966577722,50.3495735854002));
#11900=CARTESIAN_POINT('Ctrl Pts',(0.785310170844009,3.29752831649236,49.9967568224334));
#11901=CARTESIAN_POINT('Ctrl Pts',(0.746609307942668,3.30674497161701,49.9991821184928));
#11902=CARTESIAN_POINT('Ctrl Pts',(0.707750531259817,3.31527928317419,50.0016377255565));
#11903=CARTESIAN_POINT('Ctrl Pts',(0.450743211555314,3.36699988893547,50.0179748958375));
#11904=CARTESIAN_POINT('Ctrl Pts',(0.228953455097597,3.38931182096382,50.0324855428879));
#11905=CARTESIAN_POINT('Ctrl Pts',(-0.164263402961797,3.39007534803615,
50.0576378042822));
#11906=CARTESIAN_POINT('Ctrl Pts',(-0.334906605078102,3.37749079198311,
50.068370160301));
#11907=CARTESIAN_POINT('Ctrl Pts',(-0.55462065489123,3.34446296323699,50.0818357627315));
#11908=CARTESIAN_POINT('Ctrl Pts',(-0.605171315982537,3.33568653873055,
50.0849107259738));
#11909=CARTESIAN_POINT('Ctrl Pts',(-0.690689456111278,3.31883099074862,
50.0900761579914));
#11910=CARTESIAN_POINT('Ctrl Pts',(-0.725762169369974,3.31133817171354,
50.0921840802752));
#11911=CARTESIAN_POINT('Ctrl Pts',(-0.792631465371682,3.29593892778624,
50.0961849703029));
#11912=CARTESIAN_POINT('Ctrl Pts',(-0.824445060020095,3.2881253785261,50.0980805306922));
#11913=CARTESIAN_POINT('Ctrl Pts',(-0.908676532223715,3.2661383983955,50.1030814135789));
#11914=CARTESIAN_POINT('Ctrl Pts',(-0.960876609895461,3.25116435510229,
50.1061618659434));
#11915=CARTESIAN_POINT('Ctrl Pts',(-1.25430335787979,3.15930730586294,50.1234120561698));
#11916=CARTESIAN_POINT('Ctrl Pts',(-1.48667388182259,3.05684627039881,50.1367440097761));
#11917=CARTESIAN_POINT('Ctrl Pts',(-1.83576854494666,2.85360953247586,50.158354616456));
#11918=CARTESIAN_POINT('Ctrl Pts',(-1.96083938456098,2.7691575803534,50.1664915251561));
#11919=CARTESIAN_POINT('Ctrl Pts',(-2.10605221950588,2.6563224939898,50.176937725591));
#11920=CARTESIAN_POINT('Ctrl Pts',(-2.1319413911594,2.63558928487613,50.1788419978037));
#11921=CARTESIAN_POINT('Ctrl Pts',(-2.17363187534116,2.60118546863107,50.1819851336088));
#11922=CARTESIAN_POINT('Ctrl Pts',(-2.18961895312857,2.58774229155763,50.1832093048278));
#11923=CARTESIAN_POINT('Ctrl Pts',(-2.22194733711898,2.56004400476953,50.1857258995685));
#11924=CARTESIAN_POINT('Ctrl Pts',(-2.23827807376954,2.54577816874297,50.1870190523104));
#11925=CARTESIAN_POINT('Ctrl Pts',(-2.28276116009191,2.50616076360308,50.1905993904282));
#11926=CARTESIAN_POINT('Ctrl Pts',(-2.31062637683867,2.48049305170421,50.192907109681));
#11927=CARTESIAN_POINT('Ctrl Pts',(-2.47841443459673,2.32065635129221,50.2071749376582));
#11928=CARTESIAN_POINT('Ctrl Pts',(-2.60703696249065,2.17516273276916,50.2197089895251));
#11929=CARTESIAN_POINT('Ctrl Pts',(-2.84994425392242,1.84769433054061,50.2459143137803));
#11930=CARTESIAN_POINT('Ctrl Pts',(-2.96084551142556,1.66420383069609,50.2594969096643));
#11931=CARTESIAN_POINT('Ctrl Pts',(-3.07657251474616,1.42403581738916,50.275678802049));
#11932=CARTESIAN_POINT('Ctrl Pts',(-3.0983177787475,1.37608279090161,50.2788385498945));
#11933=CARTESIAN_POINT('Ctrl Pts',(-3.13299025812217,1.29462903260921,50.2840898257772));
#11934=CARTESIAN_POINT('Ctrl Pts',(-3.14651771998916,1.26139552590942,50.28620072154));
#11935=CARTESIAN_POINT('Ctrl Pts',(-3.172707477592,1.19400941833025,50.2904196061501));
#11936=CARTESIAN_POINT('Ctrl Pts',(-3.18535205776579,1.15985501045487,50.2925267965072));
#11937=CARTESIAN_POINT('Ctrl Pts',(-3.21589060270197,1.07309794581504,50.297805099226));
#11938=CARTESIAN_POINT('Ctrl Pts',(-3.23304658937067,1.02024595286799,50.3009524651739));
#11939=CARTESIAN_POINT('Ctrl Pts',(-3.3293154233636,0.696802911808041,50.3198491292813));
#11940=CARTESIAN_POINT('Ctrl Pts',(-3.37567739213672,0.417774362651803,
50.3345047438463));
#11941=CARTESIAN_POINT('Ctrl Pts',(-3.38700661811317,0.136349665777316,
50.3495735854002));
#11942=CARTESIAN_POINT('',(-3.38700661857411,0.136349654327281,50.0079012193304));
#11943=CARTESIAN_POINT('',(-3.38700661857411,0.136349654327212,0.));
#11944=CARTESIAN_POINT('',(-3.3787688286016,0.272628438300507,50.));
#11945=CARTESIAN_POINT('Ctrl Pts',(-3.38700661857411,0.136349654327351,
50.0079012193304));
#11946=CARTESIAN_POINT('Ctrl Pts',(-3.38700507140738,0.136388086870375,
50.0078990226929));
#11947=CARTESIAN_POINT('Ctrl Pts',(-3.3870035235907,0.13642651938927,50.0078968260301));
#11948=CARTESIAN_POINT('Ctrl Pts',(-3.38597226724431,0.16202186261079,50.0064338749809));
#11949=CARTESIAN_POINT('Ctrl Pts',(-3.38465335442818,0.187565683441125,
50.004963170781));
#11950=CARTESIAN_POINT('Ctrl Pts',(-3.38179470016056,0.232949742603296,
50.0023277969806));
#11951=CARTESIAN_POINT('Ctrl Pts',(-3.38036906961303,0.252796154913672,
50.0011677352365));
#11952=CARTESIAN_POINT('Ctrl Pts',(-3.3787688286016,0.272628438300507,50.));
#11953=CARTESIAN_POINT('Origin',(0.,0.,50.));
#11954=CARTESIAN_POINT('Origin',(0.,0.,0.));
#11955=CARTESIAN_POINT('Ctrl Pts',(-3.38700661811317,0.136349665777316,
50.3495735854002));
#11956=CARTESIAN_POINT('Ctrl Pts',(-3.38826066203953,0.105198470402101,
50.3512415713039));
#11957=CARTESIAN_POINT('Ctrl Pts',(-3.38908543079459,0.0740179861142426,
50.3529159549153));
#11958=CARTESIAN_POINT('Ctrl Pts',(-3.39081429351722,-0.0628422592113099,
50.3603018318282));
#11959=CARTESIAN_POINT('Ctrl Pts',(-3.38720763024682,-0.168497659618867,
50.3660982382046));
#11960=CARTESIAN_POINT('Ctrl Pts',(-3.37619544593572,-0.304386056493696,
50.373861742131));
#11961=CARTESIAN_POINT('Ctrl Pts',(-3.37330194467216,-0.334933441996331,
50.3756272594484));
#11962=CARTESIAN_POINT('Ctrl Pts',(-3.36782519952948,-0.385439113149716,
50.3785860061352));
#11963=CARTESIAN_POINT('Ctrl Pts',(-3.36547810227512,-0.40542201413453,
50.379767007702));
#11964=CARTESIAN_POINT('Ctrl Pts',(-3.36021440736446,-0.447035271618782,
50.3822500003375));
#11965=CARTESIAN_POINT('Ctrl Pts',(-3.35726658392158,-0.468660244976085,
50.3835534758816));
#11966=CARTESIAN_POINT('Ctrl Pts',(-3.34840228581628,-0.529305945517847,
50.3872430989558));
#11967=CARTESIAN_POINT('Ctrl Pts',(-3.34201302111642,-0.568252875777798,
50.3896523595134));
#11968=CARTESIAN_POINT('Ctrl Pts',(-3.30855473415173,-0.752054058905714,
50.4011835604538));
#11969=CARTESIAN_POINT('Ctrl Pts',(-3.27274021625441,-0.89514515717768,
50.410630314275));
#11970=CARTESIAN_POINT('Ctrl Pts',(-3.18548424477249,-1.16714446052443,
50.4290184106722));
#11971=CARTESIAN_POINT('Ctrl Pts',(-3.1352109698773,-1.29614479781498,50.4379383500371));
#11972=CARTESIAN_POINT('Ctrl Pts',(-3.02218025575127,-1.54079100775359,
50.4550073729889));
#11973=CARTESIAN_POINT('Ctrl Pts',(-2.96029622936766,-1.65658174036465,
50.4631587199742));
#11974=CARTESIAN_POINT('Ctrl Pts',(-2.86697385484724,-1.80918196803392,
50.4739670805158));
#11975=CARTESIAN_POINT('Ctrl Pts',(-2.84124164526892,-1.84933088892586,
50.4768181048648));
#11976=CARTESIAN_POINT('Ctrl Pts',(-2.79530057353443,-1.91778725608769,
50.4816945537671));
#11977=CARTESIAN_POINT('Ctrl Pts',(-2.77548791473621,-1.9463504886227,50.4837340295698));
#11978=CARTESIAN_POINT('Ctrl Pts',(-2.73354588082854,-2.0048737562823,50.4879248308165));
#11979=CARTESIAN_POINT('Ctrl Pts',(-2.71135498647931,-2.03478405662866,
50.4900734629393));
#11980=CARTESIAN_POINT('Ctrl Pts',(-2.6513849743876,-2.11289190962338,50.4957071611048));
#11981=CARTESIAN_POINT('Ctrl Pts',(-2.61278428946314,-2.16044287131503,
50.4991602394588));
#11982=CARTESIAN_POINT('Ctrl Pts',(-2.38981729272071,-2.42038614954167,
50.5182304973037));
#11983=CARTESIAN_POINT('Ctrl Pts',(-2.18087778385413,-2.61022403431013,
50.5327939180363));
#11984=CARTESIAN_POINT('Ctrl Pts',(-1.84993923394252,-2.8431264978651,50.554479288014));
#11985=CARTESIAN_POINT('Ctrl Pts',(-1.74519218241375,-2.90859796609916,
50.561193826104));
#11986=CARTESIAN_POINT('Ctrl Pts',(-1.60938415877447,-2.98350313292404,
50.5700078218592));
#11987=CARTESIAN_POINT('Ctrl Pts',(-1.58143696372896,-2.9984104606419,50.5718272254527));
#11988=CARTESIAN_POINT('Ctrl Pts',(-1.53531976546108,-3.02218577522506,
50.574845319316));
#11989=CARTESIAN_POINT('Ctrl Pts',(-1.51727126047909,-3.03128711080798,
50.576030414953));
#11990=CARTESIAN_POINT('Ctrl Pts',(-1.47985237606117,-3.04973844694305,
50.578497472976));
#11991=CARTESIAN_POINT('Ctrl Pts',(-1.46047271870659,-3.05906636625982,
50.5797804739509));
#11992=CARTESIAN_POINT('Ctrl Pts',(-1.40697689140364,-3.08419106254895,
50.5833338797222));
#11993=CARTESIAN_POINT('Ctrl Pts',(-1.37268554107248,-3.09960523902601,
50.5856246911011));
#11994=CARTESIAN_POINT('Ctrl Pts',(-1.15515967672149,-3.19306698094872,
50.6002063756298));
#11995=CARTESIAN_POINT('Ctrl Pts',(-0.965611784236614,-3.25540395352576,
50.6131093194901));
#11996=CARTESIAN_POINT('Ctrl Pts',(-0.568419468426531,-3.34826631767495,
50.6393410156936));
#11997=CARTESIAN_POINT('Ctrl Pts',(-0.361154943105755,-3.37691836337358,
50.6525951834277));
#11998=CARTESIAN_POINT('Ctrl Pts',(-0.0991440327766787,-3.3887214725872,
50.6685283423939));
#11999=CARTESIAN_POINT('Ctrl Pts',(-0.0456892563724606,-3.38986367444856,
50.6717389621893));
#12000=CARTESIAN_POINT('Ctrl Pts',(0.0437213682890569,-3.38965865990238,
50.6770449215391));
#12001=CARTESIAN_POINT('Ctrl Pts',(0.0796675943391308,-3.38900436853749,
50.6791607816298));
#12002=CARTESIAN_POINT('Ctrl Pts',(0.151682358896865,-3.38654708304739,
50.6833670669487));
#12003=CARTESIAN_POINT('Ctrl Pts',(0.187746023543892,-3.38473931918434,
50.6854570670065));
#12004=CARTESIAN_POINT('Ctrl Pts',(0.277968228511519,-3.37877026334543,
50.6906483448547));
#12005=CARTESIAN_POINT('Ctrl Pts',(0.33206941547825,-3.37388280555407,50.6937273556445));
#12006=CARTESIAN_POINT('Ctrl Pts',(0.64479091464955,-3.3380362042881,50.7113691915576));
#12007=CARTESIAN_POINT('Ctrl Pts',(0.899265220823585,-3.27865405311346,
50.7250211358607));
#12008=CARTESIAN_POINT('Ctrl Pts',(1.277081441481,-3.14313928076725,50.7464212444358));
#12009=CARTESIAN_POINT('Ctrl Pts',(1.40661389866871,-3.08734384367361,50.7540014877076));
#12010=CARTESIAN_POINT('Ctrl Pts',(1.56737206255776,-3.0058770775312,50.7641535609055));
#12011=CARTESIAN_POINT('Ctrl Pts',(1.60214388454224,-2.98748839098475,50.7663964741347));
#12012=CARTESIAN_POINT('Ctrl Pts',(1.65576673136436,-2.95792516865605,50.7699412553557));
#12013=CARTESIAN_POINT('Ctrl Pts',(1.67484366845317,-2.94716531636127,50.7712196291253));
#12014=CARTESIAN_POINT('Ctrl Pts',(1.7110949170622,-2.92625310504677,50.7736846367434));
#12015=CARTESIAN_POINT('Ctrl Pts',(1.72828612390148,-2.91613272148169,50.7748694119276));
#12016=CARTESIAN_POINT('Ctrl Pts',(1.77177397041937,-2.89001203745366,50.7779052089944));
#12017=CARTESIAN_POINT('Ctrl Pts',(1.79794350702348,-2.87380437391669,50.779768411163));
#12018=CARTESIAN_POINT('Ctrl Pts',(1.90812396471953,-2.8034719720309,50.787756853726));
#12019=CARTESIAN_POINT('Ctrl Pts',(1.98993481732703,-2.74600590434541,50.7940474610914));
#12020=CARTESIAN_POINT('Ctrl Pts',(2.07941931980257,-2.67704887957704,50.8012488981733));
#12021=CARTESIAN_POINT('Ctrl Pts',(2.08971144788955,-2.66902256861067,50.8020822044132));
#12022=CARTESIAN_POINT('Ctrl Pts',(2.33920773840247,-2.47212521838049,50.8224016295563));
#12023=CARTESIAN_POINT('Ctrl Pts',(2.55195419033199,-2.25186314665627,50.8422233236295));
#12024=CARTESIAN_POINT('Ctrl Pts',(2.7648108471223,-1.96194483195287,50.8640996161308));
#12025=CARTESIAN_POINT('Ctrl Pts',(2.79615982948518,-1.91700215701818,50.86739329103));
#12026=CARTESIAN_POINT('Ctrl Pts',(2.84636576997775,-1.84117192589998,50.8727940353639));
#12027=CARTESIAN_POINT('Ctrl Pts',(2.86584150458879,-1.81070836345626,50.8749233459621));
#12028=CARTESIAN_POINT('Ctrl Pts',(2.90362010169414,-1.74947887278681,50.8791256913018));
#12029=CARTESIAN_POINT('Ctrl Pts',(2.92193038749412,-1.71872306472263,50.8811988069719));
#12030=CARTESIAN_POINT('Ctrl Pts',(2.96604676899315,-1.64187733811533,50.8862896908081));
#12031=CARTESIAN_POINT('Ctrl Pts',(2.99126965412893,-1.59546259952072,50.8892869662395));
#12032=CARTESIAN_POINT('Ctrl Pts',(3.04369150994376,-1.49337975464593,50.8957265132123));
#12033=CARTESIAN_POINT('Ctrl Pts',(3.07047006879992,-1.43751703557933,50.8991549778405));
#12034=CARTESIAN_POINT('Ctrl Pts',(3.14847188970471,-1.26265871937509,50.9096383085556));
#12035=CARTESIAN_POINT('Ctrl Pts',(3.19441832538802,-1.14143611673253,50.9165550871717));
#12036=CARTESIAN_POINT('Ctrl Pts',(3.2999803841755,-0.806115290203916,50.935237920404));
#12037=CARTESIAN_POINT('Ctrl Pts',(3.34567261715104,-0.588340569558574,
50.9468782790256));
#12038=CARTESIAN_POINT('Ctrl Pts',(3.37357321334678,-0.33264385636009,50.9614335353705));
#12039=CARTESIAN_POINT('Ctrl Pts',(3.37685045289602,-0.297538190790384,
50.9634516204217));
#12040=CARTESIAN_POINT('Ctrl Pts',(3.38120630577591,-0.241434712943392,
50.9667171344041));
#12041=CARTESIAN_POINT('Ctrl Pts',(3.38263823971397,-0.220466077580982,
50.9679465923971));
#12042=CARTESIAN_POINT('Ctrl Pts',(3.38509349233651,-0.178817719287028,
50.9704087271372));
#12043=CARTESIAN_POINT('Ctrl Pts',(3.38612250565234,-0.158139326963475,
50.9716410761596));
#12044=CARTESIAN_POINT('Ctrl Pts',(3.38833211778515,-0.103692758148475,
50.9749096455387));
#12045=CARTESIAN_POINT('Ctrl Pts',(3.38919731902172,-0.0699147614432324,
50.9769614640334));
#12046=CARTESIAN_POINT('Ctrl Pts',(3.39144539304957,0.140984356942711,50.989899476896));
#12047=CARTESIAN_POINT('Ctrl Pts',(3.37944805712352,0.317961450163962,51.0013014153132));
#12048=CARTESIAN_POINT('Ctrl Pts',(3.32058220268071,0.718260439995007,51.0273503581134));
#12049=CARTESIAN_POINT('Ctrl Pts',(3.26490159203354,0.939472748909802,51.041903809923));
#12050=CARTESIAN_POINT('Ctrl Pts',(3.16763704817694,1.20825336871614,51.0593411196336));
#12051=CARTESIAN_POINT('Ctrl Pts',(3.14639793318988,1.26252973827489,51.0628526961353));
#12052=CARTESIAN_POINT('Ctrl Pts',(3.10948309290259,1.35013834081802,51.068507530299));
#12053=CARTESIAN_POINT('Ctrl Pts',(3.09464576630408,1.38380865136708,51.0706776188934));
#12054=CARTESIAN_POINT('Ctrl Pts',(3.06452005824452,1.44926369874454,51.0748919811378));
#12055=CARTESIAN_POINT('Ctrl Pts',(3.04927804288143,1.48106448503404,51.0769374713223));
#12056=CARTESIAN_POINT('Ctrl Pts',(3.01124948554602,1.55733019479729,51.0818413733612));
#12057=CARTESIAN_POINT('Ctrl Pts',(2.98797045065487,1.60154105357617,51.0846826833174));
#12058=CARTESIAN_POINT('Ctrl Pts',(2.88772764377693,1.78211950177047,51.0963035997398));
#12059=CARTESIAN_POINT('Ctrl Pts',(2.80233645084357,1.91359299465454,51.1047909677306));
#12060=CARTESIAN_POINT('Ctrl Pts',(2.62450155193859,2.1498238041335,51.120588265185));
#12061=CARTESIAN_POINT('Ctrl Pts',(2.53409034779772,2.25568973176625,51.1279114807518));
#12062=CARTESIAN_POINT('Ctrl Pts',(2.34755708273018,2.4486948039968,51.142280559732));
#12063=CARTESIAN_POINT('Ctrl Pts',(2.25244123554241,2.53646068588342,51.1492998749553));
#12064=CARTESIAN_POINT('Ctrl Pts',(2.12750804953232,2.6391600642915,51.1584845690548));
#12065=CARTESIAN_POINT('Ctrl Pts',(2.10216784750255,2.65938837396396,51.1603459586974));
#12066=CARTESIAN_POINT('Ctrl Pts',(2.06198820049496,2.69052946280075,51.1633018248083));
#12067=CARTESIAN_POINT('Ctrl Pts',(2.04734270757057,2.70169056936238,51.1643801409092));
#12068=CARTESIAN_POINT('Ctrl Pts',(2.01602156803004,2.72515901032878,51.1666898537986));
#12069=CARTESIAN_POINT('Ctrl Pts',(1.99932266557269,2.73743372839147,51.1679234501976));
#12070=CARTESIAN_POINT('Ctrl Pts',(1.95505893109681,2.76934923751482,51.1711967368812));
#12071=CARTESIAN_POINT('Ctrl Pts',(1.92731122310546,2.78873123203654,51.1732520767495));
#12072=CARTESIAN_POINT('Ctrl Pts',(1.86435461453637,2.83131856039307,51.1779147458144));
#12073=CARTESIAN_POINT('Ctrl Pts',(1.82899371716767,2.85428881029334,51.1805331487497));
#12074=CARTESIAN_POINT('Ctrl Pts',(1.71228718946605,2.92704152103061,51.189151517978));
#12075=CARTESIAN_POINT('Ctrl Pts',(1.62927004288795,2.97405058821817,51.1952444944297));
#12076=CARTESIAN_POINT('Ctrl Pts',(1.31320291347944,3.13581710690244,51.218054227701));
#12077=CARTESIAN_POINT('Ctrl Pts',(1.06914929048292,3.22719814109254,51.2348256630643));
#12078=CARTESIAN_POINT('Ctrl Pts',(0.756755189036587,3.30478201921148,51.2545202273031));
#12079=CARTESIAN_POINT('Ctrl Pts',(0.696074424957335,3.31809339150359,51.2582719191943));
#12080=CARTESIAN_POINT('Ctrl Pts',(0.598164907463169,3.33676707273177,51.2642101077037));
#12081=CARTESIAN_POINT('Ctrl Pts',(0.561155319407196,3.34319018751275,51.2664286967592));
#12082=CARTESIAN_POINT('Ctrl Pts',(0.489521157817721,3.35439938178435,51.2706748644592));
#12083=CARTESIAN_POINT('Ctrl Pts',(0.454914472380718,3.35926764811395,51.2727047261129));
#12084=CARTESIAN_POINT('Ctrl Pts',(0.372826140364179,3.36952350897208,51.2774719428083));
#12085=CARTESIAN_POINT('Ctrl Pts',(0.325293082510113,3.37444406334867,51.280194752315));
#12086=CARTESIAN_POINT('Ctrl Pts',(0.147596889819737,3.38904906566998,51.2902502451853));
#12087=CARTESIAN_POINT('Ctrl Pts',(0.0170081292474336,3.39221958541235,
51.2973885926618));
#12088=CARTESIAN_POINT('Ctrl Pts',(-0.252874782560523,3.3831820800764,51.3119167667793));
#12089=CARTESIAN_POINT('Ctrl Pts',(-0.391882060304622,3.36991034417655,
51.3192759000744));
#12090=CARTESIAN_POINT('Ctrl Pts',(-0.674657313741865,3.32517494142439,
51.3345195787468));
#12091=CARTESIAN_POINT('Ctrl Pts',(-0.817984027549354,3.2928476095757,51.3423967332442));
#12092=CARTESIAN_POINT('Ctrl Pts',(-0.996644941965798,3.24016431350472,
51.3528856327293));
#12093=CARTESIAN_POINT('Ctrl Pts',(-1.03433949712157,3.22832889352018,51.3551378653434));
#12094=CARTESIAN_POINT('Ctrl Pts',(-1.09259449605376,3.20891289933913,51.3586920747182));
#12095=CARTESIAN_POINT('Ctrl Pts',(-1.11330390725119,3.20178685767882,51.3599702013536));
#12096=CARTESIAN_POINT('Ctrl Pts',(-1.1529083576904,3.1877284109914,51.3624451994619));
#12097=CARTESIAN_POINT('Ctrl Pts',(-1.17181315036002,3.18082756018247,51.3636403816511));
#12098=CARTESIAN_POINT('Ctrl Pts',(-1.21945680171208,3.16295376060578,51.366685650754));
#12099=CARTESIAN_POINT('Ctrl Pts',(-1.24810947751682,3.15175728290683,51.3685477436155));
#12100=CARTESIAN_POINT('Ctrl Pts',(-1.37609403323414,3.09972649009205,51.376991300474));
#12101=CARTESIAN_POINT('Ctrl Pts',(-1.47359725627769,3.05457794910724,51.3837662181386));
#12102=CARTESIAN_POINT('Ctrl Pts',(-1.8234411821228,2.87193195696922,51.4089691175009));
#12103=CARTESIAN_POINT('Ctrl Pts',(-2.06021279408939,2.70712022312822,51.4276844349272));
#12104=CARTESIAN_POINT('Ctrl Pts',(-2.3224422219859,2.47002940924011,51.4493906312513));
#12105=CARTESIAN_POINT('Ctrl Pts',(-2.37021533579752,2.4242242716559,51.4533992210571));
#12106=CARTESIAN_POINT('Ctrl Pts',(-2.44374408004428,2.34947145429332,51.459659275503));
#12107=CARTESIAN_POINT('Ctrl Pts',(-2.47039540505616,2.32143230999211,51.4619484558853));
#12108=CARTESIAN_POINT('Ctrl Pts',(-2.51996675349378,2.26745888968959,51.4662472748003));
#12109=CARTESIAN_POINT('Ctrl Pts',(-2.54298073958333,2.24161801881715,51.4682606680281));
#12110=CARTESIAN_POINT('Ctrl Pts',(-2.59515928108421,2.18119222074448,51.4728696732307));
#12111=CARTESIAN_POINT('Ctrl Pts',(-2.62403553948191,2.14636645475345,51.4754535809631));
#12112=CARTESIAN_POINT('Ctrl Pts',(-2.71977396876846,2.02608151096315,51.4841485645555));
#12113=CARTESIAN_POINT('Ctrl Pts',(-2.78322965550586,1.9379918308852,51.4901314802297));
#12114=CARTESIAN_POINT('Ctrl Pts',(-2.94405356249563,1.69049987475813,51.5061386691015));
#12115=CARTESIAN_POINT('Ctrl Pts',(-3.03265169641367,1.52586559173489,51.515929248131));
#12116=CARTESIAN_POINT('Ctrl Pts',(-3.16356987145404,1.22559755007993,51.5334212304276));
#12117=CARTESIAN_POINT('Ctrl Pts',(-3.21177600473811,1.09304663090856,51.5410367137765));
#12118=CARTESIAN_POINT('Ctrl Pts',(-3.26083842657181,0.926503538899818,
51.5508932802624));
#12119=CARTESIAN_POINT('Ctrl Pts',(-3.26963087434435,0.894980351820823,
51.5527714711769));
#12120=CARTESIAN_POINT('Ctrl Pts',(-3.28267084537566,0.845469421872272,
51.5557479301081));
#12121=CARTESIAN_POINT('Ctrl Pts',(-3.2872302109388,0.827565059713995,51.5568296770401));
#12122=CARTESIAN_POINT('Ctrl Pts',(-3.29657728914046,0.789563204837427,
51.5591387703207));
#12123=CARTESIAN_POINT('Ctrl Pts',(-3.30132802622744,0.769457653527173,
51.5603682138607));
#12124=CARTESIAN_POINT('Ctrl Pts',(-3.31330767188874,0.716604480789697,
51.5636182725297));
#12125=CARTESIAN_POINT('Ctrl Pts',(-3.32023475482486,0.68379141546493,51.56565416774));
#12126=CARTESIAN_POINT('Ctrl Pts',(-3.33467145282173,0.610005144884213,
51.5702647852953));
#12127=CARTESIAN_POINT('Ctrl Pts',(-3.34191488328282,0.568985595155038,
51.5728502397294));
#12128=CARTESIAN_POINT('Ctrl Pts',(-3.36884386333107,0.398160727214537,
51.5836825681657));
#12129=CARTESIAN_POINT('Ctrl Pts',(-3.38172925503845,0.26744239336117,51.5921228543816));
#12130=CARTESIAN_POINT('Ctrl Pts',(-3.38700661379996,0.136349772919876,
51.6005689639805));
#12131=CARTESIAN_POINT('',(-3.38974999869979,9.38871559445019E-5,50.0160178032496));
#12132=CARTESIAN_POINT('Ctrl Pts',(-3.38700661857411,0.136349654327206,
51.2580969930732));
#12133=CARTESIAN_POINT('Ctrl Pts',(-3.38238609317346,0.251126257102754,
51.2513820182541));
#12134=CARTESIAN_POINT('Ctrl Pts',(-3.37193260407542,0.365517353525659,
51.244667043435));
#12135=CARTESIAN_POINT('Ctrl Pts',(-3.35574418187459,0.478942635724639,
51.2379520686159));
#12136=CARTESIAN_POINT('Ctrl Pts',(-3.33998514488251,0.589359401227443,
51.23141520324));
#12137=CARTESIAN_POINT('Ctrl Pts',(-3.31879173836351,0.6988606573217,51.2248783378641));
#12138=CARTESIAN_POINT('Ctrl Pts',(-3.29230537054002,0.806926520578764,
51.2183414724881));
#12139=CARTESIAN_POINT('Ctrl Pts',(-3.2647364948276,0.919409076614527,51.2115374429474));
#12140=CARTESIAN_POINT('Ctrl Pts',(-3.23143298620414,1.03033602875945,51.2047334134067));
#12141=CARTESIAN_POINT('Ctrl Pts',(-3.19260961647215,1.13914393265713,51.197929383866));
#12142=CARTESIAN_POINT('Ctrl Pts',(-3.15378624674016,1.24795183655482,51.1911253543253));
#12143=CARTESIAN_POINT('Ctrl Pts',(-3.10944323885395,1.3546403622979,51.1843213247846));
#12144=CARTESIAN_POINT('Ctrl Pts',(-3.05984868931851,1.45867441911338,51.1775172952438));
#12145=CARTESIAN_POINT('Ctrl Pts',(-3.01534232440451,1.55203503513846,51.1714113294782));
#12146=CARTESIAN_POINT('Ctrl Pts',(-2.96648525399577,1.64351199803028,51.1653053637126));
#12147=CARTESIAN_POINT('Ctrl Pts',(-2.91345995819217,1.73267311819365,51.159199397947));
#12148=CARTESIAN_POINT('Ctrl Pts',(-2.8605036792689,1.82171818766332,51.1531013796091));
#12149=CARTESIAN_POINT('Ctrl Pts',(-2.80339017764802,1.90845304315786,51.1470033612713));
#12150=CARTESIAN_POINT('Ctrl Pts',(-2.74234906458397,1.99246748291545,51.1409053429334));
#12151=CARTESIAN_POINT('Ctrl Pts',(-2.68137001247147,2.07639650457016,51.134813524496));
#12152=CARTESIAN_POINT('Ctrl Pts',(-2.61647153956889,2.15761026701092,51.1287217060585));
#12153=CARTESIAN_POINT('Ctrl Pts',(-2.54792758214111,2.23572585498861,51.1226298876211));
#12154=CARTESIAN_POINT('Ctrl Pts',(-2.47943149408921,2.31378688900438,51.1165423235564));
#12155=CARTESIAN_POINT('Ctrl Pts',(-2.4072952652929,2.38875373131041,51.1104547594917));
#12156=CARTESIAN_POINT('Ctrl Pts',(-2.33183378098951,2.46027565129117,51.104367195427));
#12157=CARTESIAN_POINT('Ctrl Pts',(-2.25639958327868,2.5317717092112,51.0982818326029));
#12158=CARTESIAN_POINT('Ctrl Pts',(-2.17764282950951,2.5998250272145,51.0921964697788));
#12159=CARTESIAN_POINT('Ctrl Pts',(-2.09591545520761,2.66412151883541,51.0861111069547));
#12160=CARTESIAN_POINT('Ctrl Pts',(-2.01419655095042,2.72841134690982,51.0800263748041));
#12161=CARTESIAN_POINT('Ctrl Pts',(-1.9295079740343,2.78894485889433,51.0739416426536));
#12162=CARTESIAN_POINT('Ctrl Pts',(-1.84223423472553,2.845448661794,51.0678569105031));
#12163=CARTESIAN_POINT('Ctrl Pts',(-1.75494702767579,2.90196118413879,51.0617712393806));
#12164=CARTESIAN_POINT('Ctrl Pts',(-1.66507422409557,2.95444252980832,51.055685568258));
#12165=CARTESIAN_POINT('Ctrl Pts',(-1.57302798386049,3.0026634883869,51.0495998971355));
#12166=CARTESIAN_POINT('Ctrl Pts',(-1.480886846121,3.05093416163735,51.0435079518295));
#12167=CARTESIAN_POINT('Ctrl Pts',(-1.38656817589773,3.09493547777582,51.0374160065234));
#12168=CARTESIAN_POINT('Ctrl Pts',(-1.29050729109405,3.13448496473234,51.0313240612174));
#12169=CARTESIAN_POINT('Ctrl Pts',(-1.19439439738538,3.17405586441594,51.0252288176344));
#12170=CARTESIAN_POINT('Ctrl Pts',(-1.09653781209418,3.20916998946029,51.0191335740514));
#12171=CARTESIAN_POINT('Ctrl Pts',(-0.997389454265164,3.23969432802242,
51.0130383304684));
#12172=CARTESIAN_POINT('Ctrl Pts',(-0.898082375398527,3.27026753128383,
51.0069333293523));
#12173=CARTESIAN_POINT('Ctrl Pts',(-0.797479806827848,3.29623616410636,
51.0008283282361));
#12174=CARTESIAN_POINT('Ctrl Pts',(-0.696045528625235,3.31751800064157,
50.99472332712));
#12175=CARTESIAN_POINT('Ctrl Pts',(-0.621505806011331,3.3331571141657,50.9902370223144));
#12176=CARTESIAN_POINT('Ctrl Pts',(-0.546517177004937,3.34626635828502,
50.9857507175088));
#12177=CARTESIAN_POINT('Ctrl Pts',(-0.471264993133025,3.35683100092145,
50.9812644127032));
#12178=CARTESIAN_POINT('Ctrl Pts',(-0.368976564799787,3.37119125780148,
50.9751662897786));
#12179=CARTESIAN_POINT('Ctrl Pts',(-0.265858260901948,3.38089616573506,
50.9690681668541));
#12180=CARTESIAN_POINT('Ctrl Pts',(-0.162370066605167,3.38585897874832,
50.9629700439296));
#12181=CARTESIAN_POINT('Ctrl Pts',(-0.0590172561375931,3.39081529938211,
50.9568798986033));
#12182=CARTESIAN_POINT('Ctrl Pts',(0.0447040585680405,3.39104183758612,
50.950789753277));
#12183=CARTESIAN_POINT('Ctrl Pts',(0.148326141367558,3.38650327303651,50.9446996079506));
#12184=CARTESIAN_POINT('Ctrl Pts',(0.251842401734575,3.38196934342502,50.93861568209));
#12185=CARTESIAN_POINT('Ctrl Pts',(0.355259206099814,3.37268000617653,50.9325317562294));
#12186=CARTESIAN_POINT('Ctrl Pts',(0.458107050130199,3.35865196070105,50.9264478303688));
#12187=CARTESIAN_POINT('Ctrl Pts',(0.560883025557151,3.34463371782325,50.9203681558687));
#12188=CARTESIAN_POINT('Ctrl Pts',(0.663090408115839,3.32588340899181,50.9142884813685));
#12189=CARTESIAN_POINT('Ctrl Pts',(0.764263886960711,3.30246964764064,50.9082088068684));
#12190=CARTESIAN_POINT('Ctrl Pts',(0.865400811614649,3.27906434573075,50.9021313289674));
#12191=CARTESIAN_POINT('Ctrl Pts',(0.965504158150382,3.25099903635872,50.8960538510664));
#12192=CARTESIAN_POINT('Ctrl Pts',(1.0641186988592,3.21839345904726,50.8899763731655));
#12193=CARTESIAN_POINT('Ctrl Pts',(1.16272323352482,3.18579119009999,50.8838995119231));
#12194=CARTESIAN_POINT('Ctrl Pts',(1.25983885614774,3.14864970375598,50.8778226506808));
#12195=CARTESIAN_POINT('Ctrl Pts',(1.35502628589034,3.10713836625378,50.8717457894384));
#12196=CARTESIAN_POINT('Ctrl Pts',(1.45022879016512,3.06562045473237,50.8656679658228));
#12197=CARTESIAN_POINT('Ctrl Pts',(1.5435021022964,3.01973148835263,50.8595901422072));
#12198=CARTESIAN_POINT('Ctrl Pts',(1.63442853190733,2.9696882726285,50.8535123185915));
#12199=CARTESIAN_POINT('Ctrl Pts',(1.72545008344898,2.91959270460901,50.8474281367111));
#12200=CARTESIAN_POINT('Ctrl Pts',(1.81411947369797,2.86533441547347,50.8413439548306));
#12201=CARTESIAN_POINT('Ctrl Pts',(1.90004521796449,2.80717531198005,50.8352597729502));
#12202=CARTESIAN_POINT('Ctrl Pts',(1.98601804169933,2.74898434260412,50.8291722574932));
#12203=CARTESIAN_POINT('Ctrl Pts',(2.06924388206197,2.68688855801591,50.8230847420362));
#12204=CARTESIAN_POINT('Ctrl Pts',(2.14936337133644,2.62119098130167,50.8169972265792));
#12205=CARTESIAN_POINT('Ctrl Pts',(2.22961307137135,2.55538663242126,50.810899817649));
#12206=CARTESIAN_POINT('Ctrl Pts',(2.30674601743564,2.48596908519958,50.8048024087188));
#12207=CARTESIAN_POINT('Ctrl Pts',(2.3804386759118,2.41327925709464,50.7987049997886));
#12208=CARTESIAN_POINT('Ctrl Pts',(2.43560463203426,2.35886401478006,50.7941405099133));
#12209=CARTESIAN_POINT('Ctrl Pts',(2.48884342648908,2.30261578862049,50.7895760200379));
#12210=CARTESIAN_POINT('Ctrl Pts',(2.5400344934993,2.24468925117348,50.7850115301626));
#12211=CARTESIAN_POINT('Ctrl Pts',(2.60861698763998,2.16708300760258,50.7788963206462));
#12212=CARTESIAN_POINT('Ctrl Pts',(2.6737522283564,2.08620330603658,50.7727811111299));
#12213=CARTESIAN_POINT('Ctrl Pts',(2.73511350553951,2.00238836750401,50.7666659016136));
#12214=CARTESIAN_POINT('Ctrl Pts',(2.79639464695022,1.91868288847337,50.760558678356));
#12215=CARTESIAN_POINT('Ctrl Pts',(2.85391137495837,1.83205013479395,50.7544514550985));
#12216=CARTESIAN_POINT('Ctrl Pts',(2.90737569847378,1.74286304981891,50.7483442318409));
#12217=CARTESIAN_POINT('Ctrl Pts',(2.96078530298451,1.6537672449387,50.7422432591287));
#12218=CARTESIAN_POINT('Ctrl Pts',(3.01015053355163,1.56212267104315,50.7361422864165));
#12219=CARTESIAN_POINT('Ctrl Pts',(3.055225880012,1.4683323481436,50.7300413137042));
#12220=CARTESIAN_POINT('Ctrl Pts',(3.1002689573856,1.37460916900013,50.7239447086305));
#12221=CARTESIAN_POINT('Ctrl Pts',(3.1410280749658,1.27874367860853,50.7178481035567));
#12222=CARTESIAN_POINT('Ctrl Pts',(3.17730338172666,1.18116395261976,50.711751498483));
#12223=CARTESIAN_POINT('Ctrl Pts',(3.21356515562498,1.08362062971441,50.7056571678082));
#12224=CARTESIAN_POINT('Ctrl Pts',(3.24534629552966,0.984364740910517,50.6995628371334));
#12225=CARTESIAN_POINT('Ctrl Pts',(3.27249517191522,0.88384411085417,50.6934685064585));
#12226=CARTESIAN_POINT('Ctrl Pts',(3.29964086532482,0.783335265990847,50.6873748902924));
#12227=CARTESIAN_POINT('Ctrl Pts',(3.3221552644091,0.681562385665184,50.6812812741263));
#12228=CARTESIAN_POINT('Ctrl Pts',(3.33993693075423,0.57898735831103,50.6751876579601));
#12229=CARTESIAN_POINT('Ctrl Pts',(3.35772106110552,0.476398117131597,50.6690931974014));
#12230=CARTESIAN_POINT('Ctrl Pts',(3.37077108308944,0.373006927482335,50.6629987368426));
#12231=CARTESIAN_POINT('Ctrl Pts',(3.37903703200953,0.269283862881242,50.6569042762839));
#12232=CARTESIAN_POINT('Ctrl Pts',(3.38731122028522,0.165457408914655,50.6508037408718));
#12233=CARTESIAN_POINT('Ctrl Pts',(3.39079177831328,0.0612988444033651,
50.6447032054596));
#12234=CARTESIAN_POINT('Ctrl Pts',(3.38948081194506,-0.0427187073333277,
50.6386026700475));
#12235=CARTESIAN_POINT('Ctrl Pts',(3.38816915803506,-0.146790811509927,
50.632498935184));
#12236=CARTESIAN_POINT('Ctrl Pts',(3.38206099820747,-0.250721330601563,
50.6263952003206));
#12237=CARTESIAN_POINT('Ctrl Pts',(3.37121045455189,-0.354041146789476,
50.6202914654572));
#12238=CARTESIAN_POINT('Ctrl Pts',(3.36034300140308,-0.457521976636091,
50.6141782185299));
#12239=CARTESIAN_POINT('Ctrl Pts',(3.34471846477157,-0.560389781347759,
50.6080649716027));
#12240=CARTESIAN_POINT('Ctrl Pts',(3.32444235334103,-0.662184341261841,
50.6019517246755));
#12241=CARTESIAN_POINT('Ctrl Pts',(3.30985630746213,-0.735412392222972,
50.5975540323243));
#12242=CARTESIAN_POINT('Ctrl Pts',(3.29286417536053,-0.808085261419362,
50.5931563399731));
#12243=CARTESIAN_POINT('Ctrl Pts',(3.27352104037737,-0.88003696553423,50.5887586476219));
#12244=CARTESIAN_POINT('Ctrl Pts',(3.24664850436202,-0.979996189407429,
50.58264913403));
#12245=CARTESIAN_POINT('Ctrl Pts',(3.21514945967312,-1.07888658774537,50.576539620438));
#12246=CARTESIAN_POINT('Ctrl Pts',(3.17912595974147,-1.17624963107238,50.570430106846));
#12247=CARTESIAN_POINT('Ctrl Pts',(3.14314874037317,-1.27348758892728,50.5643284423451));
#12248=CARTESIAN_POINT('Ctrl Pts',(3.10265876947978,-1.36920169648386,50.5582267778441));
#12249=CARTESIAN_POINT('Ctrl Pts',(3.05780841205472,-1.46294660793461,50.5521251133432));
#12250=CARTESIAN_POINT('Ctrl Pts',(3.01300295146507,-1.556597677327,50.5460295568298));
#12251=CARTESIAN_POINT('Ctrl Pts',(2.96384596785311,-1.64828308812112,50.5399340003165));
#12252=CARTESIAN_POINT('Ctrl Pts',(2.91053832948993,-1.73757638539144,50.5338384438032));
#12253=CARTESIAN_POINT('Ctrl Pts',(2.85726684321948,-1.82680912586984,50.527747021165));
#12254=CARTESIAN_POINT('Ctrl Pts',(2.79985051790869,-1.91365261387333,50.5216555985269));
#12255=CARTESIAN_POINT('Ctrl Pts',(2.73853629076501,-1.99770469455898,50.5155641758887));
#12256=CARTESIAN_POINT('Ctrl Pts',(2.67724349359053,-2.08172739815577,50.5094748822671));
#12257=CARTESIAN_POINT('Ctrl Pts',(2.61205575346245,-2.16296028953365,50.5033855886454));
#12258=CARTESIAN_POINT('Ctrl Pts',(2.54326304242446,-2.24103060209759,50.4972962950237));
#12259=CARTESIAN_POINT('Ctrl Pts',(2.47447670201679,-2.31909368486795,50.4912075653083));
#12260=CARTESIAN_POINT('Ctrl Pts',(2.4020863365294,-2.39399445144511,50.4851188355929));
#12261=CARTESIAN_POINT('Ctrl Pts',(2.32642128351071,-2.46539430398636,50.4790301058774));
#12262=CARTESIAN_POINT('Ctrl Pts',(2.25074379926239,-2.53680588701515,50.472940375827));
#12263=CARTESIAN_POINT('Ctrl Pts',(2.17179086853526,-2.60471512050655,50.4668506457766));
#12264=CARTESIAN_POINT('Ctrl Pts',(2.08992698377767,-2.66882188708388,50.4607609157262));
#12265=CARTESIAN_POINT('Ctrl Pts',(2.00797783578205,-2.73299542242639,50.4546648430731));
#12266=CARTESIAN_POINT('Ctrl Pts',(1.92311201553347,-2.79335831876617,50.4485687704199));
#12267=CARTESIAN_POINT('Ctrl Pts',(1.83572522232259,-2.84965225433362,50.4424726977667));
#12268=CARTESIAN_POINT('Ctrl Pts',(1.74829051866409,-2.9059770534624,50.4363732828972));
#12269=CARTESIAN_POINT('Ctrl Pts',(1.65833245748417,-2.95822823385694,50.4302738680277));
#12270=CARTESIAN_POINT('Ctrl Pts',(1.56627198999204,-3.00619312684105,50.4241744531582));
#12271=CARTESIAN_POINT('Ctrl Pts',(1.47406382635318,-3.05423497174671,50.4180652527629));
#12272=CARTESIAN_POINT('Ctrl Pts',(1.37974690559371,-3.09797661321588,50.4119560523677));
#12273=CARTESIAN_POINT('Ctrl Pts',(1.28376301401928,-3.13725319130225,50.4058468519724));
#12274=CARTESIAN_POINT('Ctrl Pts',(1.21389410839056,-3.16584352539604,50.4013998230087));
#12275=CARTESIAN_POINT('Ctrl Pts',(1.14314233688534,-3.1920689633944,50.396952794045));
#12276=CARTESIAN_POINT('Ctrl Pts',(1.07168247758956,-3.21588272947375,50.3925057650813));
#12277=CARTESIAN_POINT('Ctrl Pts',(0.974484192739338,-3.24827374229615,
50.3864570043894));
#12278=CARTESIAN_POINT('Ctrl Pts',(0.875636788894064,-3.27631376402613,
50.3804082436976));
#12279=CARTESIAN_POINT('Ctrl Pts',(0.775569533376517,-3.29983286870686,
50.3743594830057));
#12280=CARTESIAN_POINT('Ctrl Pts',(0.675634356763346,-3.32332093048986,
50.3683187060812));
#12281=CARTESIAN_POINT('Ctrl Pts',(0.574482948375973,-3.34229983416437,
50.3622779291567));
#12282=CARTESIAN_POINT('Ctrl Pts',(0.472561959383147,-3.35664866452299,
50.3562371522321));
#12283=CARTESIAN_POINT('Ctrl Pts',(0.370745031754765,-3.37098284472093,
50.3502025429429));
#12284=CARTESIAN_POINT('Ctrl Pts',(0.268160514506922,-3.3806962874626,50.3441679336537));
#12285=CARTESIAN_POINT('Ctrl Pts',(0.165266583023911,-3.38571883342897,
50.3381333243645));
#12286=CARTESIAN_POINT('Ctrl Pts',(0.062440570147767,-3.39073806409462,
50.3321026984225));
#12287=CARTESIAN_POINT('Ctrl Pts',(-0.0406940169840591,-3.39107252976694,
50.3260720724805));
#12288=CARTESIAN_POINT('Ctrl Pts',(-0.143673419542869,-3.38670385640919,
50.3200414465384));
#12289=CARTESIAN_POINT('Ctrl Pts',(-0.24661825811988,-3.3823366493519,50.3140128447143));
#12290=CARTESIAN_POINT('Ctrl Pts',(-0.349407580425442,-3.37326945722734,
50.3079842428901));
#12291=CARTESIAN_POINT('Ctrl Pts',(-0.451578116844336,-3.35953601958475,
50.3019556410659));
#12292=CARTESIAN_POINT('Ctrl Pts',(-0.553741992782523,-3.34580347722273,
50.2959274322453));
#12293=CARTESIAN_POINT('Ctrl Pts',(-0.655286730866545,-3.32740535195045,
50.2898992234247));
#12294=CARTESIAN_POINT('Ctrl Pts',(-0.755755695255239,-3.30442708976749,
50.2838710146042));
#12295=CARTESIAN_POINT('Ctrl Pts',(-0.856245283087935,-3.28144411079556,
50.2778415683623));
#12296=CARTESIAN_POINT('Ctrl Pts',(-0.955658233567042,-3.25387922458748,
50.2718121221205));
#12297=CARTESIAN_POINT('Ctrl Pts',(-1.05355059476116,-3.22186843411993,
50.2657826758787));
#12298=CARTESIAN_POINT('Ctrl Pts',(-1.15155783809582,-3.18982007720608,
50.2597461537458));
#12299=CARTESIAN_POINT('Ctrl Pts',(-1.24804051385002,-3.15331553394133,
50.2537096316129));
#12300=CARTESIAN_POINT('Ctrl Pts',(-1.34257233603639,-3.11253989291861,
50.2476731094799));
#12301=CARTESIAN_POINT('Ctrl Pts',(-1.43716132893339,-3.07173959170931,
50.2416329365948));
#12302=CARTESIAN_POINT('Ctrl Pts',(-1.52979672830863,-3.02666324234653,
50.2355927637096));
#12303=CARTESIAN_POINT('Ctrl Pts',(-1.62007662889155,-2.97754207006708,
50.2295525908245));
#12304=CARTESIAN_POINT('Ctrl Pts',(-1.71051958478066,-2.92833217961522,
50.223501508731));
#12305=CARTESIAN_POINT('Ctrl Pts',(-1.79859817213365,-2.87506310127268,
50.2174504266376));
#12306=CARTESIAN_POINT('Ctrl Pts',(-1.88393906443226,-2.81800969906175,
50.2113993445441));
#12307=CARTESIAN_POINT('Ctrl Pts',(-1.95514465282031,-2.77040624701729,
50.2063505238763));
#12308=CARTESIAN_POINT('Ctrl Pts',(-2.02444480706955,-2.72016911359938,
50.2013017032085));
#12309=CARTESIAN_POINT('Ctrl Pts',(-2.09164155441515,-2.66747833549661,
50.1962528825407));
#12310=CARTESIAN_POINT('Ctrl Pts',(-2.17420186419761,-2.60274057459771,
50.1900497221968));
#12311=CARTESIAN_POINT('Ctrl Pts',(-2.25388088605287,-2.53406697426379,
50.1838465618529));
#12312=CARTESIAN_POINT('Ctrl Pts',(-2.33028851954139,-2.46173931970743,
50.177643401509));
#12313=CARTESIAN_POINT('Ctrl Pts',(-2.40658582881859,-2.38951609832196,
50.1714491978458));
#12314=CARTESIAN_POINT('Ctrl Pts',(-2.47962085078108,-2.31364960005651,
50.1652549941826));
#12315=CARTESIAN_POINT('Ctrl Pts',(-2.54903549203045,-2.23446260270095,
50.1590607905194));
#12316=CARTESIAN_POINT('Ctrl Pts',(-2.61835116314992,-2.15538850872244,
50.1528754184388));
#12317=CARTESIAN_POINT('Ctrl Pts',(-2.68405646356693,-2.0730036513876,50.1466900463582));
#12318=CARTESIAN_POINT('Ctrl Pts',(-2.74582992284387,-1.98766775325134,
50.1405046742776));
#12319=CARTESIAN_POINT('Ctrl Pts',(-2.80755240900049,-1.90240227106804,
50.134324406132));
#12320=CARTESIAN_POINT('Ctrl Pts',(-2.86534926738651,-1.81419092354675,
50.1281441379863));
#12321=CARTESIAN_POINT('Ctrl Pts',(-2.91893923119918,-1.72342647857875,
50.1219638698406));
#12322=CARTESIAN_POINT('Ctrl Pts',(-2.97249733481119,-1.63271599471137,
50.1157872759759));
#12323=CARTESIAN_POINT('Ctrl Pts',(-3.02185331151303,-1.53945578678077,
50.1096106821112));
#12324=CARTESIAN_POINT('Ctrl Pts',(-3.06676957025133,-1.44406698787849,
50.1034340882465));
#12325=CARTESIAN_POINT('Ctrl Pts',(-3.11166948095893,-1.34871290734005,
50.0972597424574));
#12326=CARTESIAN_POINT('Ctrl Pts',(-3.15213271525814,-1.25123214969023,
50.0910853966683));
#12327=CARTESIAN_POINT('Ctrl Pts',(-3.18796827153445,-1.15206916554071,
50.0849110508792));
#12328=CARTESIAN_POINT('Ctrl Pts',(-3.22380944156518,-1.05289064719278,
50.0787357378591));
#12329=CARTESIAN_POINT('Ctrl Pts',(-3.25502133760869,-0.952029759991573,
50.072560424839));
#12330=CARTESIAN_POINT('Ctrl Pts',(-3.28146174758333,-0.849949328870463,
50.0663851118189));
#12331=CARTESIAN_POINT('Ctrl Pts',(-3.30790346808446,-0.747863838103573,
50.0602094927176));
#12332=CARTESIAN_POINT('Ctrl Pts',(-3.3295731347263,-0.644559083050461,
50.0540338736164));
#12333=CARTESIAN_POINT('Ctrl Pts',(-3.34637920118809,-0.540510225949323,
50.0478582545151));
#12334=CARTESIAN_POINT('Ctrl Pts',(-3.36319782829134,-0.436383604048632,
50.0416780198343));
#12335=CARTESIAN_POINT('Ctrl Pts',(-3.37514553356435,-0.331512176604862,
50.0354977851534));
#12336=CARTESIAN_POINT('Ctrl Pts',(-3.38218241566213,-0.226378377249048,
50.0293175504725));
#12337=CARTESIAN_POINT('Ctrl Pts',(-3.38723016104025,-0.150963066546201,
50.0248843013982));
#12338=CARTESIAN_POINT('Ctrl Pts',(-3.38975209003901,-0.0754128960838142,
50.0204510523239));
#12339=CARTESIAN_POINT('Ctrl Pts',(-3.38974999869979,9.38871559445019E-5,
50.0160178032496));
#12340=CARTESIAN_POINT('Ctrl Pts',(-3.38974999927235,7.02360661182119E-5,
50.0155995406885));
#12341=CARTESIAN_POINT('Ctrl Pts',(-3.38974905771225,0.0455120371475817,
50.0130593630806));
#12342=CARTESIAN_POINT('Ctrl Pts',(-3.38883435054036,0.0909477037524909,
50.0104961979471));
#12343=CARTESIAN_POINT('Ctrl Pts',(-3.38700661857411,0.136349654327351,
50.0079012193304));
#12344=CARTESIAN_POINT('Origin',(0.,0.,46.4896150285955));
#12345=CARTESIAN_POINT('',(-4.08499869890724,-0.00326035675198677,52.1146150285711));
#12346=CARTESIAN_POINT('Ctrl Pts',(-2.31338095599002,-3.36682247118299,
51.0573853382455));
#12347=CARTESIAN_POINT('Ctrl Pts',(-2.21485531346751,-3.43452052982407,
51.0631908707828));
#12348=CARTESIAN_POINT('Ctrl Pts',(-2.11333489385848,-3.49790437700326,
51.0689964033201));
#12349=CARTESIAN_POINT('Ctrl Pts',(-2.00923758994844,-3.55671046152736,
51.0748019358575));
#12350=CARTESIAN_POINT('Ctrl Pts',(-1.90513465637732,-3.61551972632908,
51.0806077823624));
#12351=CARTESIAN_POINT('Ctrl Pts',(-1.79845491668258,-3.66975053568956,
51.0864136288673));
#12352=CARTESIAN_POINT('Ctrl Pts',(-1.6896416456048,-3.71918487164028,51.0922194753723));
#12353=CARTESIAN_POINT('Ctrl Pts',(-1.58079687153331,-3.76863351953621,
51.0980270027526));
#12354=CARTESIAN_POINT('Ctrl Pts',(-1.46981770892226,-3.8132827636905,51.1038345301329));
#12355=CARTESIAN_POINT('Ctrl Pts',(-1.3571676249016,-3.85296263126428,51.1096420575131));
#12356=CARTESIAN_POINT('Ctrl Pts',(-1.24439571494977,-3.89268541080619,
51.1154558654696));
#12357=CARTESIAN_POINT('Ctrl Pts',(-1.12994966124609,-3.92742794946554,
51.121269673426));
#12358=CARTESIAN_POINT('Ctrl Pts',(-1.01430848479722,-3.9570700395202,51.1270834813825));
#12359=CARTESIAN_POINT('Ctrl Pts',(-0.898595034237535,-3.98673065546474,
51.1329009228872));
#12360=CARTESIAN_POINT('Ctrl Pts',(-0.781685371760786,-4.01128439002637,
51.138718364392));
#12361=CARTESIAN_POINT('Ctrl Pts',(-0.664067470212348,-4.03066240151737,
51.1445358058967));
#12362=CARTESIAN_POINT('Ctrl Pts',(-0.54627905099552,-4.05006850646433,
51.1503616812925));
#12363=CARTESIAN_POINT('Ctrl Pts',(-0.427780746829687,-4.06428385975495,
51.1561875566882));
#12364=CARTESIAN_POINT('Ctrl Pts',(-0.309064608487866,-4.07329155202279,
51.1620134320839));
#12365=CARTESIAN_POINT('Ctrl Pts',(-0.264187796497275,-4.07669661992695,
51.164215716613));
#12366=CARTESIAN_POINT('Ctrl Pts',(-0.219279844602496,-4.07935805925082,
51.166418001142));
#12367=CARTESIAN_POINT('Ctrl Pts',(-0.17436721939883,-4.08127689244422,
51.168620285671));
#12368=CARTESIAN_POINT('Ctrl Pts',(-0.0555365400593207,-4.08635377786066,
51.1744471320309));
#12369=CARTESIAN_POINT('Ctrl Pts',(0.0637050618138584,-4.08624461472206,
51.1802739783909));
#12370=CARTESIAN_POINT('Ctrl Pts',(0.182868281360663,-4.0809048251181,51.1861008247508));
#12371=CARTESIAN_POINT('Ctrl Pts',(0.301882461461882,-4.07557171407893,
51.1919203833758));
#12372=CARTESIAN_POINT('Ctrl Pts',(0.420818050366714,-4.06502100708473,
51.1977399420009));
#12373=CARTESIAN_POINT('Ctrl Pts',(0.539182790279408,-4.04926004581905,
51.2035595006259));
#12374=CARTESIAN_POINT('Ctrl Pts',(0.657430234058117,-4.03351470322347,
51.2093732922318));
#12375=CARTESIAN_POINT('Ctrl Pts',(0.775107552319402,-4.01256943182584,
51.2151870838376));
#12376=CARTESIAN_POINT('Ctrl Pts',(0.89172525873247,-3.9864835460514,51.2210008754435));
#12377=CARTESIAN_POINT('Ctrl Pts',(1.01197134723284,-3.95958603772334,51.2269955543088));
#12378=CARTESIAN_POINT('Ctrl Pts',(1.13109036807526,-3.92722281822845,51.2329902331742));
#12379=CARTESIAN_POINT('Ctrl Pts',(1.24855402613677,-3.88951640230732,51.2389849120395));
#12380=CARTESIAN_POINT('Ctrl Pts',(1.36234726760442,-3.85298820828882,51.2447922736601));
#12381=CARTESIAN_POINT('Ctrl Pts',(1.47458664040822,-3.81144590016996,51.2505996352808));
#12382=CARTESIAN_POINT('Ctrl Pts',(1.58480557157098,-3.76505196515501,51.2564069969014));
#12383=CARTESIAN_POINT('Ctrl Pts',(1.69500873526949,-3.71866466706443,51.2622135277449));
#12384=CARTESIAN_POINT('Ctrl Pts',(1.8031916564231,-3.66742728057848,51.2680200585884));
#12385=CARTESIAN_POINT('Ctrl Pts',(1.90890733784516,-3.61155060542157,51.2738265894319));
#12386=CARTESIAN_POINT('Ctrl Pts',(2.01463276006086,-3.55566878170813,51.2796336552974));
#12387=CARTESIAN_POINT('Ctrl Pts',(2.11789013001795,-3.49514700996815,51.285440721163));
#12388=CARTESIAN_POINT('Ctrl Pts',(2.21825724068107,-3.43024194688451,51.2912477870285));
#12389=CARTESIAN_POINT('Ctrl Pts',(2.31865720517891,-3.36531563799433,51.2970567537596));
#12390=CARTESIAN_POINT('Ctrl Pts',(2.41616468655407,-3.29600340549605,51.3028657204907));
#12391=CARTESIAN_POINT('Ctrl Pts',(2.51038716963343,-3.22260473197379,51.3086746872217));
#12392=CARTESIAN_POINT('Ctrl Pts',(2.60471317050794,-3.14912541879312,51.3144900359904));
#12393=CARTESIAN_POINT('Ctrl Pts',(2.69574664744501,-3.07155095401748,51.3203053847591));
#12394=CARTESIAN_POINT('Ctrl Pts',(2.78312873585002,-2.99022063394758,51.3261207335277));
#12395=CARTESIAN_POINT('Ctrl Pts',(2.87056836554361,-2.90883675769125,51.3319399117157));
#12396=CARTESIAN_POINT('Ctrl Pts',(2.95435153272342,-2.82369239045701,51.3377590899038));
#12397=CARTESIAN_POINT('Ctrl Pts',(3.03415789412681,-2.73516194648652,51.3435782680918));
#12398=CARTESIAN_POINT('Ctrl Pts',(3.11407652144017,-2.64650696418754,51.3494056322856));
#12399=CARTESIAN_POINT('Ctrl Pts',(3.19000691928114,-2.55445671187275,51.3552329964794));
#12400=CARTESIAN_POINT('Ctrl Pts',(3.26167041649538,-2.45941681993086,51.3610603606732));
#12401=CARTESIAN_POINT('Ctrl Pts',(3.27730007416623,-2.43868881984896,51.3623312965193));
#12402=CARTESIAN_POINT('Ctrl Pts',(3.29272693884235,-2.41781871297285,51.3636022323655));
#12403=CARTESIAN_POINT('Ctrl Pts',(3.30794840624843,-2.39681086896702,51.3648731682117));
#12404=CARTESIAN_POINT('Ctrl Pts',(3.37773264172279,-2.30049845086699,51.3706998920089));
#12405=CARTESIAN_POINT('Ctrl Pts',(3.44341813786752,-2.20098258530104,51.376526615806));
#12406=CARTESIAN_POINT('Ctrl Pts',(3.50469780021593,-2.0986467852313,51.3823533396032));
#12407=CARTESIAN_POINT('Ctrl Pts',(3.5659008220121,-1.99643897333789,51.3881727760996));
#12408=CARTESIAN_POINT('Ctrl Pts',(3.62270876242533,-1.89141858877044,51.393992212596));
#12409=CARTESIAN_POINT('Ctrl Pts',(3.67485620291266,-1.78400024885489,51.3998116490924));
#12410=CARTESIAN_POINT('Ctrl Pts',(3.72695197092691,-1.6766883488955,51.4056253191567));
#12411=CARTESIAN_POINT('Ctrl Pts',(3.77439624928288,-1.5669835855383,51.411438989221));
#12412=CARTESIAN_POINT('Ctrl Pts',(3.81696849768409,-1.45532693498308,51.4172526592853));
#12413=CARTESIAN_POINT('Ctrl Pts',(3.86086656961436,-1.34019297185826,51.4232473839297));
#12414=CARTESIAN_POINT('Ctrl Pts',(3.89958395878201,-1.22298393522567,51.4292421085742));
#12415=CARTESIAN_POINT('Ctrl Pts',(3.93293141597882,-1.10420807695236,51.4352368332187));
#12416=CARTESIAN_POINT('Ctrl Pts',(3.96523594665418,-0.989146879499215,
51.4410440755827));
#12417=CARTESIAN_POINT('Ctrl Pts',(3.99250130578342,-0.872615824488559,
51.4468513179468));
#12418=CARTESIAN_POINT('Ctrl Pts',(4.01460564908539,-0.755093691095127,
51.4526585603109));
#12419=CARTESIAN_POINT('Ctrl Pts',(4.03670683422612,-0.637588348693489,
51.4584649729644));
#12420=CARTESIAN_POINT('Ctrl Pts',(4.05364839468815,-0.519092610191553,
51.4642713856178));
#12421=CARTESIAN_POINT('Ctrl Pts',(4.06535958175131,-0.400095577409752,
51.4700777982713));
#12422=CARTESIAN_POINT('Ctrl Pts',(4.07707185035241,-0.281087555152209,
51.4758847471519));
#12423=CARTESIAN_POINT('Ctrl Pts',(4.08355274523143,-0.161578552421022,
51.4816916960324));
#12424=CARTESIAN_POINT('Ctrl Pts',(4.08478344148044,-0.0420622896098659,
51.487498644913));
#12425=CARTESIAN_POINT('Ctrl Pts',(4.08601454087451,0.0774931237154308,
51.4933074960036));
#12426=CARTESIAN_POINT('Ctrl Pts',(4.08199201701098,0.197055394294678,51.4991163470942));
#12427=CARTESIAN_POINT('Ctrl Pts',(4.07274914450126,0.316131943916218,51.5049251981848));
#12428=CARTESIAN_POINT('Ctrl Pts',(4.06349611297606,0.435339372819054,51.5107404338931));
#12429=CARTESIAN_POINT('Ctrl Pts',(4.04901131164756,0.554059608373962,51.5165556696015));
#12430=CARTESIAN_POINT('Ctrl Pts',(4.02937978590845,0.671806178084404,51.5223709053099));
#12431=CARTESIAN_POINT('Ctrl Pts',(4.00973532784342,0.789630313697542,51.528189971822));
#12432=CARTESIAN_POINT('Ctrl Pts',(3.9849374775445,0.906479108090121,51.5340090383342));
#12433=CARTESIAN_POINT('Ctrl Pts',(3.95512182112969,1.02187884801661,51.5398281048464));
#12434=CARTESIAN_POINT('Ctrl Pts',(3.92526420674824,1.13744098377875,51.5456553602173));
#12435=CARTESIAN_POINT('Ctrl Pts',(3.89037481199442,1.25154960673471,51.5514826155882));
#12436=CARTESIAN_POINT('Ctrl Pts',(3.85063824722395,1.3637485431765,51.5573098709591));
#12437=CARTESIAN_POINT('Ctrl Pts',(3.84196395913701,1.38824099498674,51.5585819308902));
#12438=CARTESIAN_POINT('Ctrl Pts',(3.83305886807873,1.41264253115848,51.5598539908213));
#12439=CARTESIAN_POINT('Ctrl Pts',(3.82392518819003,1.43694855688219,51.5611260507524));
#12440=CARTESIAN_POINT('Ctrl Pts',(3.78208928498747,1.54827986603781,51.5669525934814));
#12441=CARTESIAN_POINT('Ctrl Pts',(3.73532072835553,1.65795986297884,51.5727791362104));
#12442=CARTESIAN_POINT('Ctrl Pts',(3.68376995515531,1.76552086294528,51.5786056789395));
#12443=CARTESIAN_POINT('Ctrl Pts',(3.63228368614921,1.87294727452067,51.5844249310612));
#12444=CARTESIAN_POINT('Ctrl Pts',(3.57602727748281,1.97825959835997,51.5902441831829));
#12445=CARTESIAN_POINT('Ctrl Pts',(3.51520010096128,2.08100774871259,51.5960634353047));
#12446=CARTESIAN_POINT('Ctrl Pts',(3.45443323148049,2.18365402951865,51.6018769179349));
#12447=CARTESIAN_POINT('Ctrl Pts',(3.38910481626058,2.28374084551855,51.6076904005652));
#12448=CARTESIAN_POINT('Ctrl Pts',(3.31946097070129,2.38084099930903,51.6135038831955));
#12449=CARTESIAN_POINT('Ctrl Pts',(3.24764507016129,2.48096951649582,51.6194986769496));
#12450=CARTESIAN_POINT('Ctrl Pts',(3.17124033780107,2.57792162304733,51.6254934707036));
#12451=CARTESIAN_POINT('Ctrl Pts',(3.09056630564523,2.67125904966374,51.6314882644577));
#12452=CARTESIAN_POINT('Ctrl Pts',(3.01241882673005,2.76167333023932,51.637295312971));
#12453=CARTESIAN_POINT('Ctrl Pts',(2.93026575552348,2.84869563009802,51.6431023614844));
#12454=CARTESIAN_POINT('Ctrl Pts',(2.84443918786769,2.93196021571279,51.6489094099977));
#12455=CARTESIAN_POINT('Ctrl Pts',(2.75862491330545,3.0152128751913,51.6547156267571));
#12456=CARTESIAN_POINT('Ctrl Pts',(2.6691384813639,3.09470860694659,51.6605218435164));
#12457=CARTESIAN_POINT('Ctrl Pts',(2.57634878563552,3.17011859947769,51.6663280602758));
#12458=CARTESIAN_POINT('Ctrl Pts',(2.48355054971071,3.24553553260865,51.6721348114288));
#12459=CARTESIAN_POINT('Ctrl Pts',(2.38744876202428,3.31686572162996,51.6779415625819));
#12460=CARTESIAN_POINT('Ctrl Pts',(2.28844481299793,3.38382111493248,51.683748313735));
#12461=CARTESIAN_POINT('Ctrl Pts',(2.18940845936944,3.45079842314751,51.6895569654735));
#12462=CARTESIAN_POINT('Ctrl Pts',(2.08746839288154,3.51339785952447,51.695365617212));
#12463=CARTESIAN_POINT('Ctrl Pts',(1.98305379253874,3.57137545714501,51.7011742689505));
#12464=CARTESIAN_POINT('Ctrl Pts',(1.87852444961677,3.62941676711097,51.7069893038928));
#12465=CARTESIAN_POINT('Ctrl Pts',(1.77151550180268,3.68282590245674,51.7128043388352));
#12466=CARTESIAN_POINT('Ctrl Pts',(1.66247959503268,3.73140544515066,51.7186193737776));
#12467=CARTESIAN_POINT('Ctrl Pts',(1.55337187785856,3.78001698204443,51.7244382384676));
#12468=CARTESIAN_POINT('Ctrl Pts',(1.44223492164552,3.82379244249884,51.7302571031576));
#12469=CARTESIAN_POINT('Ctrl Pts',(1.32953861083212,3.86258360198282,51.7360759678477));
#12470=CARTESIAN_POINT('Ctrl Pts',(1.21668370371905,3.90142935184612,51.7419030213631));
#12471=CARTESIAN_POINT('Ctrl Pts',(1.10226545186857,3.93527668611693,51.7477300748784));
#12472=CARTESIAN_POINT('Ctrl Pts',(0.986766154322983,3.96402794600172,51.7535571283938));
#12473=CARTESIAN_POINT('Ctrl Pts',(0.961515211741925,3.97031366745555,51.7548310633602));
#12474=CARTESIAN_POINT('Ctrl Pts',(0.936212625199436,3.97635601021811,51.7561049983266));
#12475=CARTESIAN_POINT('Ctrl Pts',(0.91086347119859,3.98215428340441,51.7573789332929));
#12476=CARTESIAN_POINT('Ctrl Pts',(0.794922507767534,4.00867419722217,51.7632056069304));
#12477=CARTESIAN_POINT('Ctrl Pts',(0.677637888103198,4.03016865893983,51.7690322805679));
#12478=CARTESIAN_POINT('Ctrl Pts',(0.5594827134802,4.04650517030645,51.7748589542053));
#12479=CARTESIAN_POINT('Ctrl Pts',(0.44147534529509,4.06282124548346,51.7806783389545));
#12480=CARTESIAN_POINT('Ctrl Pts',(0.322599988750864,4.07399214894305,51.7864977237036));
#12481=CARTESIAN_POINT('Ctrl Pts',(0.203342057658757,4.07993590728912,51.7923171084527));
#12482=CARTESIAN_POINT('Ctrl Pts',(0.0842023303830821,4.08587377441342,
51.7981307252543));
#12483=CARTESIAN_POINT('Ctrl Pts',(-0.0353188120385766,4.08659478343787,
51.803944342056));
#12484=CARTESIAN_POINT('Ctrl Pts',(-0.154729263620538,4.08206857548712,
51.8097579588576));
#12485=CARTESIAN_POINT('Ctrl Pts',(-0.277860030136686,4.07740135040754,
51.8157527028983));
#12486=CARTESIAN_POINT('Ctrl Pts',(-0.400872658223365,4.06715453202206,
51.8217474469389));
#12487=CARTESIAN_POINT('Ctrl Pts',(-0.523225359481639,4.05135288801103,
51.8277421909796));
#12488=CARTESIAN_POINT('Ctrl Pts',(-0.641749994926215,4.03604563221225,
51.8335493766379));
#12489=CARTESIAN_POINT('Ctrl Pts',(-0.759654948262934,4.01552601377994,
51.8393565622962));
#12490=CARTESIAN_POINT('Ctrl Pts',(-0.876451953488757,3.98986929274954,
51.8451637479545));
#12491=CARTESIAN_POINT('Ctrl Pts',(-0.993232247399792,3.96421624268264,
51.8509701027208));
#12492=CARTESIAN_POINT('Ctrl Pts',(-1.10890451027023,3.93342763929747,51.856776457487));
#12493=CARTESIAN_POINT('Ctrl Pts',(-1.22299097464946,3.89762980231909,51.8625828122532));
#12494=CARTESIAN_POINT('Ctrl Pts',(-1.33708795306209,3.86182866626702,51.8683897021242));
#12495=CARTESIAN_POINT('Ctrl Pts',(-1.44959845329711,3.82101750085935,51.8741965919952));
#12496=CARTESIAN_POINT('Ctrl Pts',(-1.56006077978372,3.77537221521013,51.8800034818662));
#12497=CARTESIAN_POINT('Ctrl Pts',(-1.67055927107023,3.72971198552817,51.8858122728831));
#12498=CARTESIAN_POINT('Ctrl Pts',(-1.77900787829312,3.67921464363256,51.8916210639001));
#12499=CARTESIAN_POINT('Ctrl Pts',(-1.88496634784923,3.62410359502539,51.8974298549171));
#12500=CARTESIAN_POINT('Ctrl Pts',(-1.99104125621177,3.56893198434377,51.9032450292717));
#12501=CARTESIAN_POINT('Ctrl Pts',(-2.09462020294267,3.50913673530709,51.9090602036264));
#12502=CARTESIAN_POINT('Ctrl Pts',(-2.1952888154897,3.44498650455787,51.9148753779811));
#12503=CARTESIAN_POINT('Ctrl Pts',(-2.29602373029234,3.3807940232512,51.9206943823198));
#12504=CARTESIAN_POINT('Ctrl Pts',(-2.39384416028491,3.31224108133478,51.9265133866584));
#12505=CARTESIAN_POINT('Ctrl Pts',(-2.48836725530378,3.23963785055242,51.9323323909971));
#12506=CARTESIAN_POINT('Ctrl Pts',(-2.5830233571213,3.16693245718963,51.9381595834631));
#12507=CARTESIAN_POINT('Ctrl Pts',(-2.67437255274091,3.09016566156676,51.9439867759292));
#12508=CARTESIAN_POINT('Ctrl Pts',(-2.76206731988696,3.00968588401057,51.9498139683952));
#12509=CARTESIAN_POINT('Ctrl Pts',(-2.78121920958726,2.99210969476892,51.951086584208));
#12510=CARTESIAN_POINT('Ctrl Pts',(-2.80019694882373,2.97435654342491,51.9523592000208));
#12511=CARTESIAN_POINT('Ctrl Pts',(-2.81899717149045,2.95643027097357,51.9536318158336));
#12512=CARTESIAN_POINT('Ctrl Pts',(-2.90382455259405,2.87554618933505,51.9593739109389));
#12513=CARTESIAN_POINT('Ctrl Pts',(-2.98532230630841,2.79086082135747,51.9651160060442));
#12514=CARTESIAN_POINT('Ctrl Pts',(-3.0631239898746,2.70268318947203,51.9708581011494));
#12515=CARTESIAN_POINT('Ctrl Pts',(-3.14428289015889,2.61070060881995,51.9768479731253));
#12516=CARTESIAN_POINT('Ctrl Pts',(-3.22141920270685,2.51491785335467,51.9828378451012));
#12517=CARTESIAN_POINT('Ctrl Pts',(-3.29415604745111,2.41573196672174,51.9888277170772));
#12518=CARTESIAN_POINT('Ctrl Pts',(-3.36371623152867,2.32087785865119,51.9945559913611));
#12519=CARTESIAN_POINT('Ctrl Pts',(-3.42925281645865,2.22291197470652,52.0002842656451));
#12520=CARTESIAN_POINT('Ctrl Pts',(-3.49047521124661,2.12221766076736,52.006012539929));
#12521=CARTESIAN_POINT('Ctrl Pts',(-3.55166090817329,2.02158370490433,52.011737380577));
#12522=CARTESIAN_POINT('Ctrl Pts',(-3.60853733626655,1.91822492781679,52.0174622212251));
#12523=CARTESIAN_POINT('Ctrl Pts',(-3.66085668343508,1.81255436976349,52.0231870618731));
#12524=CARTESIAN_POINT('Ctrl Pts',(-3.71315785954413,1.70692051220625,52.0289099142237));
#12525=CARTESIAN_POINT('Ctrl Pts',(-3.76090491502834,1.5989768468548,52.0346327665744));
#12526=CARTESIAN_POINT('Ctrl Pts',(-3.80389594386372,1.48916105517743,52.0403556189251));
#12527=CARTESIAN_POINT('Ctrl Pts',(-3.84688287862381,1.37935572135907,52.0460779262832));
#12528=CARTESIAN_POINT('Ctrl Pts',(-3.88511453582612,1.26767900832715,52.0518002336414));
#12529=CARTESIAN_POINT('Ctrl Pts',(-3.91843742957534,1.15458785309,52.0575225409995));
#12530=CARTESIAN_POINT('Ctrl Pts',(-3.95177845910788,1.04143514867586,52.0632479626888));
#12531=CARTESIAN_POINT('Ctrl Pts',(-3.98020527092869,0.92686686891414,52.0689733843781));
#12532=CARTESIAN_POINT('Ctrl Pts',(-4.00361455484754,0.811354112710945,
52.0746988060675));
#12533=CARTESIAN_POINT('Ctrl Pts',(-4.02703139991122,0.695804046153278,
52.0804260770548));
#12534=CARTESIAN_POINT('Ctrl Pts',(-4.04542742176376,0.579309310973017,
52.0861533480421));
#12535=CARTESIAN_POINT('Ctrl Pts',(-4.0587508784753,0.462348684951092,52.0918806190295));
#12536=CARTESIAN_POINT('Ctrl Pts',(-4.07208789433607,0.345269029264654,
52.0976137186035));
#12537=CARTESIAN_POINT('Ctrl Pts',(-4.08034201096014,0.227722955682589,
52.1033468181775));
#12538=CARTESIAN_POINT('Ctrl Pts',(-4.08351353671633,0.110191630600995,
52.1090799177515));
#12539=CARTESIAN_POINT('Ctrl Pts',(-4.08453420312904,0.0723674774412442,
52.1109249546914));
#12540=CARTESIAN_POINT('Ctrl Pts',(-4.08502887233281,0.0345448325489773,
52.1127699916312));
#12541=CARTESIAN_POINT('Ctrl Pts',(-4.08499869890724,-0.00326035675198486,
52.1146150285711));
#12542=CARTESIAN_POINT('Ctrl Pts',(-4.08499869890684,-0.00326035725228949,
52.1146150285955));
#12543=CARTESIAN_POINT('Ctrl Pts',(-4.08485654869641,-0.181364589317125,
52.1233071921155));
#12544=CARTESIAN_POINT('Ctrl Pts',(-4.07306320787908,-0.359009021589031,
52.1319993556354));
#12545=CARTESIAN_POINT('Ctrl Pts',(-4.0498173705152,-0.534980621586747,
52.1406915191554));
#12546=CARTESIAN_POINT('Ctrl Pts',(-4.04162212857929,-0.597018818501584,
52.1437559122284));
#12547=CARTESIAN_POINT('Ctrl Pts',(-4.03200385599029,-0.658849401833403,
52.1468203053013));
#12548=CARTESIAN_POINT('Ctrl Pts',(-4.02097252192971,-0.720420001031497,
52.1498846983743));
#12549=CARTESIAN_POINT('Ctrl Pts',(-3.99999469520333,-0.83750623505584,
52.1557121265487));
#12550=CARTESIAN_POINT('Ctrl Pts',(-3.97386510412177,-0.95386180699246,
52.1615395547231));
#12551=CARTESIAN_POINT('Ctrl Pts',(-3.94264701505503,-1.06899930527464,
52.1673669828975));
#12552=CARTESIAN_POINT('Ctrl Pts',(-3.91142671509086,-1.18414495771379,
52.1731948237764));
#12553=CARTESIAN_POINT('Ctrl Pts',(-3.87511722923416,-1.29807195533858,
52.1790226646553));
#12554=CARTESIAN_POINT('Ctrl Pts',(-3.83383365485423,-1.41029943873882,
52.1848505055342));
#12555=CARTESIAN_POINT('Ctrl Pts',(-3.7926549498143,-1.52224183969914,52.1906635424182));
#12556=CARTESIAN_POINT('Ctrl Pts',(-3.7465275009288,-1.63249295561268,52.1964765793021));
#12557=CARTESIAN_POINT('Ctrl Pts',(-3.69561600635882,-1.74058821481259,
52.2022896161861));
#12558=CARTESIAN_POINT('Ctrl Pts',(-3.64473842267718,-1.84861147443174,
52.2080987811498));
#12559=CARTESIAN_POINT('Ctrl Pts',(-3.58908330420487,-1.95448136575595,
52.2139079461136));
#12560=CARTESIAN_POINT('Ctrl Pts',(-3.52886367089602,-2.05775270434283,
52.2197171110773));
#12561=CARTESIAN_POINT('Ctrl Pts',(-3.46866998087206,-2.16097955249345,
52.2255237733885));
#12562=CARTESIAN_POINT('Ctrl Pts',(-3.40391589366085,-2.26160972367424,
52.2313304356996));
#12563=CARTESIAN_POINT('Ctrl Pts',(-3.33486033893715,-2.35922265159183,
52.2371370980108));
#12564=CARTESIAN_POINT('Ctrl Pts',(-3.26539041267044,-2.45742131109496,
52.2429786035091));
#12565=CARTESIAN_POINT('Ctrl Pts',(-3.19156743003351,-2.55256603294785,
52.2488201090075));
#12566=CARTESIAN_POINT('Ctrl Pts',(-3.1136990161998,-2.6442585797377,52.2546616145059));
#12567=CARTESIAN_POINT('Ctrl Pts',(-3.03628664318898,-2.73541412387868,
52.2604689088929));
#12568=CARTESIAN_POINT('Ctrl Pts',(-2.95487639471255,-2.82315753412575,
52.26627620328));
#12569=CARTESIAN_POINT('Ctrl Pts',(-2.86981001746449,-2.90713182770586,
52.272083497667));
#12570=CARTESIAN_POINT('Ctrl Pts',(-2.78399194370129,-2.99184816750787,
52.277942108721));
#12571=CARTESIAN_POINT('Ctrl Pts',(-2.69445310243411,-3.07272814755913,
52.2838007197751));
#12572=CARTESIAN_POINT('Ctrl Pts',(-2.60158052560731,-3.14944499376966,
52.2896593308291));
#12573=CARTESIAN_POINT('Ctrl Pts',(-2.50870794878052,-3.22616183998019,
52.2955179418831));
#12574=CARTESIAN_POINT('Ctrl Pts',(-2.41250198808257,-3.2987153137835,52.3013765529371));
#12575=CARTESIAN_POINT('Ctrl Pts',(-2.31338095599003,-3.36682247118298,
52.3072351639912));
#12576=CARTESIAN_POINT('',(-4.08499847832697,0.00352591354478465,52.0103849713646));
#12577=CARTESIAN_POINT('Ctrl Pts',(-4.08499847832768,0.00352591272458481,
52.0103849714045));
#12578=CARTESIAN_POINT('Ctrl Pts',(-4.0851002980183,-0.114438799892165,
52.0161295062253));
#12579=CARTESIAN_POINT('Ctrl Pts',(-4.08008809612221,-0.232534395693748,
52.0218740410462));
#12580=CARTESIAN_POINT('Ctrl Pts',(-4.06995463095962,-0.350277464205617,
52.027618575867));
#12581=CARTESIAN_POINT('Ctrl Pts',(-4.05982760487945,-0.467945715534103,
52.0333594604525));
#12582=CARTESIAN_POINT('Ctrl Pts',(-4.04458582194297,-0.585261469241392,
52.039100345038));
#12583=CARTESIAN_POINT('Ctrl Pts',(-4.02427410712041,-0.701742766802956,
52.0448412296234));
#12584=CARTESIAN_POINT('Ctrl Pts',(-4.0039689110298,-0.818186681486533,
52.0505802717604));
#12585=CARTESIAN_POINT('Ctrl Pts',(-3.97859708867849,-0.933796260396595,
52.0563193138974));
#12586=CARTESIAN_POINT('Ctrl Pts',(-3.94825507161076,-1.04809679395555,
52.0620583560344));
#12587=CARTESIAN_POINT('Ctrl Pts',(-3.91791522923565,-1.16238913529297,
52.0677969868391));
#12588=CARTESIAN_POINT('Ctrl Pts',(-3.88260600808933,-1.27537221339099,
52.0735356176437));
#12589=CARTESIAN_POINT('Ctrl Pts',(-3.8424743059363,-1.38658436750864,52.0792742484484));
#12590=CARTESIAN_POINT('Ctrl Pts',(-3.80233547636011,-1.49781627299593,
52.0850138984386));
#12591=CARTESIAN_POINT('Ctrl Pts',(-3.75737260616839,-1.60727623597289,
52.0907535484288));
#12592=CARTESIAN_POINT('Ctrl Pts',(-3.70778125120284,-1.71452127231735,
52.096493198419));
#12593=CARTESIAN_POINT('Ctrl Pts',(-3.6581399257979,-1.82187437349674,52.102238631934));
#12594=CARTESIAN_POINT('Ctrl Pts',(-3.60386098019509,-1.92700771180435,
52.107984065449));
#12595=CARTESIAN_POINT('Ctrl Pts',(-3.54518661164281,-2.02950163553237,
52.113729498964));
#12596=CARTESIAN_POINT('Ctrl Pts',(-3.48647998938321,-2.13205190088108,
52.1194780907837));
#12597=CARTESIAN_POINT('Ctrl Pts',(-3.4233733573591,-2.23195950984396,52.1252266826033));
#12598=CARTESIAN_POINT('Ctrl Pts',(-3.35615204817023,-2.32883413526227,
52.130975274423));
#12599=CARTESIAN_POINT('Ctrl Pts',(-3.28882935454087,-2.42585486880931,
52.1367325363767));
#12600=CARTESIAN_POINT('Ctrl Pts',(-3.21737984600797,-2.51983315294746,
52.1424897983305));
#12601=CARTESIAN_POINT('Ctrl Pts',(-3.1421290247519,-2.61041188164085,52.1482470602843));
#12602=CARTESIAN_POINT('Ctrl Pts',(-3.09623099807221,-2.6656589186404,52.1517586095052));
#12603=CARTESIAN_POINT('Ctrl Pts',(-3.04891955031542,-2.71964195879564,
52.1552701587261));
#12604=CARTESIAN_POINT('Ctrl Pts',(-3.00027489997305,-2.77228705667211,
52.158781707947));
#12605=CARTESIAN_POINT('Ctrl Pts',(-2.91955433272997,-2.85964593649234,
52.1646087463371));
#12606=CARTESIAN_POINT('Ctrl Pts',(-2.8348867034544,-2.94361541160434,52.1704357847271));
#12607=CARTESIAN_POINT('Ctrl Pts',(-2.74658772409465,-3.0238189221335,52.1762628231172));
#12608=CARTESIAN_POINT('Ctrl Pts',(-2.65841192984707,-3.10391054146625,
52.1820817322583));
#12609=CARTESIAN_POINT('Ctrl Pts',(-2.56661516667542,-3.18024637993033,
52.1879006413995));
#12610=CARTESIAN_POINT('Ctrl Pts',(-2.47155169054511,-3.25248477951298,
52.1937195505407));
#12611=CARTESIAN_POINT('Ctrl Pts',(-2.41977587778372,-3.29182903666856,
52.1968887882168));
#12612=CARTESIAN_POINT('Ctrl Pts',(-2.36703170632116,-3.32995844726935,
52.2000580258928));
#12613=CARTESIAN_POINT('Ctrl Pts',(-2.31338095599002,-3.36682247118298,
52.2032272635689));
#12614=CARTESIAN_POINT('Ctrl Pts',(-2.31338095599002,-3.36682247118298,
50.953013989131));
#12615=CARTESIAN_POINT('Ctrl Pts',(-2.21503604400629,-3.43439634787205,
50.9588336971937));
#12616=CARTESIAN_POINT('Ctrl Pts',(-2.11384052331764,-3.49758034904679,
50.9646534052564));
#12617=CARTESIAN_POINT('Ctrl Pts',(-2.01023163741533,-3.55614872635193,
50.9704731133191));
#12618=CARTESIAN_POINT('Ctrl Pts',(-1.94619208453836,-3.59234921883563,
50.9740702131138));
#12619=CARTESIAN_POINT('Ctrl Pts',(-1.88123099978353,-3.62678730989976,
50.9776673129085));
#12620=CARTESIAN_POINT('Ctrl Pts',(-1.81545530512256,-3.65941894774326,
50.9812644127032));
#12621=CARTESIAN_POINT('Ctrl Pts',(-1.70889026982991,-3.71228637326225,
50.9870921742882));
#12622=CARTESIAN_POINT('Ctrl Pts',(-1.59984484477099,-3.76057898376045,
50.9929199358733));
#12623=CARTESIAN_POINT('Ctrl Pts',(-1.4887483140663,-3.80405749921906,50.9987476974583));
#12624=CARTESIAN_POINT('Ctrl Pts',(-1.37779067366811,-3.84748165884585,
51.0045681733109));
#12625=CARTESIAN_POINT('Ctrl Pts',(-1.26478740440378,-3.88610354726307,
51.0103886491636));
#12626=CARTESIAN_POINT('Ctrl Pts',(-1.15019154773323,-3.91973014422205,
51.0162091250162));
#12627=CARTESIAN_POINT('Ctrl Pts',(-1.03570921813449,-3.95332342820447,
51.022023834678));
#12628=CARTESIAN_POINT('Ctrl Pts',(-0.919637828923187,-3.98193115185382,
51.0278385443398));
#12629=CARTESIAN_POINT('Ctrl Pts',(-0.802448969845905,-4.00540892429141,
51.0336532540016));
#12630=CARTESIAN_POINT('Ctrl Pts',(-0.681639965355161,-4.02961196149287,
51.0396475890533));
#12631=CARTESIAN_POINT('Ctrl Pts',(-0.559643739567971,-4.04836279438894,
51.0456419241051));
#12632=CARTESIAN_POINT('Ctrl Pts',(-0.436992659478849,-4.06155911142034,
51.0516362591569));
#12633=CARTESIAN_POINT('Ctrl Pts',(-0.318148572653272,-4.07434582512819,
51.0574445347533));
#12634=CARTESIAN_POINT('Ctrl Pts',(-0.198690117475006,-4.08191769342196,
51.0632528103496));
#12635=CARTESIAN_POINT('Ctrl Pts',(-0.0791097938878756,-4.08423391109165,
51.069061085946));
#12636=CARTESIAN_POINT('Ctrl Pts',(0.0404533604251056,-4.08654979620014,
51.0748685275936));
#12637=CARTESIAN_POINT('Ctrl Pts',(0.160137940902236,-4.08361152357275,
51.0806759692411));
#12638=CARTESIAN_POINT('Ctrl Pts',(0.279449736580199,-4.0754303876677,51.0864834108886));
#12639=CARTESIAN_POINT('Ctrl Pts',(0.398772437464804,-4.06724850399937,
51.0922913833416));
#12640=CARTESIAN_POINT('Ctrl Pts',(0.517721879117753,-4.05382283216858,
51.0980993557946));
#12641=CARTESIAN_POINT('Ctrl Pts',(0.635807899724545,-4.03521663788301,
51.1039073282475));
#12642=CARTESIAN_POINT('Ctrl Pts',(0.753932461133397,-4.0166043709256,51.109717196301));
#12643=CARTESIAN_POINT('Ctrl Pts',(0.871192638594963,-3.99280828218478,
51.1155270643544));
#12644=CARTESIAN_POINT('Ctrl Pts',(0.987108027432526,-3.96394282781403,
51.1213369324079));
#12645=CARTESIAN_POINT('Ctrl Pts',(1.10315050066471,-3.93504572666341,51.1271531701381));
#12646=CARTESIAN_POINT('Ctrl Pts',(1.21784484664755,-3.90106826487509,51.1329694078684));
#12647=CARTESIAN_POINT('Ctrl Pts',(1.33072525776886,-3.86217494274094,51.1387856455987));
#12648=CARTESIAN_POINT('Ctrl Pts',(1.44367986835026,-3.82325605493535,51.1446057065051));
#12649=CARTESIAN_POINT('Ctrl Pts',(1.55481779108012,-3.77941502048066,51.1504257674115));
#12650=CARTESIAN_POINT('Ctrl Pts',(1.66369416928531,-3.7308640703041,51.156245828318));
#12651=CARTESIAN_POINT('Ctrl Pts',(1.77272339024437,-3.68224496336984,51.1620740595379));
#12652=CARTESIAN_POINT('Ctrl Pts',(1.87948436703941,-3.62890292608085,51.1679022907578));
#12653=CARTESIAN_POINT('Ctrl Pts',(1.98355765725178,-3.57109563304566,51.1737305219776));
#12654=CARTESIAN_POINT('Ctrl Pts',(2.00609748327204,-3.55857593346611,51.1749927797331));
#12655=CARTESIAN_POINT('Ctrl Pts',(2.02851135483631,-3.54584694786113,51.1762550374885));
#12656=CARTESIAN_POINT('Ctrl Pts',(2.05079520308251,-3.53291155210738,51.1775172952439));
#12657=CARTESIAN_POINT('Ctrl Pts',(2.15367449828829,-3.47319186708479,51.1833448429282));
#12658=CARTESIAN_POINT('Ctrl Pts',(2.25410615705943,-3.40887996998109,51.1891723906125));
#12659=CARTESIAN_POINT('Ctrl Pts',(2.3516538373978,-3.34020197429021,51.1949999382969));
#12660=CARTESIAN_POINT('Ctrl Pts',(2.44907980244682,-3.27160967168898,51.2008202146483));
#12661=CARTESIAN_POINT('Ctrl Pts',(2.54362861620005,-3.19866233919883,51.2066404909998));
#12662=CARTESIAN_POINT('Ctrl Pts',(2.63488942346093,-3.12163142060906,51.2124607673513));
#12663=CARTESIAN_POINT('Ctrl Pts',(2.72606004679311,-3.04467662397217,51.2182752921058));
#12664=CARTESIAN_POINT('Ctrl Pts',(2.81394881802279,-2.96364653099269,51.2240898168602));
#12665=CARTESIAN_POINT('Ctrl Pts',(2.8981752184825,-2.87885487702557,51.2299043416147));
#12666=CARTESIAN_POINT('Ctrl Pts',(2.98500734751445,-2.79144000712824,51.2358987514551));
#12667=CARTESIAN_POINT('Ctrl Pts',(3.06794645219371,-2.70002730027494,51.2418931612955));
#12668=CARTESIAN_POINT('Ctrl Pts',(3.146613551979,-2.60500444423846,51.2478875711359));
#12669=CARTESIAN_POINT('Ctrl Pts',(3.22283600547571,-2.51293450337202,51.2536956996489));
#12670=CARTESIAN_POINT('Ctrl Pts',(3.2950477569999,-2.41747580536904,51.259503828162));
#12671=CARTESIAN_POINT('Ctrl Pts',(3.36294316667186,-2.31901665749409,51.265311956675));
#12672=CARTESIAN_POINT('Ctrl Pts',(3.43082899567965,-2.2205714031067,51.2711192656079));
#12673=CARTESIAN_POINT('Ctrl Pts',(3.49439946281028,-2.11912687641255,51.2769265745408));
#12674=CARTESIAN_POINT('Ctrl Pts',(3.55339144620601,-2.01510154335457,51.2827338834737));
#12675=CARTESIAN_POINT('Ctrl Pts',(3.61238896987661,-1.91106644068205,51.2885417378043));
#12676=CARTESIAN_POINT('Ctrl Pts',(3.66680695376404,-1.80445040434974,51.2943495921348));
#12677=CARTESIAN_POINT('Ctrl Pts',(3.71642786354686,-1.69569718259261,51.3001574464653));
#12678=CARTESIAN_POINT('Ctrl Pts',(3.76606509555665,-1.58690818771532,51.3059672112227));
#12679=CARTESIAN_POINT('Ctrl Pts',(3.81090194606285,-1.47598097993228,51.31177697598));
#12680=CARTESIAN_POINT('Ctrl Pts',(3.85076896470228,-1.36337939711797,51.3175867407374));
#12681=CARTESIAN_POINT('Ctrl Pts',(3.89067984733628,-1.25065392354416,51.3234028977332));
#12682=CARTESIAN_POINT('Ctrl Pts',(3.92560984752966,-1.13625078225909,51.329219054729));
#12683=CARTESIAN_POINT('Ctrl Pts',(3.9554393111504,-1.02064923250156,51.3350352117248));
#12684=CARTESIAN_POINT('Ctrl Pts',(3.98528845015726,-0.90497143245822,51.3408552050328));
#12685=CARTESIAN_POINT('Ctrl Pts',(4.0100302680747,-0.78809404753574,51.3466751983408));
#12686=CARTESIAN_POINT('Ctrl Pts',(4.02959648159546,-0.670505179333855,
51.3524951916488));
#12687=CARTESIAN_POINT('Ctrl Pts',(4.04919022894369,-0.552750838563258,
51.3583233749262));
#12688=CARTESIAN_POINT('Ctrl Pts',(4.06359378695451,-0.434283419442727,
51.3641515582037));
#12689=CARTESIAN_POINT('Ctrl Pts',(4.07279079626367,-0.315594882515428,
51.3699797414812));
#12690=CARTESIAN_POINT('Ctrl Pts',(4.07478459526346,-0.289864661064443,
51.371243220249));
#12691=CARTESIAN_POINT('Ctrl Pts',(4.07653389700963,-0.264124041270327,
51.3725066990167));
#12692=CARTESIAN_POINT('Ctrl Pts',(4.07803885719302,-0.238378017492929,
51.3737701777845));
#12693=CARTESIAN_POINT('Ctrl Pts',(4.08497817797847,-0.119663967836718,
51.379596035885));
#12694=CARTESIAN_POINT('Ctrl Pts',(4.08674052243847,-0.000457205424181928,
51.3854218939854));
#12695=CARTESIAN_POINT('Ctrl Pts',(4.08327350447201,0.118753895417587,51.3912477520858));
#12696=CARTESIAN_POINT('Ctrl Pts',(4.07981083073444,0.237815622845764,51.397066310293));
#12697=CARTESIAN_POINT('Ctrl Pts',(4.07113183939052,0.356881273646933,51.4028848685002));
#12698=CARTESIAN_POINT('Ctrl Pts',(4.05723600945606,0.475458687556647,51.4087034267074));
#12699=CARTESIAN_POINT('Ctrl Pts',(4.0433539781617,0.593918353403358,51.4145162070523));
#12700=CARTESIAN_POINT('Ctrl Pts',(4.02426546143581,0.711890343989486,51.4203289873973));
#12701=CARTESIAN_POINT('Ctrl Pts',(4.00002194848,0.828884438072178,51.4261417677423));
#12702=CARTESIAN_POINT('Ctrl Pts',(3.97501822268229,0.94954715942479,51.4321368215999));
#12703=CARTESIAN_POINT('Ctrl Pts',(3.94453089160701,1.06916920351069,51.4381318754575));
#12704=CARTESIAN_POINT('Ctrl Pts',(3.90867410516127,1.18722017319524,51.4441269293152));
#12705=CARTESIAN_POINT('Ctrl Pts',(3.87394608817749,1.30155490551603,51.449933259241));
#12706=CARTESIAN_POINT('Ctrl Pts',(3.83418173070917,1.41441557471631,51.4557395891669));
#12707=CARTESIAN_POINT('Ctrl Pts',(3.78953605866919,1.52533322918174,51.4615459190928));
#12708=CARTESIAN_POINT('Ctrl Pts',(3.74489681890927,1.63623490329824,51.4673514124776));
#12709=CARTESIAN_POINT('Ctrl Pts',(3.69537781552154,1.74519374108193,51.4731569058624));
#12710=CARTESIAN_POINT('Ctrl Pts',(3.64118269125795,1.85175959802657,51.4789623992472));
#12711=CARTESIAN_POINT('Ctrl Pts',(3.58698261568811,1.95833519090596,51.4847684230261));
#12712=CARTESIAN_POINT('Ctrl Pts',(3.52810575477887,2.06251700463936,51.490574446805));
#12713=CARTESIAN_POINT('Ctrl Pts',(3.46480199459916,2.1638789564626,51.4963804705839));
#12714=CARTESIAN_POINT('Ctrl Pts',(3.40147754716054,2.26527403271534,51.5021883917338));
#12715=CARTESIAN_POINT('Ctrl Pts',(3.33372353927051,2.36384706853591,51.5079963128836));
#12716=CARTESIAN_POINT('Ctrl Pts',(3.26183314596471,2.45920099379574,51.5138042340335));
#12717=CARTESIAN_POINT('Ctrl Pts',(3.18986375518712,2.55465969966219,51.5196185372752));
#12718=CARTESIAN_POINT('Ctrl Pts',(3.11374915219426,2.64689190844894,51.5254328405168));
#12719=CARTESIAN_POINT('Ctrl Pts',(3.0338228506004,2.73553356974007,51.5312471437584));
#12720=CARTESIAN_POINT('Ctrl Pts',(2.95384392377078,2.82423359465157,51.5370652752653));
#12721=CARTESIAN_POINT('Ctrl Pts',(2.87004858564418,2.90933807383332,51.5428834067721));
#12722=CARTESIAN_POINT('Ctrl Pts',(2.78280606796309,2.99052092253303,51.548701538279));
#12723=CARTESIAN_POINT('Ctrl Pts',(2.69544070968695,3.07181807959645,51.5545278619237));
#12724=CARTESIAN_POINT('Ctrl Pts',(2.60461879405326,3.14918232216273,51.5603541855685));
#12725=CARTESIAN_POINT('Ctrl Pts',(2.5107414184921,3.22232874323342,51.5661805092132));
#12726=CARTESIAN_POINT('Ctrl Pts',(2.49010355513011,3.23840914422942,51.5674613595839));
#12727=CARTESIAN_POINT('Ctrl Pts',(2.46931812920197,3.25428587253981,51.5687422099545));
#12728=CARTESIAN_POINT('Ctrl Pts',(2.44838957246161,3.26995619259055,51.5700230603252));
#12729=CARTESIAN_POINT('Ctrl Pts',(2.35318136683388,3.34124362402462,51.575849905768));
#12730=CARTESIAN_POINT('Ctrl Pts',(2.25470573000445,3.40848286671879,51.5816767512108));
#12731=CARTESIAN_POINT('Ctrl Pts',(2.15334133041396,3.47136084478854,51.5875035966536));
#12732=CARTESIAN_POINT('Ctrl Pts',(2.05210370916048,3.53416018020341,51.5933231543526));
#12733=CARTESIAN_POINT('Ctrl Pts',(1.94798485517365,3.59260888757542,51.5991427120516));
#12734=CARTESIAN_POINT('Ctrl Pts',(1.84139519027646,3.64643507459364,51.6049622697506));
#12735=CARTESIAN_POINT('Ctrl Pts',(1.73491115290288,3.7002079212918,51.6107760604227));
#12736=CARTESIAN_POINT('Ctrl Pts',(1.62596153775807,3.74936717810325,51.6165898510948));
#12737=CARTESIAN_POINT('Ctrl Pts',(1.51498382552037,3.79368541242044,51.6224036417669));
#12738=CARTESIAN_POINT('Ctrl Pts',(1.4005531860078,3.83938255099654,51.6283983209793));
#12739=CARTESIAN_POINT('Ctrl Pts',(1.28396655721288,3.87993226317693,51.6343930001918));
#12740=CARTESIAN_POINT('Ctrl Pts',(1.1657291361518,3.91513736427303,51.6403876794042));
#12741=CARTESIAN_POINT('Ctrl Pts',(1.0511863349633,3.94924239514637,51.6461950400778));
#12742=CARTESIAN_POINT('Ctrl Pts',(0.935094790972726,3.97833172795182,51.6520024007515));
#12743=CARTESIAN_POINT('Ctrl Pts',(0.817931329882171,4.00227601991632,51.6578097614251));
#12744=CARTESIAN_POINT('Ctrl Pts',(0.700784629779372,4.02621688649563,51.6636162913184));
#12745=CARTESIAN_POINT('Ctrl Pts',(0.582566716966366,4.04501409443355,51.6694228212117));
#12746=CARTESIAN_POINT('Ctrl Pts',(0.463765540101661,4.05858922826815,51.6752293511049));
#12747=CARTESIAN_POINT('Ctrl Pts',(0.344953416769791,4.07216561293005,51.6810364160181));
#12748=CARTESIAN_POINT('Ctrl Pts',(0.225558327689244,4.08051892051422,51.6868434809312));
#12749=CARTESIAN_POINT('Ctrl Pts',(0.106073654365429,4.08362258048532,51.6926505458443));
#12750=CARTESIAN_POINT('Ctrl Pts',(-0.0134501306549043,4.08672725639765,
51.6984595116219));
#12751=CARTESIAN_POINT('Ctrl Pts',(-0.133063150818387,4.08457885652801,
51.7042684773994));
#12752=CARTESIAN_POINT('Ctrl Pts',(-0.252272348793747,4.07720292137074,
51.7100774431769));
#12753=CARTESIAN_POINT('Ctrl Pts',(-0.371612516373126,4.0698188826164,51.7158927909951));
#12754=CARTESIAN_POINT('Ctrl Pts',(-0.490547568998258,4.05719587012279,
51.7217081388133));
#12755=CARTESIAN_POINT('Ctrl Pts',(-0.608589741591365,4.03941128463415,
51.7275234866315));
#12756=CARTESIAN_POINT('Ctrl Pts',(-0.726709645230837,4.02161498795444,
51.7333426638698));
#12757=CARTESIAN_POINT('Ctrl Pts',(-0.843935098636929,3.9986504272913,51.7391618411081));
#12758=CARTESIAN_POINT('Ctrl Pts',(-0.959790300434298,3.97064573831414,
51.7449810183464));
#12759=CARTESIAN_POINT('Ctrl Pts',(-1.0758084792732,3.94260165428792,51.7508083815985));
#12760=CARTESIAN_POINT('Ctrl Pts',(-1.19045216910166,3.90950340407007,51.7566357448507));
#12761=CARTESIAN_POINT('Ctrl Pts',(-1.30326233582066,3.87152841705072,51.7624631081029));
#12762=CARTESIAN_POINT('Ctrl Pts',(-1.32786617502205,3.86324609196006,51.7637340530239));
#12763=CARTESIAN_POINT('Ctrl Pts',(-1.35238288136288,3.85473197179528,51.7650049979448));
#12764=CARTESIAN_POINT('Ctrl Pts',(-1.37680783803398,3.84598819253624,51.7662759428658));
#12765=CARTESIAN_POINT('Ctrl Pts',(-1.48878552586352,3.80590180886304,51.7721026665536));
#12766=CARTESIAN_POINT('Ctrl Pts',(-1.59918920479397,3.7608571761825,51.7779293902414));
#12767=CARTESIAN_POINT('Ctrl Pts',(-1.707548870435,3.71099742051597,51.7837561139291));
#12768=CARTESIAN_POINT('Ctrl Pts',(-1.81577301396521,3.66120002291683,51.7895755503123));
#12769=CARTESIAN_POINT('Ctrl Pts',(-1.92195786169754,3.60659964961025,51.7953949866954));
#12770=CARTESIAN_POINT('Ctrl Pts',(-2.02565024277944,3.547388630236,51.8012144230786));
#12771=CARTESIAN_POINT('Ctrl Pts',(-2.12923987585959,3.48823628261619,51.8070280930259));
#12772=CARTESIAN_POINT('Ctrl Pts',(-2.23034160361061,3.42448257910419,51.8128417629732));
#12773=CARTESIAN_POINT('Ctrl Pts',(-2.32852441122453,3.35636694452967,51.8186554329206));
#12774=CARTESIAN_POINT('Ctrl Pts',(-2.42976491953772,3.28612998924197,51.8246501576075));
#12775=CARTESIAN_POINT('Ctrl Pts',(-2.52790132295908,3.2112551532176,51.8306448822944));
#12776=CARTESIAN_POINT('Ctrl Pts',(-2.62249044523785,3.13205505453467,51.8366396069813));
#12777=CARTESIAN_POINT('Ctrl Pts',(-2.71412133320897,3.05533190503415,51.8424468492198));
#12778=CARTESIAN_POINT('Ctrl Pts',(-2.80242317725726,2.97455028346731,51.8482540914584));
#12779=CARTESIAN_POINT('Ctrl Pts',(-2.8870250743218,2.8900365430626,51.8540613336969));
#12780=CARTESIAN_POINT('Ctrl Pts',(-2.97161488383443,2.80553487761435,51.8598677462219));
#12781=CARTESIAN_POINT('Ctrl Pts',(-3.05250550927932,2.71730244194935,51.8656741587469));
#12782=CARTESIAN_POINT('Ctrl Pts',(-3.12936238979499,2.62570295984459,51.8714805712719));
#12783=CARTESIAN_POINT('Ctrl Pts',(-3.20622636807049,2.53409501849557,51.8772875200211));
#12784=CARTESIAN_POINT('Ctrl Pts',(-3.27905559863151,2.43911972487573,51.8830944687703));
#12785=CARTESIAN_POINT('Ctrl Pts',(-3.34755576718379,2.34117393322122,51.8889014175195));
#12786=CARTESIAN_POINT('Ctrl Pts',(-3.41607837463245,2.24319605704027,51.894710268476));
#12787=CARTESIAN_POINT('Ctrl Pts',(-3.48026886616441,2.14224608158912,51.9005191194325));
#12788=CARTESIAN_POINT('Ctrl Pts',(-3.53987657185992,2.03874933623466,51.906327970389));
#12789=CARTESIAN_POINT('Ctrl Pts',(-3.59954979347561,1.93513883571334,51.9121432059599));
#12790=CARTESIAN_POINT('Ctrl Pts',(-3.65462997162388,1.82897633158772,51.9179584415308));
#12791=CARTESIAN_POINT('Ctrl Pts',(-3.70491261208295,1.72071134616725,51.9237736771017));
#12792=CARTESIAN_POINT('Ctrl Pts',(-3.75522837636329,1.61237504090371,51.9295927434743));
#12793=CARTESIAN_POINT('Ctrl Pts',(-3.80074015378899,1.50193387212695,51.9354118098469));
#12794=CARTESIAN_POINT('Ctrl Pts',(-3.8412923675263,1.38985536916046,51.9412308762195));
#12795=CARTESIAN_POINT('Ctrl Pts',(-3.88190164819559,1.27761914419275,51.9470581314487));
#12796=CARTESIAN_POINT('Ctrl Pts',(-3.91753731438086,1.16374137413654,51.9528853866779));
#12797=CARTESIAN_POINT('Ctrl Pts',(-3.94809415420144,1.04870279372205,51.9587126419072));
#12798=CARTESIAN_POINT('Ctrl Pts',(-3.95476456209936,1.02359043721307,51.9599847030736));
#12799=CARTESIAN_POINT('Ctrl Pts',(-3.96119314504871,0.998422794177258,
51.96125676424));
#12800=CARTESIAN_POINT('Ctrl Pts',(-3.96737913600756,0.973204907083755,
51.9625288254064));
#12801=CARTESIAN_POINT('Ctrl Pts',(-4.00616627586605,0.815084774006025,
51.9705048497328));
#12802=CARTESIAN_POINT('Ctrl Pts',(-4.03551488037941,0.654566284093707,
51.9784808740591));
#12803=CARTESIAN_POINT('Ctrl Pts',(-4.05518763375965,0.492623847375249,
51.9864568983855));
#12804=CARTESIAN_POINT('Ctrl Pts',(-4.07361578512735,0.340926742296961,
51.9939283173962));
#12805=CARTESIAN_POINT('Ctrl Pts',(-4.08355402542618,0.187980020910348,
52.001399736407));
#12806=CARTESIAN_POINT('Ctrl Pts',(-4.08485340672103,0.0346070166231305,
52.0088711554177));
#12807=CARTESIAN_POINT('Ctrl Pts',(-4.08494116444249,0.0242484979634525,
52.0093757607333));
#12808=CARTESIAN_POINT('Ctrl Pts',(-4.08498953438796,0.0138880443175454,
52.0098803660489));
#12809=CARTESIAN_POINT('Ctrl Pts',(-4.08499847832697,0.00352591354478465,
52.0103849713646));
#12810=CARTESIAN_POINT('Ctrl Pts',(-3.3742051597689,0.272260201830434,50.0026433987789));
#12811=CARTESIAN_POINT('Ctrl Pts',(-3.46373108274233,-0.837262340205114,
50.0680610262924));
#12812=CARTESIAN_POINT('Ctrl Pts',(-2.46188142412267,-3.13325453455775,
50.1988962813195));
#12813=CARTESIAN_POINT('Ctrl Pts',(1.26137334667247,-3.78380856561343,50.3951491638602));
#12814=CARTESIAN_POINT('Ctrl Pts',(3.84893150453541,-1.03415529302938,50.5914020464008));
#12815=CARTESIAN_POINT('Ctrl Pts',(2.98722390906374,2.63934847059358,50.7876549289415));
#12816=CARTESIAN_POINT('Ctrl Pts',(-0.554316335019722,3.94781660436653,
50.9839078114821));
#12817=CARTESIAN_POINT('Ctrl Pts',(-3.59823642187141,1.71527100232214,51.1801606940228));
#12818=CARTESIAN_POINT('Ctrl Pts',(-3.41577519450092,-2.0549734213795,51.3764135765633));
#12819=CARTESIAN_POINT('Ctrl Pts',(-0.170140265370355,-3.98267722262975,
51.5726664591041));
#12820=CARTESIAN_POINT('Ctrl Pts',(3.22799613435637,-2.3388745938823,51.7689193416447));
#12821=CARTESIAN_POINT('Ctrl Pts',(3.73151821384908,1.40221729238016,51.9651722241853));
#12822=CARTESIAN_POINT('Ctrl Pts',(0.888849611894781,3.88592324617839,52.161425106726));
#12823=CARTESIAN_POINT('Ctrl Pts',(-2.75087059625197,2.88498188108543,52.3576779892666));
#12824=CARTESIAN_POINT('Ctrl Pts',(-3.92380027550394,-0.703009314092971,
52.5539308718072));
#12825=CARTESIAN_POINT('Ctrl Pts',(-1.57812882528071,-3.6605927578834,52.7501837543479));
#12826=CARTESIAN_POINT('Ctrl Pts',(2.18270082891269,-3.33560221219144,52.9464366368885));
#12827=CARTESIAN_POINT('Ctrl Pts',(3.98623241350175,-0.0194698709056399,
53.1426895194292));
#12828=CARTESIAN_POINT('Ctrl Pts',(2.21517984862058,3.31412217551562,53.3389424019698));
#12829=CARTESIAN_POINT('Ctrl Pts',(-1.54229618557997,3.67583317214676,53.5351952845106));
#12830=CARTESIAN_POINT('Ctrl Pts',(-3.91674528364537,0.741305469766164,
53.731448167051));
#12831=CARTESIAN_POINT('Ctrl Pts',(-2.77892183456758,-2.8579749427365,53.9277010495919));
#12832=CARTESIAN_POINT('Ctrl Pts',(0.850850924385935,-3.8944165145412,54.1239539321323));
#12833=CARTESIAN_POINT('Ctrl Pts',(3.71763807573328,-1.43860851900921,54.3202068146731));
#12834=CARTESIAN_POINT('Ctrl Pts',(3.25069860030425,2.30724639538179,54.5164596972136));
#12835=CARTESIAN_POINT('Ctrl Pts',(-0.131247725255445,3.98411864144676,
54.7127125797544));
#12836=CARTESIAN_POINT('Ctrl Pts',(-3.39549996047873,2.08830250185008,54.9089654622949));
#12837=CARTESIAN_POINT('Ctrl Pts',(-3.61489726723329,-1.68016221397994,
55.1052183448357));
#12838=CARTESIAN_POINT('Ctrl Pts',(-0.592698966878081,-3.94197098576313,
55.3014712273762));
#12839=CARTESIAN_POINT('Ctrl Pts',(2.96099171844794,-2.66888654013749,55.4977241099169));
#12840=CARTESIAN_POINT('Ctrl Pts',(3.85946510628054,0.997475016183975,55.6939769924575));
#12841=CARTESIAN_POINT('Ctrl Pts',(1.297030976099,3.76936837760147,55.8902298749982));
#12842=CARTESIAN_POINT('Ctrl Pts',(-2.42849289597393,3.16114687847811,56.0864827575388));
#12843=CARTESIAN_POINT('Ctrl Pts',(-3.97630842629188,-0.281777542149775,
56.2827356400795));
#12844=CARTESIAN_POINT('Ctrl Pts',(-1.95843925820106,-3.47202289852517,
56.4789885226201));
#12845=CARTESIAN_POINT('Ctrl Pts',(1.81562593482226,-3.54879273574328,56.6752414051608));
#12846=CARTESIAN_POINT('Ctrl Pts',(3.9615604099093,-0.443245024956087,56.8714942877014));
#12847=CARTESIAN_POINT('Ctrl Pts',(2.5550353209114,3.05977483891776,57.067747170242));
#12848=CARTESIAN_POINT('Ctrl Pts',(-1.14267304857574,3.81899544833241,57.2640000527827));
#12849=CARTESIAN_POINT('Ctrl Pts',(-3.81570893955738,1.15359885362914,57.4602529353233));
#12850=CARTESIAN_POINT('Ctrl Pts',(-3.06707588158816,-2.54626696652778,
57.656505817864));
#12851=CARTESIAN_POINT('Ctrl Pts',(0.431905572125819,-3.962813176837,57.8527587004047));
#12852=CARTESIAN_POINT('Ctrl Pts',(3.54357932256467,-1.82577519870519,58.0490115829453));
#12853=CARTESIAN_POINT('Ctrl Pts',(3.47761850079261,1.94849240971066,58.2452644654859));
#12854=CARTESIAN_POINT('Ctrl Pts',(0.293148588013416,3.97548807326636,58.4415173480266));
#12855=CARTESIAN_POINT('Ctrl Pts',(-3.15416563634503,2.43752590710906,58.6377702305672));
#12856=CARTESIAN_POINT('Ctrl Pts',(-3.77310016312419,-1.28622732383755,
58.8340231131078));
#12857=CARTESIAN_POINT('Ctrl Pts',(-1.00844788781245,-3.85661364405493,
59.0302759956485));
#12858=CARTESIAN_POINT('Ctrl Pts',(2.6602618623872,-2.96857992693771,59.2265288781891));
#12859=CARTESIAN_POINT('Ctrl Pts',(3.94392822706054,0.581336976956441,59.4227817607298));
#12860=CARTESIAN_POINT('Ctrl Pts',(1.68994917986025,3.61022697369519,59.6190346432704));
#12861=CARTESIAN_POINT('Ctrl Pts',(-2.07747158823233,3.40115608239218,59.8152875258111));
#12862=CARTESIAN_POINT('Ctrl Pts',(-3.98594307013179,0.143275338329916,
60.0115404083517));
#12863=CARTESIAN_POINT('Ctrl Pts',(-2.3119444938318,-3.24546711309908,60.2077932908924));
#12864=CARTESIAN_POINT('Ctrl Pts',(0.17337489301873,-3.55926711365582,60.3386285459194));
#12865=CARTESIAN_POINT('Ctrl Pts',(1.21263345687891,-3.16052308597322,60.404046173433));
#12866=CARTESIAN_POINT('Ctrl Pts',(-3.60785736139254,0.291113292428083,
49.8673058081045));
#12867=CARTESIAN_POINT('Ctrl Pts',(-3.70358264925775,-0.895239902286395,
49.932723435618));
#12868=CARTESIAN_POINT('Ctrl Pts',(-2.63235831798232,-3.3502217270022,50.0635586906451));
#12869=CARTESIAN_POINT('Ctrl Pts',(1.34871914977698,-4.04582440638657,50.2598115731858));
#12870=CARTESIAN_POINT('Ctrl Pts',(4.11545688676643,-1.10576702070916,50.4560644557264));
#12871=CARTESIAN_POINT('Ctrl Pts',(3.19407897864206,2.82211435227708,50.652317338267));
#12872=CARTESIAN_POINT('Ctrl Pts',(-0.592700851058509,4.2211894425729,50.8485702208078));
#12873=CARTESIAN_POINT('Ctrl Pts',(-3.84740202447223,1.83404767033637,51.0448231033483));
#12874=CARTESIAN_POINT('Ctrl Pts',(-3.65230597928024,-2.19727332356336,
51.241075985889));
#12875=CARTESIAN_POINT('Ctrl Pts',(-0.181921898586555,-4.25846403977975,
51.4373288684296));
#12876=CARTESIAN_POINT('Ctrl Pts',(3.45152385952784,-2.50083368418836,51.6335817509703));
#12877=CARTESIAN_POINT('Ctrl Pts',(3.98991312606725,1.49931605846165,51.829834633511));
#12878=CARTESIAN_POINT('Ctrl Pts',(0.950399416633318,4.15501018038018,52.0260875160515));
#12879=CARTESIAN_POINT('Ctrl Pts',(-2.94135900485841,3.08475703886098,52.2223403985922));
#12880=CARTESIAN_POINT('Ctrl Pts',(-4.19551006482977,-0.751690311904906,
52.4185932811329));
#12881=CARTESIAN_POINT('Ctrl Pts',(-1.68740886517545,-3.91407632412441,
52.6148461636735));
#12882=CARTESIAN_POINT('Ctrl Pts',(2.33384541853099,-3.56658129132739,52.8110990462142));
#12883=CARTESIAN_POINT('Ctrl Pts',(4.2622654154968,-0.020818093075613,53.0073519287548));
#12884=CARTESIAN_POINT('Ctrl Pts',(2.36857349960355,3.54361383535649,53.2036048112954));
#12885=CARTESIAN_POINT('Ctrl Pts',(-1.64909493736103,3.93037208510725,53.399857693836));
#12886=CARTESIAN_POINT('Ctrl Pts',(-4.18796653884179,0.792638345772549,
53.5961105763767));
#12887=CARTESIAN_POINT('Ctrl Pts',(-2.97135269577556,-3.05587996212226,
53.7923634589173));
#12888=CARTESIAN_POINT('Ctrl Pts',(0.909769449586076,-4.16409157861594,
53.988616341458));
#12889=CARTESIAN_POINT('Ctrl Pts',(3.97507183571676,-1.53822725344444,54.1848692239986));
#12890=CARTESIAN_POINT('Ctrl Pts',(3.47579839382954,2.46701534079058,54.3811221065393));
#12891=CARTESIAN_POINT('Ctrl Pts',(-0.140336182688226,4.26000527193475,
54.5773749890799));
#12892=CARTESIAN_POINT('Ctrl Pts',(-3.63062675443846,2.23291032920782,54.7736278716206));
#12893=CARTESIAN_POINT('Ctrl Pts',(-3.86521657656367,-1.79650771811881,
54.9698807541612));
#12894=CARTESIAN_POINT('Ctrl Pts',(-0.633741349292258,-4.21493903481416,
55.1661336367019));
#12895=CARTESIAN_POINT('Ctrl Pts',(3.16603029827518,-2.85369783241513,55.3623865192425));
#12896=CARTESIAN_POINT('Ctrl Pts',(4.12671990451392,1.06654675976815,55.5586394017832));
#12897=CARTESIAN_POINT('Ctrl Pts',(1.38684594845247,4.03038428459433,55.7548922843238));
#12898=CARTESIAN_POINT('Ctrl Pts',(-2.59665774811071,3.38004552062906,55.9511451668644));
#12899=CARTESIAN_POINT('Ctrl Pts',(-4.25165422601242,-0.301289676111394,
56.147398049405));
#12900=CARTESIAN_POINT('Ctrl Pts',(-2.09405449875632,-3.71244864500931,
56.3436509319458));
#12901=CARTESIAN_POINT('Ctrl Pts',(1.9413518397122,-3.79453453167758,56.5399038144863));
#12902=CARTESIAN_POINT('Ctrl Pts',(4.23588495978454,-0.473938231514639,
56.736156697027));
#12903=CARTESIAN_POINT('Ctrl Pts',(2.73196280447852,3.27165381299732,56.9324095795677));
#12904=CARTESIAN_POINT('Ctrl Pts',(-1.22179926079279,4.08344786075023,57.1286624621083));
#12905=CARTESIAN_POINT('Ctrl Pts',(-4.07993377244917,1.23348164059026,57.3249153446489));
#12906=CARTESIAN_POINT('Ctrl Pts',(-3.27946042797683,-2.72258727145301,
57.5211682271896));
#12907=CARTESIAN_POINT('Ctrl Pts',(0.461813560242235,-4.2372244765502,57.7174211097302));
#12908=CARTESIAN_POINT('Ctrl Pts',(3.78896010741355,-1.95220390551107,57.9136739922709));
#12909=CARTESIAN_POINT('Ctrl Pts',(3.71843172365335,2.08341886492568,58.1099268748115));
#12910=CARTESIAN_POINT('Ctrl Pts',(0.313448128127004,4.25077706633721,58.3061797573521));
#12911=CARTESIAN_POINT('Ctrl Pts',(-3.37258085128358,2.60631626446532,58.5024326398928));
#12912=CARTESIAN_POINT('Ctrl Pts',(-4.03437448353951,-1.37529418011125,
58.6986855224334));
#12913=CARTESIAN_POINT('Ctrl Pts',(-1.07827946534055,-4.12367098825238,
58.8949384049742));
#12914=CARTESIAN_POINT('Ctrl Pts',(2.8444759251399,-3.17414396432785,59.0911912875147));
#12915=CARTESIAN_POINT('Ctrl Pts',(4.21703180839744,0.621592580311748,59.2874441700555));
#12916=CARTESIAN_POINT('Ctrl Pts',(1.80697239801379,3.86022288112327,59.4836970525959));
#12917=CARTESIAN_POINT('Ctrl Pts',(-2.22132941175433,3.63667454350762,59.6799499351367));
#12918=CARTESIAN_POINT('Ctrl Pts',(-4.26195603608509,0.153196666955191,
59.8762028176772));
#12919=CARTESIAN_POINT('Ctrl Pts',(-2.47203876653822,-3.47020464397426,
60.0724557002181));
#12920=CARTESIAN_POINT('Ctrl Pts',(0.185380513169834,-3.80573422454402,
60.203290955245));
#12921=CARTESIAN_POINT('Ctrl Pts',(1.2966041888132,-3.37937853262027,60.2687085827586));
#12922=CARTESIAN_POINT('Ctrl Pts',(-3.84150956301618,0.309966383025731,
49.7319682174301));
#12923=CARTESIAN_POINT('Ctrl Pts',(-3.94343421577317,-0.953217464367681,
49.7973858449436));
#12924=CARTESIAN_POINT('Ctrl Pts',(-2.80283521184197,-3.56718891944667,
49.9282210999707));
#12925=CARTESIAN_POINT('Ctrl Pts',(1.43606495288148,-4.30784024715974,50.1244739825114));
#12926=CARTESIAN_POINT('Ctrl Pts',(4.38198226899745,-1.17737874838892,50.3207268650521));
#12927=CARTESIAN_POINT('Ctrl Pts',(3.40093404822038,3.00488023396059,50.5169797475926));
#12928=CARTESIAN_POINT('Ctrl Pts',(-0.631085367097292,4.49456228077927,
50.7132326301334));
#12929=CARTESIAN_POINT('Ctrl Pts',(-4.09656762707307,1.9528243383506,50.9094855126739));
#12930=CARTESIAN_POINT('Ctrl Pts',(-3.88883676405956,-2.33957322574722,
51.1057383952146));
#12931=CARTESIAN_POINT('Ctrl Pts',(-0.193703531802759,-4.53425085692975,
51.3019912777552));
#12932=CARTESIAN_POINT('Ctrl Pts',(3.6750515846993,-2.66279277449443,51.4982441602959));
#12933=CARTESIAN_POINT('Ctrl Pts',(4.24830803828541,1.59641482454314,51.6944970428365));
#12934=CARTESIAN_POINT('Ctrl Pts',(1.01194922137185,4.42409711458196,51.8907499253772));
#12935=CARTESIAN_POINT('Ctrl Pts',(-3.13184741346485,3.28453219663654,52.0870028079178));
#12936=CARTESIAN_POINT('Ctrl Pts',(-4.46721985415561,-0.800371309716849,
52.2832556904585));
#12937=CARTESIAN_POINT('Ctrl Pts',(-1.79668890507018,-4.16755989036541,
52.4795085729991));
#12938=CARTESIAN_POINT('Ctrl Pts',(2.48499000814928,-3.79756037046334,52.6757614555397));
#12939=CARTESIAN_POINT('Ctrl Pts',(4.53829841749185,-0.0221663152455843,
52.8720143380803));
#12940=CARTESIAN_POINT('Ctrl Pts',(2.52196715058651,3.77310549519735,53.0682672206211));
#12941=CARTESIAN_POINT('Ctrl Pts',(-1.75589368914209,4.18491099806776,53.2645201031617));
#12942=CARTESIAN_POINT('Ctrl Pts',(-4.45918779403821,0.843971221778929,
53.4607729857023));
#12943=CARTESIAN_POINT('Ctrl Pts',(-3.16378355698353,-3.25378498150801,
53.6570258682431));
#12944=CARTESIAN_POINT('Ctrl Pts',(0.968687974786214,-4.4337666426907,53.8532787507835));
#12945=CARTESIAN_POINT('Ctrl Pts',(4.23250559570023,-1.63784598787967,54.0495316333243));
#12946=CARTESIAN_POINT('Ctrl Pts',(3.70089818735484,2.62678428619937,54.2457845158648));
#12947=CARTESIAN_POINT('Ctrl Pts',(-0.149424640121008,4.53589190242274,
54.4420373984056));
#12948=CARTESIAN_POINT('Ctrl Pts',(-3.86575354839818,2.37751815656555,54.6382902809461));
#12949=CARTESIAN_POINT('Ctrl Pts',(-4.11553588589404,-1.91285322225766,
54.8345431634869));
#12950=CARTESIAN_POINT('Ctrl Pts',(-0.674783731706433,-4.4879070838652,
55.0307960460274));
#12951=CARTESIAN_POINT('Ctrl Pts',(3.3710688781024,-3.03850912469279,55.2270489285682));
#12952=CARTESIAN_POINT('Ctrl Pts',(4.3939747027473,1.13561850335233,55.4233018111087));
#12953=CARTESIAN_POINT('Ctrl Pts',(1.47666092080595,4.29140019158721,55.6195546936494));
#12954=CARTESIAN_POINT('Ctrl Pts',(-2.76482260024748,3.59894416277999,55.8158075761901));
#12955=CARTESIAN_POINT('Ctrl Pts',(-4.52700002573295,-0.320801810073011,
56.0120604587307));
#12956=CARTESIAN_POINT('Ctrl Pts',(-2.22966973931158,-3.95287439149345,
56.2083133412713));
#12957=CARTESIAN_POINT('Ctrl Pts',(2.06707774460212,-4.04027632761189,56.4045662238119));
#12958=CARTESIAN_POINT('Ctrl Pts',(4.51020950965979,-0.504631438073187,
56.6008191063527));
#12959=CARTESIAN_POINT('Ctrl Pts',(2.90889028804564,3.48353278707687,56.7970719888932));
#12960=CARTESIAN_POINT('Ctrl Pts',(-1.30092547300982,4.34790027316804,56.993324871434));
#12961=CARTESIAN_POINT('Ctrl Pts',(-4.34415860534098,1.31336442755139,57.1895777539745));
#12962=CARTESIAN_POINT('Ctrl Pts',(-3.49184497436551,-2.89890757637825,
57.3858306365152));
#12963=CARTESIAN_POINT('Ctrl Pts',(0.491721548358648,-4.51163577626339,
57.5820835190559));
#12964=CARTESIAN_POINT('Ctrl Pts',(4.03434089226244,-2.07863261231695,57.7783364015964));
#12965=CARTESIAN_POINT('Ctrl Pts',(3.95924494651409,2.2183453201407,57.9745892841372));
#12966=CARTESIAN_POINT('Ctrl Pts',(0.333747668240588,4.52606605940804,58.1708421666777));
#12967=CARTESIAN_POINT('Ctrl Pts',(-3.59099606622211,2.77510662182156,58.3670950492184));
#12968=CARTESIAN_POINT('Ctrl Pts',(-4.29564880395483,-1.46436103638495,
58.563347931759));
#12969=CARTESIAN_POINT('Ctrl Pts',(-1.14811104286864,-4.39072833244981,
58.7596008142997));
#12970=CARTESIAN_POINT('Ctrl Pts',(3.02868998789261,-3.37970800171799,58.9558536968403));
#12971=CARTESIAN_POINT('Ctrl Pts',(4.49013538973434,0.661848183667063,59.152106579381));
#12972=CARTESIAN_POINT('Ctrl Pts',(1.92399561616732,4.11021878855135,59.3483594619216));
#12973=CARTESIAN_POINT('Ctrl Pts',(-2.36518723527633,3.87219300462306,59.5446123444623));
#12974=CARTESIAN_POINT('Ctrl Pts',(-4.53796900203841,0.163117995580461,
59.7408652270028));
#12975=CARTESIAN_POINT('Ctrl Pts',(-2.63213303924464,-3.69494217484943,
59.9371181095436));
#12976=CARTESIAN_POINT('Ctrl Pts',(0.197386133320944,-4.05220133543222,
60.0679533645706));
#12977=CARTESIAN_POINT('Ctrl Pts',(1.38057492074749,-3.59823397926732,60.1333709920842));
#12978=CARTESIAN_POINT('Ctrl Pts',(-4.07516176463982,0.32881947362338,49.5966306267557));
#12979=CARTESIAN_POINT('Ctrl Pts',(-4.18328578228859,-1.01119502644896,
49.6620482542693));
#12980=CARTESIAN_POINT('Ctrl Pts',(-2.97331210570162,-3.78415611189113,
49.7928835092963));
#12981=CARTESIAN_POINT('Ctrl Pts',(1.523410755986,-4.56985608793288,49.989136391837));
#12982=CARTESIAN_POINT('Ctrl Pts',(4.64850765122846,-1.2489904760687,50.1853892743776));
#12983=CARTESIAN_POINT('Ctrl Pts',(3.6077891177987,3.18764611564409,50.3816421569182));
#12984=CARTESIAN_POINT('Ctrl Pts',(-0.669469883136082,4.76793511898564,
50.5778950394589));
#12985=CARTESIAN_POINT('Ctrl Pts',(-4.34573322967388,2.07160100636482,50.7741479219996));
#12986=CARTESIAN_POINT('Ctrl Pts',(-4.12536754883888,-2.48187312793108,
50.9704008045402));
#12987=CARTESIAN_POINT('Ctrl Pts',(-0.205485165018958,-4.81003767407975,
51.1666536870808));
#12988=CARTESIAN_POINT('Ctrl Pts',(3.89857930987077,-2.8247518648005,51.3629065696215));
#12989=CARTESIAN_POINT('Ctrl Pts',(4.50670295050357,1.69351359062463,51.5591594521622));
#12990=CARTESIAN_POINT('Ctrl Pts',(1.07349902611038,4.69318404878375,51.7554123347027));
#12991=CARTESIAN_POINT('Ctrl Pts',(-3.32233582207128,3.48430735441209,51.9516652172434));
#12992=CARTESIAN_POINT('Ctrl Pts',(-4.73892964348144,-0.84905230752879,
52.1479180997841));
#12993=CARTESIAN_POINT('Ctrl Pts',(-1.90596894496492,-4.42104345660641,
52.3441709823247));
#12994=CARTESIAN_POINT('Ctrl Pts',(2.63613459776757,-4.02853944959931,52.5404238648654));
#12995=CARTESIAN_POINT('Ctrl Pts',(4.8143314194869,-0.0235145374155529,
52.736676747406));
#12996=CARTESIAN_POINT('Ctrl Pts',(2.67536080156949,4.0025971550382,52.9329296299466));
#12997=CARTESIAN_POINT('Ctrl Pts',(-1.86269244092313,4.43944991102827,53.1291825124873));
#12998=CARTESIAN_POINT('Ctrl Pts',(-4.73040904923462,0.895304097785309,
53.3254353950279));
#12999=CARTESIAN_POINT('Ctrl Pts',(-3.35621441819151,-3.45169000089377,
53.5216882775686));
#13000=CARTESIAN_POINT('Ctrl Pts',(1.02760649998635,-4.70344170676544,53.7179411601092));
#13001=CARTESIAN_POINT('Ctrl Pts',(4.48993935568372,-1.73746472231492,53.9141940426499));
#13002=CARTESIAN_POINT('Ctrl Pts',(3.92599798088014,2.78655323160816,54.1104469251905));
#13003=CARTESIAN_POINT('Ctrl Pts',(-0.158513097553788,4.81177853291072,
54.3066998077312));
#13004=CARTESIAN_POINT('Ctrl Pts',(-4.10088034235792,2.52212598392328,54.5029526902718));
#13005=CARTESIAN_POINT('Ctrl Pts',(-4.36585519522442,-2.02919872639653,
54.6992055728124));
#13006=CARTESIAN_POINT('Ctrl Pts',(-0.715826114120611,-4.76087513291625,
54.8954584553531));
#13007=CARTESIAN_POINT('Ctrl Pts',(3.57610745792964,-3.22332041697045,55.0917113378937));
#13008=CARTESIAN_POINT('Ctrl Pts',(4.66122950098068,1.20469024693651,55.2879642204344));
#13009=CARTESIAN_POINT('Ctrl Pts',(1.56647589315943,4.55241609858009,55.484217102975));
#13010=CARTESIAN_POINT('Ctrl Pts',(-2.93298745238425,3.81784280493093,55.6804699855157));
#13011=CARTESIAN_POINT('Ctrl Pts',(-4.80234582545348,-0.340313944034631,
55.8767228680562));
#13012=CARTESIAN_POINT('Ctrl Pts',(-2.36528497986683,-4.19330013797761,
56.0729757505969));
#13013=CARTESIAN_POINT('Ctrl Pts',(2.19280364949204,-4.28601812354619,56.2692286331376));
#13014=CARTESIAN_POINT('Ctrl Pts',(4.78453405953504,-0.53532464463174,56.4654815156782));
#13015=CARTESIAN_POINT('Ctrl Pts',(3.08581777161277,3.69541176115642,56.6617343982189));
#13016=CARTESIAN_POINT('Ctrl Pts',(-1.38005168522687,4.61235268558585,56.8579872807595));
#13017=CARTESIAN_POINT('Ctrl Pts',(-4.60838343823277,1.39324721451252,57.0542401633002));
#13018=CARTESIAN_POINT('Ctrl Pts',(-3.70422952075418,-3.0752278813035,57.2504930458408));
#13019=CARTESIAN_POINT('Ctrl Pts',(0.521629536475065,-4.78604707597658,
57.4467459283814));
#13020=CARTESIAN_POINT('Ctrl Pts',(4.27972167711132,-2.20506131912283,57.6429988109221));
#13021=CARTESIAN_POINT('Ctrl Pts',(4.20005816937483,2.35327177535572,57.8392516934627));
#13022=CARTESIAN_POINT('Ctrl Pts',(0.354047208354176,4.80135505247888,58.0355045760034));
#13023=CARTESIAN_POINT('Ctrl Pts',(-3.80941128116065,2.94389697917782,58.231757458544));
#13024=CARTESIAN_POINT('Ctrl Pts',(-4.55692312437015,-1.55342789265866,
58.4280103410846));
#13025=CARTESIAN_POINT('Ctrl Pts',(-1.21794262039674,-4.65778567664726,
58.6242632236253));
#13026=CARTESIAN_POINT('Ctrl Pts',(3.21290405064532,-3.58527203910813,58.8205161061659));
#13027=CARTESIAN_POINT('Ctrl Pts',(4.76323897107123,0.702103787022373,59.0167689887067));
#13028=CARTESIAN_POINT('Ctrl Pts',(2.04101883432086,4.36021469597944,59.2130218712472));
#13029=CARTESIAN_POINT('Ctrl Pts',(-2.50904505879833,4.10771146573851,59.4092747537879));
#13030=CARTESIAN_POINT('Ctrl Pts',(-4.81398196799173,0.173039324205733,
59.6055276363284));
#13031=CARTESIAN_POINT('Ctrl Pts',(-2.79222731195107,-3.9196797057246,59.8017805188692));
#13032=CARTESIAN_POINT('Ctrl Pts',(0.209391753472049,-4.29866844632042,
59.9326157738963));
#13033=CARTESIAN_POINT('Ctrl Pts',(1.46454565268177,-3.81708942591437,59.9980334014098));
#13034=CARTESIAN_POINT('Ctrl Pts',(1.46332546897508,-3.81390922438499,60.));
#13035=CARTESIAN_POINT('Ctrl Pts',(1.34436836356881,-3.84840020465489,60.));
#13036=CARTESIAN_POINT('Ctrl Pts',(1.22405644550263,-3.87694498383428,60.));
#13037=CARTESIAN_POINT('Ctrl Pts',(1.10278998189303,-3.89970205494259,60.));
#13038=CARTESIAN_POINT('Ctrl Pts',(0.979743769206862,-3.92279311679397,
60.));
#13039=CARTESIAN_POINT('Ctrl Pts',(0.855713935497655,-3.93992519841741,
60.));
#13040=CARTESIAN_POINT('Ctrl Pts',(0.731113253599479,-3.95120932990782,
60.));
#13041=CARTESIAN_POINT('Ctrl Pts',(0.606016724725583,-3.96253836646928,
60.));
#13042=CARTESIAN_POINT('Ctrl Pts',(0.480343917845818,-3.96797258676211,
60.));
#13043=CARTESIAN_POINT('Ctrl Pts',(0.354520267150776,-3.96757271750024,
60.));
#13044=CARTESIAN_POINT('Ctrl Pts',(0.236435009120947,-3.96719744095481,
60.));
#13045=CARTESIAN_POINT('Ctrl Pts',(0.118216376475947,-3.96168300047746,
60.));
#13046=CARTESIAN_POINT('Ctrl Pts',(0.000232491209287232,-3.95104119203084,
60.));
#13047=CARTESIAN_POINT('Ctrl Pts',(-0.0270686093560331,-3.94857871097302,
60.));
#13048=CARTESIAN_POINT('Ctrl Pts',(-0.0543570496058564,-3.9458415373458,
60.));
#13049=CARTESIAN_POINT('Ctrl Pts',(-0.0816280901417187,-3.94282955007168,
60.));
#13050=CARTESIAN_POINT('Ctrl Pts',(-0.0980670002502211,-3.94101393221939,
60.));
#13051=CARTESIAN_POINT('Ctrl Pts',(-0.11448987603851,-3.93909952500333,
60.));
#13052=CARTESIAN_POINT('Ctrl Pts',(-0.130895119287348,-3.93708671595757,
60.));
#13053=CARTESIAN_POINT('Ctrl Pts',(-0.253258278521662,-3.922073608865,60.));
#13054=CARTESIAN_POINT('Ctrl Pts',(-0.374653550889227,-3.90158893120011,
60.));
#13055=CARTESIAN_POINT('Ctrl Pts',(-0.494687238785102,-3.87573365348574,
60.));
#13056=CARTESIAN_POINT('Ctrl Pts',(-0.614101450198027,-3.85001181111594,
60.));
#13057=CARTESIAN_POINT('Ctrl Pts',(-0.732168902791401,-3.81897433807138,
60.));
#13058=CARTESIAN_POINT('Ctrl Pts',(-0.848484137137308,-3.78267264792025,
60.));
#13059=CARTESIAN_POINT('Ctrl Pts',(-0.962109235726436,-3.7472105423279,
60.));
#13060=CARTESIAN_POINT('Ctrl Pts',(-1.07406285827702,-3.70672450335135,
60.));
#13061=CARTESIAN_POINT('Ctrl Pts',(-1.18393954190618,-3.66122205541169,
60.));
#13062=CARTESIAN_POINT('Ctrl Pts',(-1.27514614729463,-3.62345131391892,
60.));
#13063=CARTESIAN_POINT('Ctrl Pts',(-1.36492137435496,-3.5822233159453,60.));
#13064=CARTESIAN_POINT('Ctrl Pts',(-1.45301378049063,-3.53752319123988,
60.));
#13065=CARTESIAN_POINT('Ctrl Pts',(-1.47260001339677,-3.52758468357708,
60.));
#13066=CARTESIAN_POINT('Ctrl Pts',(-1.49210297812145,-3.51747447034406,
60.));
#13067=CARTESIAN_POINT('Ctrl Pts',(-1.51151976882622,-3.5071922786389,60.));
#13068=CARTESIAN_POINT('Ctrl Pts',(-1.52703531384485,-3.49897599765215,
60.));
#13069=CARTESIAN_POINT('Ctrl Pts',(-1.54248829386977,-3.4906538686883,60.));
#13070=CARTESIAN_POINT('Ctrl Pts',(-1.55787301693303,-3.48222851609215,
60.));
#13071=CARTESIAN_POINT('Ctrl Pts',(-1.66023918258982,-3.42616829089158,
60.));
#13072=CARTESIAN_POINT('Ctrl Pts',(-1.75964967742654,-3.36550766599683,
60.));
#13073=CARTESIAN_POINT('Ctrl Pts',(-1.85574301784674,-3.30029197211021,
60.));
#13074=CARTESIAN_POINT('Ctrl Pts',(-1.95138228900223,-3.2353844415369,60.));
#13075=CARTESIAN_POINT('Ctrl Pts',(-2.04373633146293,-3.16596450359091,
60.));
#13076=CARTESIAN_POINT('Ctrl Pts',(-2.13241450197746,-3.09203869892246,
60.));
#13077=CARTESIAN_POINT('Ctrl Pts',(-2.14806574423071,-3.07899117357412,
60.));
#13078=CARTESIAN_POINT('Ctrl Pts',(-2.16360238068116,-3.06580319830772,
60.));
#13079=CARTESIAN_POINT('Ctrl Pts',(-2.17902212861498,-3.05247469509659,
60.));
#13080=CARTESIAN_POINT('Ctrl Pts',(-2.26873549460814,-2.97492836347992,
60.));
#13081=CARTESIAN_POINT('Ctrl Pts',(-2.3544959880784,-2.89262699475134,60.));
#13082=CARTESIAN_POINT('Ctrl Pts',(-2.43611517004137,-2.80597529075037,
60.));
#13083=CARTESIAN_POINT('Ctrl Pts',(-2.48139017941949,-2.75790868904081,
60.));
#13084=CARTESIAN_POINT('Ctrl Pts',(-2.52539005963298,-2.70850304152369,
60.));
#13085=CARTESIAN_POINT('Ctrl Pts',(-2.56807609809654,-2.65782521592468,
60.));
#13086=CARTESIAN_POINT('Ctrl Pts',(-2.58354147909752,-2.63946436752084,
60.));
#13087=CARTESIAN_POINT('Ctrl Pts',(-2.59883435230139,-2.62093651679172,
60.));
#13088=CARTESIAN_POINT('Ctrl Pts',(-2.61395271713795,-2.60224481794349,
60.));
#13089=CARTESIAN_POINT('Ctrl Pts',(-2.62426766003826,-2.58949186427332,
60.));
#13090=CARTESIAN_POINT('Ctrl Pts',(-2.63450128189901,-2.57666264063865,
60.));
#13091=CARTESIAN_POINT('Ctrl Pts',(-2.64464422032148,-2.56376952712175,
60.));
#13092=CARTESIAN_POINT('Ctrl Pts',(-2.71647381695367,-2.47246392073068,
60.));
#13093=CARTESIAN_POINT('Ctrl Pts',(-2.78387371613041,-2.37781639842496,
60.));
#13094=CARTESIAN_POINT('Ctrl Pts',(-2.84672278780816,-2.28023988477505,
60.));
#13095=CARTESIAN_POINT('Ctrl Pts',(-2.90983003259932,-2.18226254368803,
60.));
#13096=CARTESIAN_POINT('Ctrl Pts',(-2.96834927587283,-2.08133117047599,
60.));
#13097=CARTESIAN_POINT('Ctrl Pts',(-3.02211025220274,-1.97784096098337,
60.));
#13098=CARTESIAN_POINT('Ctrl Pts',(-3.07502331645505,-1.87598298744577,
60.));
#13099=CARTESIAN_POINT('Ctrl Pts',(-3.12332713951146,-1.77164536324422,
60.));
#13100=CARTESIAN_POINT('Ctrl Pts',(-3.16681056806896,-1.66519640248744,
60.));
#13101=CARTESIAN_POINT('Ctrl Pts',(-3.20826497072667,-1.56371456841652,
60.));
#13102=CARTESIAN_POINT('Ctrl Pts',(-3.24533818764054,-1.46031316007369,
60.));
#13103=CARTESIAN_POINT('Ctrl Pts',(-3.27780325480812,-1.35531477701105,
60.));
#13104=CARTESIAN_POINT('Ctrl Pts',(-3.28326313294003,-1.33765646222576,
60.));
#13105=CARTESIAN_POINT('Ctrl Pts',(-3.28858985830397,-1.31996173909606,
60.));
#13106=CARTESIAN_POINT('Ctrl Pts',(-3.29378192183614,-1.30223481302024,
60.));
#13107=CARTESIAN_POINT('Ctrl Pts',(-3.32564288426071,-1.19345399358192,
60.));
#13108=CARTESIAN_POINT('Ctrl Pts',(-3.35244706188043,-1.08342861884937,
60.));
#13109=CARTESIAN_POINT('Ctrl Pts',(-3.37400268186516,-0.972525911804353,
60.));
#13110=CARTESIAN_POINT('Ctrl Pts',(-3.38941338834796,-0.89323851169108,
60.));
#13111=CARTESIAN_POINT('Ctrl Pts',(-3.40214040744648,-0.813502527884589,
60.));
#13112=CARTESIAN_POINT('Ctrl Pts',(-3.4120970300337,-0.733453791823358,
60.));
#13113=CARTESIAN_POINT('Ctrl Pts',(-3.41707534132731,-0.693429423792743,
60.));
#13114=CARTESIAN_POINT('Ctrl Pts',(-3.42136083200587,-0.653326908117905,
60.));
#13115=CARTESIAN_POINT('Ctrl Pts',(-3.42494130955714,-0.613163563714322,
60.));
#13116=CARTESIAN_POINT('Ctrl Pts',(-3.42733857929183,-0.586272634053829,
60.));
#13117=CARTESIAN_POINT('Ctrl Pts',(-3.42941992625259,-0.559352204490316,
60.));
#13118=CARTESIAN_POINT('Ctrl Pts',(-3.43118099378155,-0.532414906879469,
60.));
#13119=CARTESIAN_POINT('Ctrl Pts',(-3.43205019462101,-0.519119606550955,
60.));
#13120=CARTESIAN_POINT('Ctrl Pts',(-3.43284129656963,-0.505821333168536,
60.));
#13121=CARTESIAN_POINT('Ctrl Pts',(-3.43355375141007,-0.492524272718991,
60.));
#13122=CARTESIAN_POINT('Ctrl Pts',(-3.43931430586481,-0.385010874731565,
60.));
#13123=CARTESIAN_POINT('Ctrl Pts',(-3.43994303873128,-0.277485424520412,
60.));
#13124=CARTESIAN_POINT('Ctrl Pts',(-3.43524294624951,-0.170275803271761,
60.));
#13125=CARTESIAN_POINT('Ctrl Pts',(-3.43095381794618,-0.072440319678238,
60.));
#13126=CARTESIAN_POINT('Ctrl Pts',(-3.42222653673074,0.0251324780656352,
60.));
#13127=CARTESIAN_POINT('Ctrl Pts',(-3.40887510827288,0.122182273906181,
60.));
#13128=CARTESIAN_POINT('Ctrl Pts',(-3.40196952873072,0.172378032872603,
60.));
#13129=CARTESIAN_POINT('Ctrl Pts',(-3.39382628966267,0.222433662010737,
60.));
#13130=CARTESIAN_POINT('Ctrl Pts',(-3.38446664719617,0.272313465330584,
60.));
#13131=CARTESIAN_POINT('Ctrl Pts',(-3.3787688286016,0.272628438300531,50.));
#13132=CARTESIAN_POINT('Ctrl Pts',(-3.398044957201,0.167781606543633,50.));
#13133=CARTESIAN_POINT('Ctrl Pts',(-3.4119369975876,0.0622133010350053,
50.));
#13134=CARTESIAN_POINT('Ctrl Pts',(-3.42067227660546,-0.0437408776964314,
50.));
#13135=CARTESIAN_POINT('Ctrl Pts',(-3.4296483594719,-0.15261587601,50.));
#13136=CARTESIAN_POINT('Ctrl Pts',(-3.4331795612354,-0.261898933983832,
50.));
#13137=CARTESIAN_POINT('Ctrl Pts',(-3.43146110672633,-0.371245945305364,
50.));
#13138=CARTESIAN_POINT('Ctrl Pts',(-3.43059312612378,-0.426476435418754,
50.));
#13139=CARTESIAN_POINT('Ctrl Pts',(-3.42838504090139,-0.481723495358662,
50.));
#13140=CARTESIAN_POINT('Ctrl Pts',(-3.42485710615297,-0.536943839237519,
50.));
#13141=CARTESIAN_POINT('Ctrl Pts',(-3.42359637193536,-0.55667724759124,
50.));
#13142=CARTESIAN_POINT('Ctrl Pts',(-3.42216768464111,-0.576397395127722,
50.));
#13143=CARTESIAN_POINT('Ctrl Pts',(-3.42057240953287,-0.596101939689996,
50.));
#13144=CARTESIAN_POINT('Ctrl Pts',(-3.41158937887145,-0.707058681294052,
50.));
#13145=CARTESIAN_POINT('Ctrl Pts',(-3.39732801924954,-0.817522731174477,
50.));
#13146=CARTESIAN_POINT('Ctrl Pts',(-3.37799845802815,-0.927138977536138,
50.));
#13147=CARTESIAN_POINT('Ctrl Pts',(-3.35829521492687,-1.03887434106446,
50.));
#13148=CARTESIAN_POINT('Ctrl Pts',(-3.33332592513191,-1.14972960302005,
50.));
#13149=CARTESIAN_POINT('Ctrl Pts',(-3.3032601024926,-1.25933625667802,50.));
#13150=CARTESIAN_POINT('Ctrl Pts',(-3.29844646564883,-1.27688464152349,
50.));
#13151=CARTESIAN_POINT('Ctrl Pts',(-3.29350208061623,-1.29440102123175,
50.));
#13152=CARTESIAN_POINT('Ctrl Pts',(-3.28842751996456,-1.31188387913012,
50.));
#13153=CARTESIAN_POINT('Ctrl Pts',(-3.2834078609544,-1.32917759009288,50.));
#13154=CARTESIAN_POINT('Ctrl Pts',(-3.27826010256289,-1.3464408573239,50.));
#13155=CARTESIAN_POINT('Ctrl Pts',(-3.27298715730616,-1.36366443683881,
50.));
#13156=CARTESIAN_POINT('Ctrl Pts',(-3.23910916783017,-1.47432370165853,
50.));
#13157=CARTESIAN_POINT('Ctrl Pts',(-3.20012754844998,-1.58315475274442,
50.));
#13158=CARTESIAN_POINT('Ctrl Pts',(-3.15627292953829,-1.68978377711049,
50.));
#13159=CARTESIAN_POINT('Ctrl Pts',(-3.1120226081207,-1.79737492070572,50.));
#13160=CARTESIAN_POINT('Ctrl Pts',(-3.0628108296211,-1.90272499793219,50.));
#13161=CARTESIAN_POINT('Ctrl Pts',(-3.00882082981536,-2.00545305375488,
50.));
#13162=CARTESIAN_POINT('Ctrl Pts',(-2.95521231287092,-2.10745525307056,
50.));
#13163=CARTESIAN_POINT('Ctrl Pts',(-2.89689260366845,-2.20687322975469,
50.));
#13164=CARTESIAN_POINT('Ctrl Pts',(-2.83399143376612,-2.30332392463489,
50.));
#13165=CARTESIAN_POINT('Ctrl Pts',(-2.77196506401352,-2.39843322821104,
50.));
#13166=CARTESIAN_POINT('Ctrl Pts',(-2.70548349258012,-2.49065802267417,
50.));
#13167=CARTESIAN_POINT('Ctrl Pts',(-2.63462677786824,-2.57960868853371,
50.));
#13168=CARTESIAN_POINT('Ctrl Pts',(-2.62467602866062,-2.59210045831754,
50.));
#13169=CARTESIAN_POINT('Ctrl Pts',(-2.61463966718517,-2.60452658608384,
50.));
#13170=CARTESIAN_POINT('Ctrl Pts',(-2.60452587293078,-2.61687649059976,
50.));
#13171=CARTESIAN_POINT('Ctrl Pts',(-2.52905384554601,-2.70903501275091,
50.));
#13172=CARTESIAN_POINT('Ctrl Pts',(-2.44915924290189,-2.79709501168693,
50.));
#13173=CARTESIAN_POINT('Ctrl Pts',(-2.36503095553586,-2.88066875053339,
50.));
#13174=CARTESIAN_POINT('Ctrl Pts',(-2.3451491342261,-2.90041951682089,50.));
#13175=CARTESIAN_POINT('Ctrl Pts',(-2.32503063734273,-2.91991966440883,
50.));
#13176=CARTESIAN_POINT('Ctrl Pts',(-2.30467755267561,-2.93916394474508,
50.));
#13177=CARTESIAN_POINT('Ctrl Pts',(-2.22198064086081,-3.01735565769346,
50.));
#13178=CARTESIAN_POINT('Ctrl Pts',(-2.13541444818756,-3.09132566298283,
50.));
#13179=CARTESIAN_POINT('Ctrl Pts',(-2.04539122416378,-3.16106159088775,
50.));
#13180=CARTESIAN_POINT('Ctrl Pts',(-1.95303496262569,-3.23260479172319,
50.));
#13181=CARTESIAN_POINT('Ctrl Pts',(-1.85703964938763,-3.29969204706846,
50.));
#13182=CARTESIAN_POINT('Ctrl Pts',(-1.75780798754775,-3.36227497304928,
50.));
#13183=CARTESIAN_POINT('Ctrl Pts',(-1.70235630506146,-3.39724696158808,
50.));
#13184=CARTESIAN_POINT('Ctrl Pts',(-1.64589330109836,-3.43081172826972,
50.));
#13185=CARTESIAN_POINT('Ctrl Pts',(-1.58848467446361,-3.46295546999867,
50.));
#13186=CARTESIAN_POINT('Ctrl Pts',(-1.56669561237047,-3.47515541320397,
50.));
#13187=CARTESIAN_POINT('Ctrl Pts',(-1.54477030125963,-3.4871506118423,50.));
#13188=CARTESIAN_POINT('Ctrl Pts',(-1.52271223344434,-3.49894015606824,
50.));
#13189=CARTESIAN_POINT('Ctrl Pts',(-1.50575545848698,-3.50800317328095,
50.));
#13190=CARTESIAN_POINT('Ctrl Pts',(-1.48872551819598,-3.51694176326732,
50.));
#13191=CARTESIAN_POINT('Ctrl Pts',(-1.47163483009586,-3.52575038926294,
50.));
#13192=CARTESIAN_POINT('Ctrl Pts',(-1.36499561930288,-3.58071277104894,
50.));
#13193=CARTESIAN_POINT('Ctrl Pts',(-1.25587296134188,-3.63068347298158,
50.));
#13194=CARTESIAN_POINT('Ctrl Pts',(-1.14472361822858,-3.67565706105989,
50.));
#13195=CARTESIAN_POINT('Ctrl Pts',(-1.03178949125138,-3.7213528138587,50.));
#13196=CARTESIAN_POINT('Ctrl Pts',(-0.916762391257988,-3.7618900713334,
50.));
#13197=CARTESIAN_POINT('Ctrl Pts',(-0.800081831029844,-3.79722493418074,
50.));
#13198=CARTESIAN_POINT('Ctrl Pts',(-0.682285258005057,-3.83289776385845,
50.));
#13199=CARTESIAN_POINT('Ctrl Pts',(-0.56280265193181,-3.86326859172821,
50.));
#13200=CARTESIAN_POINT('Ctrl Pts',(-0.44205744347992,-3.88824777960903,
50.));
#13201=CARTESIAN_POINT('Ctrl Pts',(-0.334854840094098,-3.91042533850035,
50.));
#13202=CARTESIAN_POINT('Ctrl Pts',(-0.226656168903308,-3.92835240650093,
50.));
#13203=CARTESIAN_POINT('Ctrl Pts',(-0.117746834687938,-3.94193358936827,
50.));
#13204=CARTESIAN_POINT('Ctrl Pts',(-0.0928091818766533,-3.94504335792532,
50.));
#13205=CARTESIAN_POINT('Ctrl Pts',(-0.0678276535994453,-3.94792574054485,
50.));
#13206=CARTESIAN_POINT('Ctrl Pts',(-0.0428407696516749,-3.95057590881759,
50.));
#13207=CARTESIAN_POINT('Ctrl Pts',(0.0829695540103623,-3.96391965063228,
50.));
#13208=CARTESIAN_POINT('Ctrl Pts',(0.209038870700189,-3.97139872228523,
50.));
#13209=CARTESIAN_POINT('Ctrl Pts',(0.334905058101018,-3.972971048347,50.));
#13210=CARTESIAN_POINT('Ctrl Pts',(0.460908954032592,-3.97454509466992,
50.));
#13211=CARTESIAN_POINT('Ctrl Pts',(0.586710165776045,-3.97019977642533,
50.));
#13212=CARTESIAN_POINT('Ctrl Pts',(0.711866498333914,-3.95984534068554,
50.));
#13213=CARTESIAN_POINT('Ctrl Pts',(0.834749370138242,-3.94967899293778,
50.));
#13214=CARTESIAN_POINT('Ctrl Pts',(0.957011452282639,-3.9337200035174,50.));
#13215=CARTESIAN_POINT('Ctrl Pts',(1.07824174393589,-3.91183445670416,50.));
#13216=CARTESIAN_POINT('Ctrl Pts',(1.14882044428184,-3.89909297576425,50.));
#13217=CARTESIAN_POINT('Ctrl Pts',(1.21904950303075,-3.88434180939321,50.));
#13218=CARTESIAN_POINT('Ctrl Pts',(1.28884726169396,-3.86754634556837,50.));
#13219=CARTESIAN_POINT('Ctrl Pts',(1.34761180649662,-3.85340580860388,50.));
#13220=CARTESIAN_POINT('Ctrl Pts',(1.40607062746006,-3.83781606804309,50.));
#13221=CARTESIAN_POINT('Ctrl Pts',(1.46419354633185,-3.82081011676438,50.));
#13222=CARTESIAN_POINT('Origin',(-5.03504358328054E-16,0.,50.));
#13223=CARTESIAN_POINT('Ctrl Pts',(3.17505078219416,-2.57026798806821,50.));
#13224=CARTESIAN_POINT('Ctrl Pts',(3.24523509733765,-2.46687553038923,50.));
#13225=CARTESIAN_POINT('Ctrl Pts',(3.31015861353681,-2.36019756641044,50.));
#13226=CARTESIAN_POINT('Ctrl Pts',(3.36981505207394,-2.25066384020241,50.));
#13227=CARTESIAN_POINT('Ctrl Pts',(3.43040434804249,-2.13941731730403,50.));
#13228=CARTESIAN_POINT('Ctrl Pts',(3.48556070638999,-2.02522414499354,50.));
#13229=CARTESIAN_POINT('Ctrl Pts',(3.53522634918029,-1.90851946139768,50.));
#13230=CARTESIAN_POINT('Ctrl Pts',(3.5564460412567,-1.85865727678377,50.));
#13231=CARTESIAN_POINT('Ctrl Pts',(3.57666279615249,-1.80833652507169,50.));
#13232=CARTESIAN_POINT('Ctrl Pts',(3.59586921884357,-1.75759093627737,50.));
#13233=CARTESIAN_POINT('Ctrl Pts',(3.6065618017966,-1.72933989617423,50.));
#13234=CARTESIAN_POINT('Ctrl Pts',(3.61694279150167,-1.70095237454767,50.));
#13235=CARTESIAN_POINT('Ctrl Pts',(3.62700082864274,-1.67246314294838,50.));
#13236=CARTESIAN_POINT('Ctrl Pts',(3.66865222780369,-1.554486211616,50.));
#13237=CARTESIAN_POINT('Ctrl Pts',(3.70480266953197,-1.43468347218372,50.));
#13238=CARTESIAN_POINT('Ctrl Pts',(3.73541042587578,-1.31348080674658,50.));
#13239=CARTESIAN_POINT('Ctrl Pts',(3.76589523593952,-1.19276499231163,50.));
#13240=CARTESIAN_POINT('Ctrl Pts',(3.79088177393648,-1.0706595858572,50.));
#13241=CARTESIAN_POINT('Ctrl Pts',(3.81027760599455,-0.94758574640565,50.));
#13242=CARTESIAN_POINT('Ctrl Pts',(3.81807683061491,-0.898096736813369,
50.));
#13243=CARTESIAN_POINT('Ctrl Pts',(3.82497150996076,-0.848451218381541,
50.));
#13244=CARTESIAN_POINT('Ctrl Pts',(3.83095329809871,-0.798677085168631,
50.));
#13245=CARTESIAN_POINT('Ctrl Pts',(3.83306694698269,-0.781089527954901,
50.));
#13246=CARTESIAN_POINT('Ctrl Pts',(3.83506545254141,-0.763495503405024,
50.));
#13247=CARTESIAN_POINT('Ctrl Pts',(3.8369487712744,-0.745896401652321,50.));
#13248=CARTESIAN_POINT('Ctrl Pts',(3.84995310709515,-0.62437441744116,50.));
#13249=CARTESIAN_POINT('Ctrl Pts',(3.85747000929851,-0.502607486434189,
50.));
#13250=CARTESIAN_POINT('Ctrl Pts',(3.85946271601747,-0.380991411560717,
50.));
#13251=CARTESIAN_POINT('Ctrl Pts',(3.86143713309906,-0.260491564121916,
50.));
#13252=CARTESIAN_POINT('Ctrl Pts',(3.85798820094272,-0.140138992815084,
50.));
#13253=CARTESIAN_POINT('Ctrl Pts',(3.84903013630596,-0.0203256074983453,
50.));
#13254=CARTESIAN_POINT('Ctrl Pts',(3.84031877784156,0.0961881028453232,
50.));
#13255=CARTESIAN_POINT('Ctrl Pts',(3.82639733308781,0.21219256465117,50.));
#13256=CARTESIAN_POINT('Ctrl Pts',(3.80714191444518,0.327310135268585,50.));
#13257=CARTESIAN_POINT('Ctrl Pts',(3.78801864936847,0.441637632310381,50.));
#13258=CARTESIAN_POINT('Ctrl Pts',(3.76363432380651,0.555091014364022,50.));
#13259=CARTESIAN_POINT('Ctrl Pts',(3.73382433235031,0.667273537351628,50.));
#13260=CARTESIAN_POINT('Ctrl Pts',(3.72965489737509,0.682964173682061,50.));
#13261=CARTESIAN_POINT('Ctrl Pts',(3.72537940927025,0.6986290799777,50.));
#13262=CARTESIAN_POINT('Ctrl Pts',(3.72100102262887,0.714254781139606,50.));
#13263=CARTESIAN_POINT('Ctrl Pts',(3.68974751216623,0.825793129565523,50.));
#13264=CARTESIAN_POINT('Ctrl Pts',(3.65321090588756,0.935503458745713,50.));
#13265=CARTESIAN_POINT('Ctrl Pts',(3.61131430658357,1.04303117745521,50.));
#13266=CARTESIAN_POINT('Ctrl Pts',(3.60007235780076,1.07188366492544,50.));
#13267=CARTESIAN_POINT('Ctrl Pts',(3.58844422947595,1.10057889493759,50.));
#13268=CARTESIAN_POINT('Ctrl Pts',(3.5764278521007,1.12910974135774,50.));
#13269=CARTESIAN_POINT('Ctrl Pts',(3.53097968982238,1.23701868076171,50.));
#13270=CARTESIAN_POINT('Ctrl Pts',(3.47998089180808,1.3425786226534,50.));
#13271=CARTESIAN_POINT('Ctrl Pts',(3.42377585100192,1.44551956867172,50.));
#13272=CARTESIAN_POINT('Ctrl Pts',(3.36714914422034,1.54923280653062,50.));
#13273=CARTESIAN_POINT('Ctrl Pts',(3.30523702670668,1.65028821482483,50.));
#13274=CARTESIAN_POINT('Ctrl Pts',(3.23835550909232,1.74837178168865,50.));
#13275=CARTESIAN_POINT('Ctrl Pts',(3.20504349173018,1.79722476228559,50.));
#13276=CARTESIAN_POINT('Ctrl Pts',(3.17049818267377,1.84533984771772,50.));
#13277=CARTESIAN_POINT('Ctrl Pts',(3.13475621275442,1.89267404943633,50.));
#13278=CARTESIAN_POINT('Ctrl Pts',(3.1196368449191,1.91269709821035,50.));
#13279=CARTESIAN_POINT('Ctrl Pts',(3.10430260645072,1.93258129321551,50.));
#13280=CARTESIAN_POINT('Ctrl Pts',(3.08875851336575,1.95232029170191,50.));
#13281=CARTESIAN_POINT('Ctrl Pts',(3.07718604865985,1.96701583309276,50.));
#13282=CARTESIAN_POINT('Ctrl Pts',(3.06550133267884,1.9816256810886,50.));
#13283=CARTESIAN_POINT('Ctrl Pts',(3.05371157276739,1.99614166688898,50.));
#13284=CARTESIAN_POINT('Ctrl Pts',(2.98053827720831,2.08623531826787,50.));
#13285=CARTESIAN_POINT('Ctrl Pts',(2.90324873921887,2.17280900608232,50.));
#13286=CARTESIAN_POINT('Ctrl Pts',(2.82218516087522,2.25561271799166,50.));
#13287=CARTESIAN_POINT('Ctrl Pts',(2.74120372507107,2.33833252406665,50.));
#13288=CARTESIAN_POINT('Ctrl Pts',(2.65645508440711,2.41729050520046,50.));
#13289=CARTESIAN_POINT('Ctrl Pts',(2.5682492184672,2.49219595040595,50.));
#13290=CARTESIAN_POINT('Ctrl Pts',(2.48188236538523,2.56553968454615,50.));
#13291=CARTESIAN_POINT('Ctrl Pts',(2.3922001582028,2.63499841901754,50.));
#13292=CARTESIAN_POINT('Ctrl Pts',(2.29947556791442,2.70025360331428,50.));
#13293=CARTESIAN_POINT('Ctrl Pts',(2.22429001464763,2.75316564228494,50.));
#13294=CARTESIAN_POINT('Ctrl Pts',(2.14710368697748,2.80331320719412,50.));
#13295=CARTESIAN_POINT('Ctrl Pts',(2.06805826776658,2.85050151206886,50.));
#13296=CARTESIAN_POINT('Ctrl Pts',(2.04933268687684,2.86168025498405,50.));
#13297=CARTESIAN_POINT('Ctrl Pts',(2.03049854742624,2.87269513025456,50.));
#13298=CARTESIAN_POINT('Ctrl Pts',(2.01158369015662,2.88352879838473,50.));
#13299=CARTESIAN_POINT('Ctrl Pts',(1.91478828735083,2.93896930504972,50.));
#13300=CARTESIAN_POINT('Ctrl Pts',(1.81576602416327,2.98973918263213,50.));
#13301=CARTESIAN_POINT('Ctrl Pts',(1.71479982556319,3.03557905684995,50.));
#13302=CARTESIAN_POINT('Ctrl Pts',(1.61533953705197,3.08073522969034,50.));
#13303=CARTESIAN_POINT('Ctrl Pts',(1.51399215317973,3.1211076533205,50.));
#13304=CARTESIAN_POINT('Ctrl Pts',(1.41101601441157,3.15639999041054,50.));
#13305=CARTESIAN_POINT('Ctrl Pts',(1.3110481444873,3.1906613232372,50.));
#13306=CARTESIAN_POINT('Ctrl Pts',(1.2095446961283,3.22013515814445,50.));
#13307=CARTESIAN_POINT('Ctrl Pts',(1.1067400605449,3.24450171044004,50.));
#13308=CARTESIAN_POINT('Ctrl Pts',(1.05060132164677,3.25780760379209,50.));
#13309=CARTESIAN_POINT('Ctrl Pts',(0.994074592830348,3.26958966548783,50.));
#13310=CARTESIAN_POINT('Ctrl Pts',(0.937198714841526,3.27978922887549,50.));
#13311=CARTESIAN_POINT('Ctrl Pts',(0.887344887209746,3.28872952646787,50.));
#13312=CARTESIAN_POINT('Ctrl Pts',(0.837222776659118,3.29645381842423,50.));
#13313=CARTESIAN_POINT('Ctrl Pts',(0.786872907515106,3.30296842846219,50.));
#13314=CARTESIAN_POINT('Ctrl Pts',(3.17769854739391,-2.57241140768573,50.0019668001262));
#13315=CARTESIAN_POINT('Ctrl Pts',(4.02357137049521,-1.5275051251144,50.0673844276397));
#13316=CARTESIAN_POINT('Ctrl Pts',(4.59067653632725,1.44432493371321,50.1982196826668));
#13317=CARTESIAN_POINT('Ctrl Pts',(1.32303540089108,4.6318390767834,50.3944725652074));
#13318=CARTESIAN_POINT('Ctrl Pts',(-3.13133040812979,3.65559906892329,50.5907254477481));
#13319=CARTESIAN_POINT('Ctrl Pts',(-4.77752052222781,-0.593745130084182,
50.7869783302887));
#13320=CARTESIAN_POINT('Ctrl Pts',(-2.13966303858673,-4.31314779114456,
50.9832312128294));
#13321=CARTESIAN_POINT('Ctrl Pts',(2.41695513486635,-4.16356472240538,51.1794840953701));
#13322=CARTESIAN_POINT('Ctrl Pts',(4.80618344626051,-0.281002499380672,
51.3757369779108));
#13323=CARTESIAN_POINT('Ctrl Pts',(2.88556513840277,3.85385660156029,51.5719898604514));
#13324=CARTESIAN_POINT('Ctrl Pts',(-1.62263998902743,4.53268077196006,51.768242742992));
#13325=CARTESIAN_POINT('Ctrl Pts',(-4.67576771837635,1.14698163614136,51.9644956255326));
#13326=CARTESIAN_POINT('Ctrl Pts',(-3.53598465659234,-3.26729247706627,
52.1607485080733));
#13327=CARTESIAN_POINT('Ctrl Pts',(0.77463139421997,-4.75165975509162,52.3570013906139));
#13328=CARTESIAN_POINT('Ctrl Pts',(4.39060991305368,-1.97506951667604,52.5532542731545));
#13329=CARTESIAN_POINT('Ctrl Pts',(4.06938635955616,2.57263455668398,52.7495071556952));
#13330=CARTESIAN_POINT('Ctrl Pts',(0.0990119801423522,4.81337131475641,
52.9457600382359));
#13331=CARTESIAN_POINT('Ctrl Pts',(-3.96014959737916,2.73780316381413,53.1420129207765));
#13332=CARTESIAN_POINT('Ctrl Pts',(-4.46811663431751,-1.79284249136897,
53.3382658033171));
#13333=CARTESIAN_POINT('Ctrl Pts',(-0.969378574065539,-4.71578783221568,
53.5345186858578));
#13334=CARTESIAN_POINT('Ctrl Pts',(3.39863268272756,-3.40993345113973,53.7307715683984));
#13335=CARTESIAN_POINT('Ctrl Pts',(4.71897980158013,0.95371891518651,53.9270244509391));
#13336=CARTESIAN_POINT('Ctrl Pts',(1.80766469802749,4.46214056271427,54.1232773334797));
#13337=CARTESIAN_POINT('Ctrl Pts',(-2.72464196043686,3.96921608382251,54.3195302160203));
#13338=CARTESIAN_POINT('Ctrl Pts',(-4.81367381553503,-0.0830331856687988,
54.515783098561));
#13339=CARTESIAN_POINT('Ctrl Pts',(-2.58612825661705,-4.06082389990848,
54.7120359811016));
#13340=CARTESIAN_POINT('Ctrl Pts',(1.96048237593438,-4.3971421364971,54.9082888636423));
#13341=CARTESIAN_POINT('Ctrl Pts',(4.74906488512995,-0.790400422274602,
55.1045417461829));
#13342=CARTESIAN_POINT('Ctrl Pts',(3.27900690378524,3.52511898176996,55.3007946287236));
#13343=CARTESIAN_POINT('Ctrl Pts',(-1.13144290403263,4.67954987897574,55.4970475112642));
#13344=CARTESIAN_POINT('Ctrl Pts',(-4.52729116726062,1.63767664469671,55.6933003938049));
#13345=CARTESIAN_POINT('Ctrl Pts',(-3.86337062611881,-2.8727543434015,55.8895532763454));
#13346=CARTESIAN_POINT('Ctrl Pts',(0.264959644539609,-4.80709335455575,
56.0858061588862));
#13347=CARTESIAN_POINT('Ctrl Pts',(4.15569200315892,-2.4307558570938,56.2820590414267));
#13348=CARTESIAN_POINT('Ctrl Pts',(4.31988058961095,2.12531922976485,56.4783119239675));
#13349=CARTESIAN_POINT('Ctrl Pts',(0.610292135893617,4.77555167097707,56.6745648065081));
#13350=CARTESIAN_POINT('Ctrl Pts',(-3.6465650167766,3.14339200176368,56.8708176890487));
#13351=CARTESIAN_POINT('Ctrl Pts',(-4.63342916476401,-1.30754909347115,
57.0670705715894));
#13352=CARTESIAN_POINT('Ctrl Pts',(-1.46534692102897,-4.58596875244958,
57.26332345413));
#13353=CARTESIAN_POINT('Ctrl Pts',(3.01675902475045,-3.7520010357832,57.4595763366706));
#13354=CARTESIAN_POINT('Ctrl Pts',(4.79364012442147,0.44650673356943,57.6558292192113));
#13355=CARTESIAN_POINT('Ctrl Pts',(2.27190706938155,4.24461933186031,57.852082101752));
#13356=CARTESIAN_POINT('Ctrl Pts',(-2.28711553473289,4.23644034017381,58.0483349842925));
#13357=CARTESIAN_POINT('Ctrl Pts',(-4.79521384845463,0.429315466689967,
58.2445878668332));
#13358=CARTESIAN_POINT('Ctrl Pts',(-3.00327566838071,-3.76280558753283,
58.4408407493739));
#13359=CARTESIAN_POINT('Ctrl Pts',(1.48177178817488,-4.5806667508406,58.6370936319145));
#13360=CARTESIAN_POINT('Ctrl Pts',(4.63811714181827,-1.29095555776593,58.8333465144552));
#13361=CARTESIAN_POINT('Ctrl Pts',(3.6352112313189,3.15651723066099,59.0295993969958));
#13362=CARTESIAN_POINT('Ctrl Pts',(-0.627304473579594,4.77319939024576,
59.2258522795364));
#13363=CARTESIAN_POINT('Ctrl Pts',(-4.32769908146539,2.1100764079135,59.4221051620771));
#13364=CARTESIAN_POINT('Ctrl Pts',(-4.1465008886248,-2.44617374698532,59.6183580446177));
#13365=CARTESIAN_POINT('Ctrl Pts',(-0.248607397570823,-4.80695631761555,
59.8146109271585));
#13366=CARTESIAN_POINT('Ctrl Pts',(3.87543306135802,-2.8610093484926,60.0108638096989));
#13367=CARTESIAN_POINT('Ctrl Pts',(4.51789674603907,1.65944634992689,60.2071616790379));
#13368=CARTESIAN_POINT('Ctrl Pts',(2.2528534253199,3.66744558551292,60.3380419208631));
#13369=CARTESIAN_POINT('Ctrl Pts',(0.943870013894813,3.9779614512679,60.403504535175));
#13370=CARTESIAN_POINT('Ctrl Pts',(2.9951670455048,-2.42464845575103,49.8663796336412));
#13371=CARTESIAN_POINT('Ctrl Pts',(3.79245173650198,-1.43976306888344,49.9317972611547));
#13372=CARTESIAN_POINT('Ctrl Pts',(4.32698157899718,1.36136086539945,50.0626325161818));
#13373=CARTESIAN_POINT('Ctrl Pts',(1.24703837500101,4.36577968487308,50.2588853987225));
#13374=CARTESIAN_POINT('Ctrl Pts',(-2.95146235778382,3.44561628471545,50.4551382812631));
#13375=CARTESIAN_POINT('Ctrl Pts',(-4.50309298191142,-0.559639569497738,
50.6513911638038));
#13376=CARTESIAN_POINT('Ctrl Pts',(-2.01675776543231,-4.0653944777181,50.8476440463444));
#13377=CARTESIAN_POINT('Ctrl Pts',(2.27812181125624,-3.92440367214893,51.043896928885));
#13378=CARTESIAN_POINT('Ctrl Pts',(4.53010946702169,-0.264861318119594,
51.2401498114257));
#13379=CARTESIAN_POINT('Ctrl Pts',(2.7198141929761,3.63248562408825,51.4364026939663));
#13380=CARTESIAN_POINT('Ctrl Pts',(-1.52943325157104,4.27231717341537,51.632655576507));
#13381=CARTESIAN_POINT('Ctrl Pts',(-4.4071850031217,1.08109738766354,51.8289084590476));
#13382=CARTESIAN_POINT('Ctrl Pts',(-3.33287269351643,-3.07961457305647,
52.0251613415883));
#13383=CARTESIAN_POINT('Ctrl Pts',(0.730135470617217,-4.4787176938397,52.2214142241289));
#13384=CARTESIAN_POINT('Ctrl Pts',(4.13840706571432,-1.86161872836576,52.4176671066696));
#13385=CARTESIAN_POINT('Ctrl Pts',(3.83563504775033,2.42485878675501,52.6139199892101));
#13386=CARTESIAN_POINT('Ctrl Pts',(0.0933245918735013,4.53688445417833,
52.8101728717508));
#13387=CARTESIAN_POINT('Ctrl Pts',(-3.73267299979315,2.5805398753321,53.0064257542915));
#13388=CARTESIAN_POINT('Ctrl Pts',(-4.2114616912152,-1.68985908129423,53.2026786368321));
#13389=CARTESIAN_POINT('Ctrl Pts',(-0.913696096831058,-4.44490630498251,
53.3989315193728));
#13390=CARTESIAN_POINT('Ctrl Pts',(3.20341041142166,-3.21406204770251,53.5951844019134));
#13391=CARTESIAN_POINT('Ctrl Pts',(4.44791492310913,0.898935950920812,53.7914372844541));
#13392=CARTESIAN_POINT('Ctrl Pts',(1.70382987942474,4.20582889362266,53.9876901669947));
#13393=CARTESIAN_POINT('Ctrl Pts',(-2.56813467010359,3.74121869442359,54.1839430495353));
#13394=CARTESIAN_POINT('Ctrl Pts',(-4.5371695788841,-0.0782636419689434,
54.380195932076));
#13395=CARTESIAN_POINT('Ctrl Pts',(-2.43757738946658,-3.82756442790307,
54.5764488146166));
#13396=CARTESIAN_POINT('Ctrl Pts',(1.84786949363316,-4.14456406899824,54.7727016971573));
#13397=CARTESIAN_POINT('Ctrl Pts',(4.47627187688111,-0.744998703382836,
54.968954579698));
#13398=CARTESIAN_POINT('Ctrl Pts',(3.09065610652554,3.32263115843381,55.1652074622385));
#13399=CARTESIAN_POINT('Ctrl Pts',(-1.06645122231876,4.41074991106344,55.3614603447792));
#13400=CARTESIAN_POINT('Ctrl Pts',(-4.26723715523765,1.54360618045763,55.5577132273198));
#13401=CARTESIAN_POINT('Ctrl Pts',(-3.64145314961115,-2.70773926817054,
55.7539661098605));
#13402=CARTESIAN_POINT('Ctrl Pts',(0.249739987565699,-4.53096710889666,
55.9502189924011));
#13403=CARTESIAN_POINT('Ctrl Pts',(3.91698317303808,-2.29112980046708,56.1464718749418));
#13404=CARTESIAN_POINT('Ctrl Pts',(4.0717405347118,2.00323788528963,56.3427247574824));
#13405=CARTESIAN_POINT('Ctrl Pts',(0.575236091874863,4.501237224263,56.5389776400231));
#13406=CARTESIAN_POINT('Ctrl Pts',(-3.43710116130976,2.96283111640888,56.7352305225637));
#13407=CARTESIAN_POINT('Ctrl Pts',(-4.36727843594967,-1.23244162299672,
56.9314834051044));
#13408=CARTESIAN_POINT('Ctrl Pts',(-1.38117532001182,-4.32254421688825,
57.127736287645));
#13409=CARTESIAN_POINT('Ctrl Pts',(2.84347211681614,-3.53648078616334,57.3239891701857));
#13410=CARTESIAN_POINT('Ctrl Pts',(4.51828665134137,0.420858754862052,57.5202420527263));
#13411=CARTESIAN_POINT('Ctrl Pts',(2.14140551193621,4.00080239012195,57.7164949352669));
#13412=CARTESIAN_POINT('Ctrl Pts',(-2.15574038151357,3.99309321129347,57.9127478178076));
#13413=CARTESIAN_POINT('Ctrl Pts',(-4.5197699784388,0.404654978682567,58.1090007003482));
#13414=CARTESIAN_POINT('Ctrl Pts',(-2.83076326351899,-3.54666470916903,
58.3052535828889));
#13415=CARTESIAN_POINT('Ctrl Pts',(1.39665671954312,-4.31754676975549,58.5015064654295));
#13416=CARTESIAN_POINT('Ctrl Pts',(4.37169712896714,-1.21680124346688,58.6977593479701));
#13417=CARTESIAN_POINT('Ctrl Pts',(3.4263995533575,2.97520241358248,58.8940122305108));
#13418=CARTESIAN_POINT('Ctrl Pts',(-0.591271216806967,4.49902006186603,
59.0902651130514));
#13419=CARTESIAN_POINT('Ctrl Pts',(-4.07910992132878,1.98887063269826,59.2865179955921));
#13420=CARTESIAN_POINT('Ctrl Pts',(-3.90832000913077,-2.30566206494264,
59.4827708781327));
#13421=CARTESIAN_POINT('Ctrl Pts',(-0.234327036805779,-4.53083794355226,
59.6790237606734));
#13422=CARTESIAN_POINT('Ctrl Pts',(3.65282270149852,-2.69666892239163,59.875276643214));
#13423=CARTESIAN_POINT('Ctrl Pts',(4.25838236286678,1.5641254030092,60.0715745125529));
#13424=CARTESIAN_POINT('Ctrl Pts',(2.12344633615567,3.45678232062606,60.2024547543781));
#13425=CARTESIAN_POINT('Ctrl Pts',(0.889652784458242,3.74946171558581,60.2679173686899));
#13426=CARTESIAN_POINT('Ctrl Pts',(2.81263554361569,-2.27688550381632,49.7307924671561));
#13427=CARTESIAN_POINT('Ctrl Pts',(3.56133210250875,-1.3520210126525,49.7962100946696));
#13428=CARTESIAN_POINT('Ctrl Pts',(4.06328662166709,1.27839679708567,49.9270453496967));
#13429=CARTESIAN_POINT('Ctrl Pts',(1.17104134911095,4.09972029296276,50.1232982322374));
#13430=CARTESIAN_POINT('Ctrl Pts',(-2.77159430743786,3.23563350050761,50.3195511147781));
#13431=CARTESIAN_POINT('Ctrl Pts',(-4.22866544159503,-0.525534008911289,
50.5158039973186));
#13432=CARTESIAN_POINT('Ctrl Pts',(-1.8938524922779,-3.81764116429163,50.7120568798594));
#13433=CARTESIAN_POINT('Ctrl Pts',(2.13928848764612,-3.68524262189247,50.9083097623999));
#13434=CARTESIAN_POINT('Ctrl Pts',(4.25403548778285,-0.248720136858517,
51.1045626449406));
#13435=CARTESIAN_POINT('Ctrl Pts',(2.55406324754943,3.41111464661623,51.3008155274813));
#13436=CARTESIAN_POINT('Ctrl Pts',(-1.43622651411465,4.01195357487067,51.4970684100218));
#13437=CARTESIAN_POINT('Ctrl Pts',(-4.13860228786703,1.01521313918572,51.6933212925626));
#13438=CARTESIAN_POINT('Ctrl Pts',(-3.12976073044053,-2.89193666904667,
51.8895741751032));
#13439=CARTESIAN_POINT('Ctrl Pts',(0.685639547014467,-4.20577563258779,
52.0858270576438));
#13440=CARTESIAN_POINT('Ctrl Pts',(3.88620421837496,-1.74816794005548,52.2820799401845));
#13441=CARTESIAN_POINT('Ctrl Pts',(3.60188373594449,2.27708301682602,52.4783328227251));
#13442=CARTESIAN_POINT('Ctrl Pts',(0.087637203604645,4.26039759360026,52.6745857052657));
#13443=CARTESIAN_POINT('Ctrl Pts',(-3.50519640220714,2.42327658685007,52.8708385878064));
#13444=CARTESIAN_POINT('Ctrl Pts',(-3.95480674811289,-1.58687567121949,
53.067091470347));
#13445=CARTESIAN_POINT('Ctrl Pts',(-0.858013619596578,-4.17402477774934,
53.2633443528877));
#13446=CARTESIAN_POINT('Ctrl Pts',(3.00818814011577,-3.01819064426531,53.4595972354283));
#13447=CARTESIAN_POINT('Ctrl Pts',(4.17685004463815,0.844152986655114,53.655850117969));
#13448=CARTESIAN_POINT('Ctrl Pts',(1.59999506082199,3.94951722453104,53.8521030005096));
#13449=CARTESIAN_POINT('Ctrl Pts',(-2.4116273797703,3.51322130502469,54.0483558830502));
#13450=CARTESIAN_POINT('Ctrl Pts',(-4.2606653422332,-0.0734940982690915,
54.2446087655909));
#13451=CARTESIAN_POINT('Ctrl Pts',(-2.2890265223161,-3.59430495589765,54.4408616481315));
#13452=CARTESIAN_POINT('Ctrl Pts',(1.73525661133193,-3.89198600149939,54.6371145306722));
#13453=CARTESIAN_POINT('Ctrl Pts',(4.20347886863225,-0.699596984491061,
54.8333674132129));
#13454=CARTESIAN_POINT('Ctrl Pts',(2.90230530926582,3.12014333509764,55.0296202957534));
#13455=CARTESIAN_POINT('Ctrl Pts',(-1.00145954060489,4.14194994315114,55.2258731782941));
#13456=CARTESIAN_POINT('Ctrl Pts',(-4.00718314321467,1.44953571621855,55.4221260608347));
#13457=CARTESIAN_POINT('Ctrl Pts',(-3.41953567310348,-2.54272419293957,
55.6183789433754));
#13458=CARTESIAN_POINT('Ctrl Pts',(0.234520330591796,-4.25484086323758,
55.8146318259161));
#13459=CARTESIAN_POINT('Ctrl Pts',(3.67827434291722,-2.15150374384035,56.0108847084567));
#13460=CARTESIAN_POINT('Ctrl Pts',(3.82360047981264,1.88115654081442,56.2071375909973));
#13461=CARTESIAN_POINT('Ctrl Pts',(0.540180047856109,4.22692277754893,56.403390473538));
#13462=CARTESIAN_POINT('Ctrl Pts',(-3.22763730584292,2.78227023105407,56.5996433560786));
#13463=CARTESIAN_POINT('Ctrl Pts',(-4.10112770713532,-1.15733415252229,
56.7958962386193));
#13464=CARTESIAN_POINT('Ctrl Pts',(-1.29700371899468,-4.05911968132693,
56.9921491211599));
#13465=CARTESIAN_POINT('Ctrl Pts',(2.67018520888184,-3.32096053654349,57.1884020037006));
#13466=CARTESIAN_POINT('Ctrl Pts',(4.24293317826126,0.395210776154675,57.3846548862412));
#13467=CARTESIAN_POINT('Ctrl Pts',(2.01090395449088,3.75698544838359,57.5809077687819));
#13468=CARTESIAN_POINT('Ctrl Pts',(-2.02436522829424,3.74974608241314,57.7771606513224));
#13469=CARTESIAN_POINT('Ctrl Pts',(-4.24432610842296,0.379994490675165,
57.9734135338631));
#13470=CARTESIAN_POINT('Ctrl Pts',(-2.65825085865726,-3.33052383080523,
58.1696664164038));
#13471=CARTESIAN_POINT('Ctrl Pts',(1.31154165091137,-4.0544267886704,58.3659192989444));
#13472=CARTESIAN_POINT('Ctrl Pts',(4.10527711611601,-1.14264692916782,58.562172181485));
#13473=CARTESIAN_POINT('Ctrl Pts',(3.21758787539612,2.79388759650396,58.7584250640257));
#13474=CARTESIAN_POINT('Ctrl Pts',(-0.555237960034345,4.2248407334863,58.9546779465664));
#13475=CARTESIAN_POINT('Ctrl Pts',(-3.83052076119216,1.86766485748302,59.1509308291069));
#13476=CARTESIAN_POINT('Ctrl Pts',(-3.67013912963673,-2.16515038289994,
59.3471837116477));
#13477=CARTESIAN_POINT('Ctrl Pts',(-0.220046676040735,-4.25471956948896,
59.5434365941882));
#13478=CARTESIAN_POINT('Ctrl Pts',(3.43021234163902,-2.53232849629068,59.739689476729));
#13479=CARTESIAN_POINT('Ctrl Pts',(3.99886797969449,1.46880445609153,59.9359873460677));
#13480=CARTESIAN_POINT('Ctrl Pts',(1.99403924699144,3.2461190557392,60.066867587893));
#13481=CARTESIAN_POINT('Ctrl Pts',(0.835435555021673,3.5209619799037,60.1323302022048));
#13482=CARTESIAN_POINT('Ctrl Pts',(2.63010404172658,-2.12912255188162,49.595205300671));
#13483=CARTESIAN_POINT('Ctrl Pts',(3.33021246851552,-1.26427895642155,49.6606229281846));
#13484=CARTESIAN_POINT('Ctrl Pts',(3.79959166433701,1.19543272877191,49.7914581832116));
#13485=CARTESIAN_POINT('Ctrl Pts',(1.0950443232209,3.83366090105244,49.9877110657523));
#13486=CARTESIAN_POINT('Ctrl Pts',(-2.59172625709189,3.02565071629977,50.1839639482929));
#13487=CARTESIAN_POINT('Ctrl Pts',(-3.95423790127865,-0.491428448324842,
50.3802168308336));
#13488=CARTESIAN_POINT('Ctrl Pts',(-1.77094721912348,-3.56988785086517,
50.5764697133742));
#13489=CARTESIAN_POINT('Ctrl Pts',(2.00045516403601,-3.446081571636,50.7727225959148));
#13490=CARTESIAN_POINT('Ctrl Pts',(3.97796150854402,-0.23257895559744,50.9689754784555));
#13491=CARTESIAN_POINT('Ctrl Pts',(2.38831230212276,3.18974366914418,51.1652283609961));
#13492=CARTESIAN_POINT('Ctrl Pts',(-1.34301977665826,3.75158997632597,51.3614812435369));
#13493=CARTESIAN_POINT('Ctrl Pts',(-3.87001957261238,0.949328890707901,
51.5577341260774));
#13494=CARTESIAN_POINT('Ctrl Pts',(-2.92664876736462,-2.70425876503685,
51.7539870086181));
#13495=CARTESIAN_POINT('Ctrl Pts',(0.641143623411707,-3.93283357133589,
51.9502398911587));
#13496=CARTESIAN_POINT('Ctrl Pts',(3.6340013710356,-1.6347171517452,52.1464927736993));
#13497=CARTESIAN_POINT('Ctrl Pts',(3.36813242413865,2.12930724689704,52.34274565624));
#13498=CARTESIAN_POINT('Ctrl Pts',(0.0819498153357979,3.9839107330222,52.5389985387806));
#13499=CARTESIAN_POINT('Ctrl Pts',(-3.27771980462114,2.26601329836803,52.7352514213213));
#13500=CARTESIAN_POINT('Ctrl Pts',(-3.69815180501057,-1.48389226114473,
52.9315043038619));
#13501=CARTESIAN_POINT('Ctrl Pts',(-0.802331142362098,-3.90314325051617,
53.1277571864026));
#13502=CARTESIAN_POINT('Ctrl Pts',(2.81296586880989,-2.82231924082809,53.3240100689432));
#13503=CARTESIAN_POINT('Ctrl Pts',(3.90578516616716,0.789370022389415,53.5202629514839));
#13504=CARTESIAN_POINT('Ctrl Pts',(1.49616024221923,3.69320555543942,53.7165158340245));
#13505=CARTESIAN_POINT('Ctrl Pts',(-2.25512008943702,3.28522391562577,53.9127687165651));
#13506=CARTESIAN_POINT('Ctrl Pts',(-3.98416110558228,-0.0687245545692351,
54.1090215991058));
#13507=CARTESIAN_POINT('Ctrl Pts',(-2.14047565516563,-3.36104548389223,
54.3052744816464));
#13508=CARTESIAN_POINT('Ctrl Pts',(1.62264372903072,-3.63940793400053,54.5015273641871));
#13509=CARTESIAN_POINT('Ctrl Pts',(3.93068586038341,-0.65419526559929,54.6977802467277));
#13510=CARTESIAN_POINT('Ctrl Pts',(2.71395451200611,2.91765551176149,54.8940331292684));
#13511=CARTESIAN_POINT('Ctrl Pts',(-0.936467858891026,3.87314997523886,
55.090286011809));
#13512=CARTESIAN_POINT('Ctrl Pts',(-3.7471291311917,1.35546525197946,55.2865388943497));
#13513=CARTESIAN_POINT('Ctrl Pts',(-3.19761819659582,-2.37770911770861,
55.4827917768903));
#13514=CARTESIAN_POINT('Ctrl Pts',(0.219300673617886,-3.9787146175785,55.6790446594309));
#13515=CARTESIAN_POINT('Ctrl Pts',(3.43956551279636,-2.01187768721363,55.8752975419716));
#13516=CARTESIAN_POINT('Ctrl Pts',(3.5754604249135,1.75907519633921,56.0715504245122));
#13517=CARTESIAN_POINT('Ctrl Pts',(0.505124003837354,3.95260833083485,56.2678033070529));
#13518=CARTESIAN_POINT('Ctrl Pts',(-3.01817345037608,2.60170934569926,56.4640561895935));
#13519=CARTESIAN_POINT('Ctrl Pts',(-3.83497697832098,-1.08222668204786,
56.6603090721341));
#13520=CARTESIAN_POINT('Ctrl Pts',(-1.21283211797753,-3.7956951457656,56.8565619546748));
#13521=CARTESIAN_POINT('Ctrl Pts',(2.49689830094754,-3.10544028692363,57.0528148372155));
#13522=CARTESIAN_POINT('Ctrl Pts',(3.96757970518115,0.369562797447294,57.2490677197561));
#13523=CARTESIAN_POINT('Ctrl Pts',(1.88040239704553,3.51316850664524,57.4453206022968));
#13524=CARTESIAN_POINT('Ctrl Pts',(-1.89299007507492,3.5063989535328,57.6415734848374));
#13525=CARTESIAN_POINT('Ctrl Pts',(-3.96888223840713,0.355334002667765,
57.837826367378));
#13526=CARTESIAN_POINT('Ctrl Pts',(-2.48573845379553,-3.11438295244143,
58.0340792499187));
#13527=CARTESIAN_POINT('Ctrl Pts',(1.22642658227961,-3.79130680758531,58.2303321324593));
#13528=CARTESIAN_POINT('Ctrl Pts',(3.83885710326488,-1.06849261486876,58.4265850149999));
#13529=CARTESIAN_POINT('Ctrl Pts',(3.00877619743473,2.61257277942545,58.6228378975406));
#13530=CARTESIAN_POINT('Ctrl Pts',(-0.519204703261722,3.95066140510655,
58.8190907800813));
#13531=CARTESIAN_POINT('Ctrl Pts',(-3.58193160105556,1.74645908226778,59.0153436626219));
#13532=CARTESIAN_POINT('Ctrl Pts',(-3.4319582501427,-2.02463870085725,59.2115965451625));
#13533=CARTESIAN_POINT('Ctrl Pts',(-0.205766315275689,-3.97860119542568,
59.4078494277032));
#13534=CARTESIAN_POINT('Ctrl Pts',(3.20760198177951,-2.36798807018971,59.6041023102438));
#13535=CARTESIAN_POINT('Ctrl Pts',(3.73935359652219,1.37348350917383,59.8004001795827));
#13536=CARTESIAN_POINT('Ctrl Pts',(1.8646321578272,3.03545579085233,59.931280421408));
#13537=CARTESIAN_POINT('Ctrl Pts',(0.781218325585102,3.29246224422161,59.9967430357197));
#13538=CARTESIAN_POINT('Ctrl Pts',(0.784811935329597,3.29764693208115,60.));
#13539=CARTESIAN_POINT('Ctrl Pts',(0.889235603863764,3.28374633008718,60.));
#13540=CARTESIAN_POINT('Ctrl Pts',(0.992623261153783,3.26463846910174,60.));
#13541=CARTESIAN_POINT('Ctrl Pts',(1.09473595312137,3.24065669353082,60.));
#13542=CARTESIAN_POINT('Ctrl Pts',(1.20064317507693,3.2157837499296,60.));
#13543=CARTESIAN_POINT('Ctrl Pts',(1.3051794749988,3.18566793874592,60.));
#13544=CARTESIAN_POINT('Ctrl Pts',(1.40808566984841,3.15062538127982,60.));
#13545=CARTESIAN_POINT('Ctrl Pts',(1.51283637750168,3.11495471346514,60.));
#13546=CARTESIAN_POINT('Ctrl Pts',(1.61589871569635,3.07417889385732,60.));
#13547=CARTESIAN_POINT('Ctrl Pts',(1.71699714510354,3.02857636387343,60.));
#13548=CARTESIAN_POINT('Ctrl Pts',(1.78322715166281,2.99870195457091,60.));
#13549=CARTESIAN_POINT('Ctrl Pts',(1.84861426059305,2.9667549850191,60.));
#13550=CARTESIAN_POINT('Ctrl Pts',(1.91307826822121,2.93280201322383,60.));
#13551=CARTESIAN_POINT('Ctrl Pts',(1.94433236805735,2.91634058599851,60.));
#13552=CARTESIAN_POINT('Ctrl Pts',(1.97536889450896,2.89940780269719,60.));
#13553=CARTESIAN_POINT('Ctrl Pts',(2.00618011160133,2.88200955967882,60.));
#13554=CARTESIAN_POINT('Ctrl Pts',(2.03056702399939,2.86823894402617,60.));
#13555=CARTESIAN_POINT('Ctrl Pts',(2.05481756915562,2.85417358949421,60.));
#13556=CARTESIAN_POINT('Ctrl Pts',(2.07888625271118,2.83984169026282,60.));
#13557=CARTESIAN_POINT('Ctrl Pts',(2.17718404178886,2.78130944837773,60.));
#13558=CARTESIAN_POINT('Ctrl Pts',(2.2725670919976,2.71827226665768,60.));
#13559=CARTESIAN_POINT('Ctrl Pts',(2.36475625773662,2.65106472009617,60.));
#13560=CARTESIAN_POINT('Ctrl Pts',(2.45801085040187,2.58308045829727,60.));
#13561=CARTESIAN_POINT('Ctrl Pts',(2.54799808861466,2.51082853560115,60.));
#13562=CARTESIAN_POINT('Ctrl Pts',(2.63441837229004,2.43460216440961,60.));
#13563=CARTESIAN_POINT('Ctrl Pts',(2.72073546283663,2.35846681395307,60.));
#13564=CARTESIAN_POINT('Ctrl Pts',(2.80349489384814,2.27836603613578,60.));
#13565=CARTESIAN_POINT('Ctrl Pts',(2.88237584537992,2.19454559636136,60.));
#13566=CARTESIAN_POINT('Ctrl Pts',(2.95189189665301,2.12067648251395,60.));
#13567=CARTESIAN_POINT('Ctrl Pts',(3.01839575888545,2.04391761646293,60.));
#13568=CARTESIAN_POINT('Ctrl Pts',(3.08164607665535,1.96441162407651,60.));
#13569=CARTESIAN_POINT('Ctrl Pts',(3.09160214974873,1.95189678621529,60.));
#13570=CARTESIAN_POINT('Ctrl Pts',(3.10147565654979,1.93931615773848,60.));
#13571=CARTESIAN_POINT('Ctrl Pts',(3.11125942805904,1.92667863680468,60.));
#13572=CARTESIAN_POINT('Ctrl Pts',(3.18384639438312,1.83291936354545,60.));
#13573=CARTESIAN_POINT('Ctrl Pts',(3.25159841668943,1.73590401314964,60.));
#13574=CARTESIAN_POINT('Ctrl Pts',(3.31421073674484,1.63593934473944,60.));
#13575=CARTESIAN_POINT('Ctrl Pts',(3.37660547873583,1.53632205395468,60.));
#13576=CARTESIAN_POINT('Ctrl Pts',(3.43389695780907,1.4337753814893,60.));
#13577=CARTESIAN_POINT('Ctrl Pts',(3.48575479573506,1.32856043853129,60.));
#13578=CARTESIAN_POINT('Ctrl Pts',(3.4931113037334,1.31363473780076,60.));
#13579=CARTESIAN_POINT('Ctrl Pts',(3.50035840622805,1.2986552783797,60.));
#13580=CARTESIAN_POINT('Ctrl Pts',(3.50749509871695,1.28362274566985,60.));
#13581=CARTESIAN_POINT('Ctrl Pts',(3.55683940162616,1.17968526361056,60.));
#13582=CARTESIAN_POINT('Ctrl Pts',(3.60090919697516,1.07321295524336,60.));
#13583=CARTESIAN_POINT('Ctrl Pts',(3.63979310801694,0.964595844985372,60.));
#13584=CARTESIAN_POINT('Ctrl Pts',(3.66420924373342,0.896392569282407,60.));
#13585=CARTESIAN_POINT('Ctrl Pts',(3.68657974486052,0.827342990746825,60.));
#13586=CARTESIAN_POINT('Ctrl Pts',(3.7069172792925,0.757538875098194,60.));
#13587=CARTESIAN_POINT('Ctrl Pts',(3.71289219481231,0.737031291185787,60.));
#13588=CARTESIAN_POINT('Ctrl Pts',(3.71869159509938,0.716458563232633,60.));
#13589=CARTESIAN_POINT('Ctrl Pts',(3.72431568230938,0.695822974884761,60.));
#13590=CARTESIAN_POINT('Ctrl Pts',(3.72862390834875,0.680015471242239,60.));
#13591=CARTESIAN_POINT('Ctrl Pts',(3.73282894190367,0.664172025657236,60.));
#13592=CARTESIAN_POINT('Ctrl Pts',(3.73692780152788,0.648306312974997,60.));
#13593=CARTESIAN_POINT('Ctrl Pts',(3.76710608338592,0.531493347150171,60.));
#13594=CARTESIAN_POINT('Ctrl Pts',(3.79158238148832,0.41329696895828,60.));
#13595=CARTESIAN_POINT('Ctrl Pts',(3.8105094559077,0.294179008852515,60.));
#13596=CARTESIAN_POINT('Ctrl Pts',(3.82934522625211,0.175635672955355,60.));
#13597=CARTESIAN_POINT('Ctrl Pts',(3.84268518208166,0.0561787816862602,
60.));
#13598=CARTESIAN_POINT('Ctrl Pts',(3.85063242918259,-0.063766621316311,
60.));
#13599=CARTESIAN_POINT('Ctrl Pts',(3.858704791944,-0.18560035723804,60.));
#13600=CARTESIAN_POINT('Ctrl Pts',(3.86121348940923,-0.30793892891327,60.));
#13601=CARTESIAN_POINT('Ctrl Pts',(3.85821592230841,-0.43035561873873,60.));
#13602=CARTESIAN_POINT('Ctrl Pts',(3.85526835997703,-0.550730179682494,
60.));
#13603=CARTESIAN_POINT('Ctrl Pts',(3.84699662600882,-0.671181149539089,
60.));
#13604=CARTESIAN_POINT('Ctrl Pts',(3.83340642503076,-0.791307982107533,
60.));
#13605=CARTESIAN_POINT('Ctrl Pts',(3.83135847340105,-0.809410285592786,
60.));
#13606=CARTESIAN_POINT('Ctrl Pts',(3.82918993653534,-0.827502340964368,
60.));
#13607=CARTESIAN_POINT('Ctrl Pts',(3.82690230603326,-0.845572403651534,
60.));
#13608=CARTESIAN_POINT('Ctrl Pts',(3.81116757337382,-0.969861533939128,
60.));
#13609=CARTESIAN_POINT('Ctrl Pts',(3.78978713160578,-1.0932500409073,60.));
#13610=CARTESIAN_POINT('Ctrl Pts',(3.76284273210423,-1.21528813763156,60.));
#13611=CARTESIAN_POINT('Ctrl Pts',(3.73586199351469,-1.33749082340648,60.));
#13612=CARTESIAN_POINT('Ctrl Pts',(3.70330231983611,-1.45834038572235,60.));
#13613=CARTESIAN_POINT('Ctrl Pts',(3.665194221274,-1.57738923136754,60.));
#13614=CARTESIAN_POINT('Ctrl Pts',(3.65552125866432,-1.60760734972301,60.));
#13615=CARTESIAN_POINT('Ctrl Pts',(3.64549055351521,-1.6377094291362,60.));
#13616=CARTESIAN_POINT('Ctrl Pts',(3.6351020718132,-1.66768807850306,60.));
#13617=CARTESIAN_POINT('Ctrl Pts',(3.62847368432654,-1.68681600402967,60.));
#13618=CARTESIAN_POINT('Ctrl Pts',(3.62169927309294,-1.70589468101949,60.));
#13619=CARTESIAN_POINT('Ctrl Pts',(3.61477991705996,-1.72491906517069,60.));
#13620=CARTESIAN_POINT('Ctrl Pts',(3.57054791692283,-1.84653248676284,60.));
#13621=CARTESIAN_POINT('Ctrl Pts',(3.52049512035426,-1.96566066503241,60.));
#13622=CARTESIAN_POINT('Ctrl Pts',(3.46468375047193,-2.0818202580808,60.));
#13623=CARTESIAN_POINT('Ctrl Pts',(3.4088723805896,-2.19797985112919,60.));
#13624=CARTESIAN_POINT('Ctrl Pts',(3.34730245526163,-2.31117192238551,60.));
#13625=CARTESIAN_POINT('Ctrl Pts',(3.27997999600525,-2.42090362774469,60.));
#13626=CARTESIAN_POINT('Ctrl Pts',(3.24835722849275,-2.47244690536188,60.));
#13627=CARTESIAN_POINT('Ctrl Pts',(3.21546442815301,-2.52322646076057,60.));
#13628=CARTESIAN_POINT('Ctrl Pts',(3.18134623828594,-2.57322545645539,59.9999999999999));
#13629=CARTESIAN_POINT('Origin',(0.,0.,60.));
#13630=CARTESIAN_POINT('',(8.,9.79717439317883E-16,58.5));
#13631=CARTESIAN_POINT('Origin',(0.,0.,58.5));
#13632=CARTESIAN_POINT('',(8.,9.79717439317883E-16,60.));
#13633=CARTESIAN_POINT('',(8.,-9.79717439317883E-16,60.));
#13634=CARTESIAN_POINT('Origin',(0.,0.,60.));
#13635=CARTESIAN_POINT('Origin',(0.,0.,58.5));
#13636=CARTESIAN_POINT('',(-5.,-6.12323399573677E-16,58.5));
#13637=CARTESIAN_POINT('Origin',(0.,0.,58.5));
#13638=CARTESIAN_POINT('Origin',(0.,0.,28.));
#13639=CARTESIAN_POINT('',(-5.,-6.12323399573677E-16,28.));
#13640=CARTESIAN_POINT('Origin',(0.,0.,28.));
#13641=CARTESIAN_POINT('Origin',(0.,0.,0.));
#13642=CARTESIAN_POINT('',(-5.,-6.12323399573677E-16,0.));
#13643=CARTESIAN_POINT('Origin',(0.,0.,60.));
#34388=UNCERTAINTY_MEASURE_WITH_UNIT(LENGTH_MEASURE(0.01),#34404,
'DISTANCE_ACCURACY_VALUE',
'Maximum model space distance between geometric entities at asserted c
onnectivities');
#34393=UNCERTAINTY_MEASURE_WITH_UNIT(LENGTH_MEASURE(0.01),#34404,
'DISTANCE_ACCURACY_VALUE',
'Maximum model space distance between geometric entities at asserted c
onnectivities');
#34398=(
GEOMETRIC_REPRESENTATION_CONTEXT(3)
GLOBAL_UNCERTAINTY_ASSIGNED_CONTEXT((#34388))
GLOBAL_UNIT_ASSIGNED_CONTEXT((#34404,#34406,#34407))
REPRESENTATION_CONTEXT('','3D')
);
#34403=(
GEOMETRIC_REPRESENTATION_CONTEXT(3)
GLOBAL_UNCERTAINTY_ASSIGNED_CONTEXT((#34393))
GLOBAL_UNIT_ASSIGNED_CONTEXT((#34404,#34406,#34407))
REPRESENTATION_CONTEXT('','3D')
);
#34404=(
LENGTH_UNIT()
NAMED_UNIT(*)
SI_UNIT(.MILLI.,.METRE.)
);
#34406=(
NAMED_UNIT(*)
PLANE_ANGLE_UNIT()
SI_UNIT($,.RADIAN.)
);
#34407=(
NAMED_UNIT(*)
SI_UNIT($,.STERADIAN.)
SOLID_ANGLE_UNIT()
);
#34412=SHAPE_DEFINITION_REPRESENTATION(#34421,#34438);
#34421=PRODUCT_DEFINITION_SHAPE('',$,#34448);
#34438=SHAPE_REPRESENTATION('',(#4522),#34398);
#34443=PRODUCT_DEFINITION_CONTEXT('part definition',#34472,'design');
#34448=PRODUCT_DEFINITION('Extended_Neck','Extended_Neck',#34457,#34443);
#34457=PRODUCT_DEFINITION_FORMATION('',$,#34478);
#34472=APPLICATION_CONTEXT(
'Core Data for Automotive Mechanical Design Process');
#34473=PRODUCT_CONTEXT('part definition',#34472,'mechanical');
#34478=PRODUCT('Extended_Neck','Extended_Neck',$,(#34473));
#34484=PRESENTATION_STYLE_ASSIGNMENT((#34486));
#34486=SURFACE_STYLE_USAGE(.BOTH.,#34488);
#34488=SURFACE_SIDE_STYLE('',(#34490));
#34490=SURFACE_STYLE_FILL_AREA(#34492);
#34492=FILL_AREA_STYLE('Opaque(160,160,160)',(#34494));
#34494=FILL_AREA_STYLE_COLOUR('Opaque(160,160,160)',#34496);
#34496=COLOUR_RGB('Opaque(160,160,160)', 0.09019608, 0.27058824, 0.51372549);
ENDSEC;
END-ISO-10303-21;
